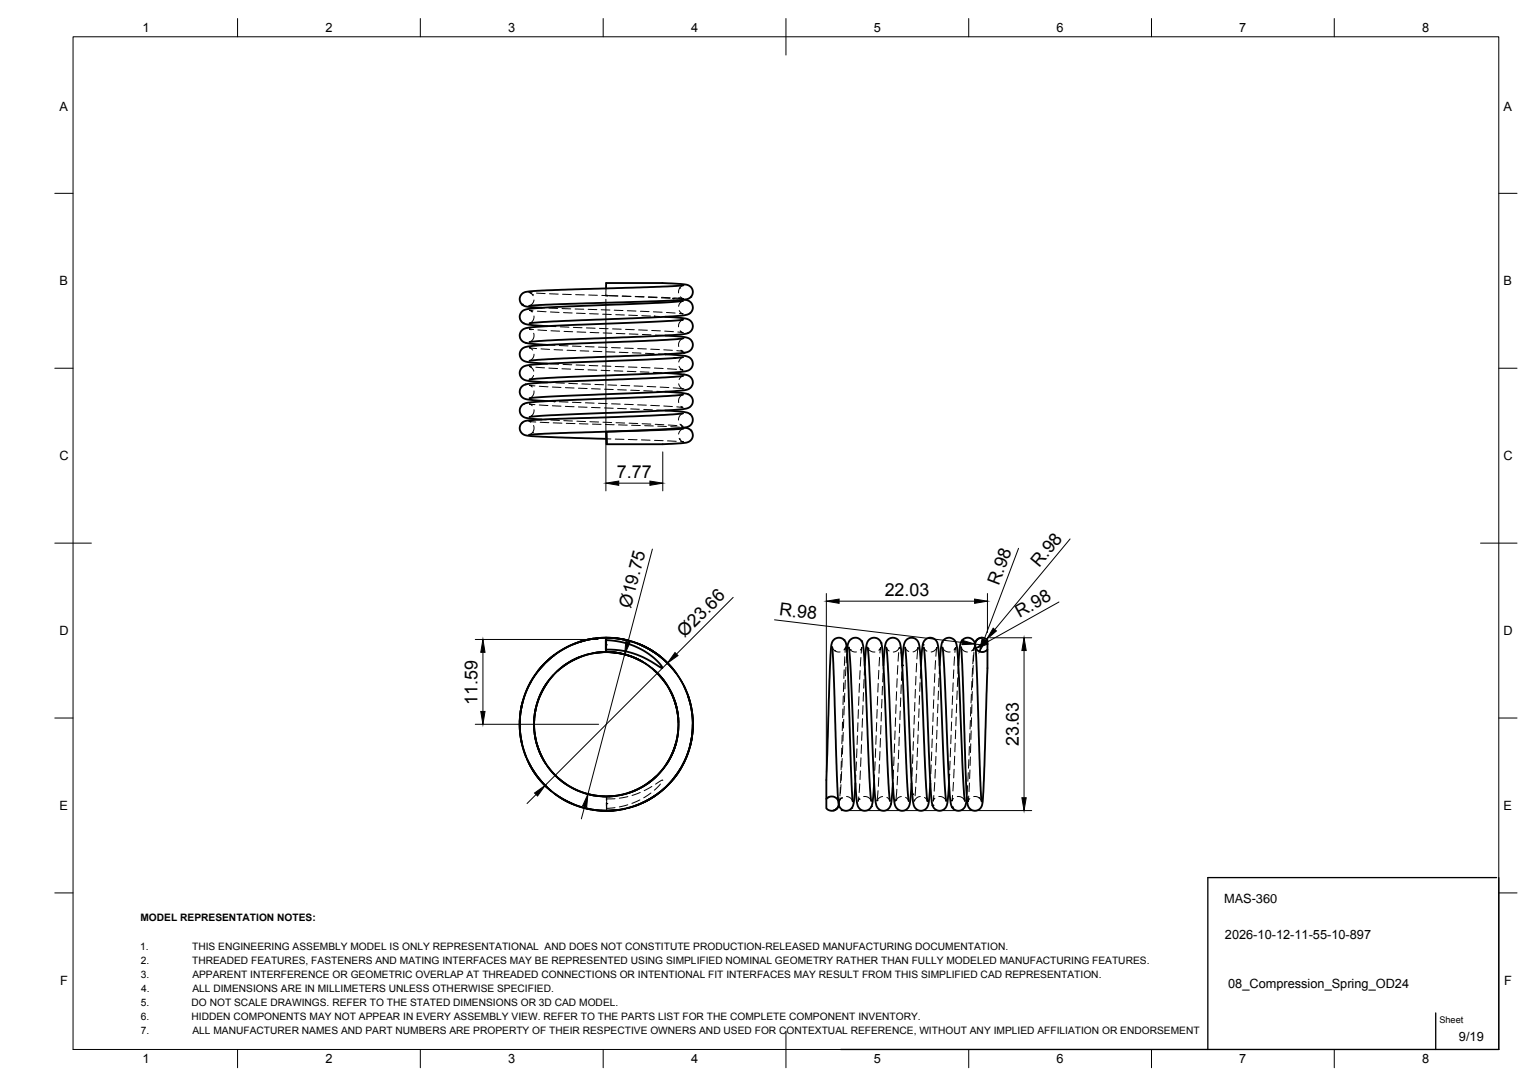
ISO-10303-21;
HEADER;
/* Generated by software containing ST-Developer
 * from STEP Tools, Inc. (www.steptools.com) 
 */

FILE_DESCRIPTION(
/* description */ (''),
/* implementation_level */ '2;1');

FILE_NAME(
/* name */ '08_Compression_Spring_OD24.step',
/* time_stamp */ '2026-11-04T18:53:29-08:00',
/* author */ (''),
/* organization */ (''),
/* preprocessor_version */ 'ST-DEVELOPER v20.2',
/* originating_system */ 'Autodesk Translation Framework v15.17.0.0',
/* authorisation */ '');

FILE_SCHEMA (('AUTOMOTIVE_DESIGN { 1 0 10303 214 3 1 1 }'));
ENDSEC;

DATA;
#10=MECHANICAL_DESIGN_GEOMETRIC_PRESENTATION_REPRESENTATION('',(#1334),#100031);
#1298=SHAPE_REPRESENTATION_RELATIONSHIP('SRR','None',#100108,#1316);
#1316=ADVANCED_BREP_SHAPE_REPRESENTATION('',(#1352),#100020);
#1334=STYLED_ITEM('',(#100203),#1352);
#1352=MANIFOLD_SOLID_BREP('Body1',#20124);
#1634=PLANE('',#22153);
#1635=PLANE('',#22154);
#1636=PLANE('',#22155);
#1637=PLANE('',#22156);
#1774=FACE_BOUND('',#7247,.T.);
#1775=FACE_BOUND('',#7248,.T.);
#3151=LINE('',#93226,#4438);
#3152=LINE('',#93320,#4439);
#4438=VECTOR('',#27336,10.);
#4439=VECTOR('',#27341,10.);
#6005=FACE_OUTER_BOUND('',#7242,.T.);
#6006=FACE_OUTER_BOUND('',#7243,.T.);
#6007=FACE_OUTER_BOUND('',#7244,.T.);
#6008=FACE_OUTER_BOUND('',#7245,.T.);
#6009=FACE_OUTER_BOUND('',#7246,.T.);
#6010=FACE_OUTER_BOUND('',#7249,.T.);
#7242=EDGE_LOOP('',(#18137,#18138));
#7243=EDGE_LOOP('',(#18139,#18140,#18141,#18142,#18143,#18144,#18145));
#7244=EDGE_LOOP('',(#18146,#18147));
#7245=EDGE_LOOP('',(#18148,#18149,#18150,#18151,#18152,#18153,#18154));
#7246=EDGE_LOOP('',(#18155,#18156,#18157,#18158,#18159,#18160,#18161,#18162));
#7247=EDGE_LOOP('',(#18163,#18164));
#7248=EDGE_LOOP('',(#18165,#18166));
#7249=EDGE_LOOP('',(#18167,#18168,#18169,#18170,#18171,#18172,#18173,#18174,
#18175,#18176));
#7985=B_SPLINE_CURVE_WITH_KNOTS('',3,(#93194,#93195,#93196,#93197,#93198,
#93199,#93200,#93201,#93202,#93203,#93204,#93205,#93206,#93207,#93208,#93209,
#93210,#93211,#93212,#93213,#93214,#93215,#93216,#93217,#93218,#93219,#93220,
#93221,#93222,#93223,#93224,#93225),.UNSPECIFIED.,.F.,.F.,(4,2,2,2,2,2,
2,2,2,2,2,2,2,2,2,4),(3.54152458065573E-10,0.288711445101139,0.523258332244725,
0.921227317049852,1.09267154481917,1.12602826877806,1.13805490776081,1.14561247672485,
1.15218349843735,1.15992334586198,1.17330081210199,1.20544465265463,1.30433060811633,
1.73541082798229,2.00533365271455,2.34908372554942),.UNSPECIFIED.);
#7986=B_SPLINE_CURVE_WITH_KNOTS('',3,(#93229,#93230,#93231,#93232,#93233,
#93234,#93235,#93236,#93237,#93238),.UNSPECIFIED.,.F.,.F.,(4,2,2,2,4),(-0.235035705616533,
-0.164045621201278,-0.0870897131881243,-0.0381417578315876,0.),
 .UNSPECIFIED.);
#7987=B_SPLINE_CURVE_WITH_KNOTS('',3,(#93240,#93241,#93242,#93243,#93244,
#93245,#93246,#93247,#93248,#93249),.UNSPECIFIED.,.F.,.F.,(4,2,2,2,4),(-0.0803122862957921,
-0.0602646333915054,-0.0402202940526313,-0.0201483463522527,-3.56243524540593E-5),
 .UNSPECIFIED.);
#7988=B_SPLINE_CURVE_WITH_KNOTS('',3,(#93251,#93252,#93253,#93254,#93255,
#93256),.UNSPECIFIED.,.F.,.F.,(4,2,4),(8.43662143615864E-5,0.00327116298064693,
0.00646179051431274),.UNSPECIFIED.);
#7989=B_SPLINE_CURVE_WITH_KNOTS('',3,(#93258,#93259,#93260,#93261,#93262,
#93263,#93264,#93265,#93266,#93267),.UNSPECIFIED.,.F.,.F.,(4,2,2,2,4),(-0.106351401183245,
-0.0798864576605021,-0.0531877160318232,-0.0265812067152108,-7.06104949174502E-6),
 .UNSPECIFIED.);
#7990=B_SPLINE_CURVE_WITH_KNOTS('',3,(#93269,#93270,#93271,#93272,#93273,
#93274,#93275,#93276,#93277,#93278),.UNSPECIFIED.,.F.,.F.,(4,2,2,2,4),(-0.0971883190541716,
-0.0727561460747867,-0.048468056376207,-0.0242270507757942,0.),
 .UNSPECIFIED.);
#7991=B_SPLINE_CURVE_WITH_KNOTS('',3,(#93279,#93280,#93281,#93282,#93283,
#93284),.UNSPECIFIED.,.F.,.F.,(4,2,4),(-0.0301723368590298,-0.0150922159606526,
-2.55953913249195E-6),.UNSPECIFIED.);
#7992=B_SPLINE_CURVE_WITH_KNOTS('',3,(#93288,#93289,#93290,#93291,#93292,
#93293,#93294,#93295,#93296,#93297,#93298,#93299,#93300,#93301,#93302,#93303,
#93304,#93305,#93306,#93307,#93308,#93309,#93310,#93311,#93312,#93313,#93314,
#93315,#93316,#93317,#93318,#93319),.UNSPECIFIED.,.F.,.F.,(4,2,2,2,2,2,
2,2,2,2,2,2,2,2,2,4),(-2.01212438752124,-1.76578196828659,-1.5647664663706,
-1.20118246901991,-1.06053517315717,-1.02977885200715,-1.0193276272259,
-1.01279623524482,-1.00715009449403,-1.00055979488344,-0.989257775261865,
-0.96242213266161,-0.881471927659453,-0.518895860123459,-0.290806811506921,
-8.2501916409683E-10),.UNSPECIFIED.);
#7993=B_SPLINE_CURVE_WITH_KNOTS('',3,(#93323,#93324,#93325,#93326,#93327,
#93328,#93329,#93330,#93331,#93332),.UNSPECIFIED.,.F.,.F.,(4,2,2,2,4),(-0.189468447311924,
-0.155678960910493,-0.111541963335214,-0.0470106922386932,-7.10058815808075E-6),
 .UNSPECIFIED.);
#7994=B_SPLINE_CURVE_WITH_KNOTS('',3,(#93334,#93335,#93336,#93337,#93338,
#93339,#93340,#93341,#93342,#93343),.UNSPECIFIED.,.F.,.F.,(4,2,2,2,4),(-0.0812741980146226,
-0.061010630542918,-0.0406258560977219,-0.0203042042142377,0.),
 .UNSPECIFIED.);
#7995=B_SPLINE_CURVE_WITH_KNOTS('',3,(#93345,#93346,#93347,#93348,#93349,
#93350),.UNSPECIFIED.,.F.,.F.,(4,2,4),(-0.0064959341341575,-0.00329347810601311,
-8.81436577924804E-5),.UNSPECIFIED.);
#7996=B_SPLINE_CURVE_WITH_KNOTS('',3,(#93352,#93353,#93354,#93355,#93356,
#93357),.UNSPECIFIED.,.F.,.F.,(4,2,4),(-0.00936112110047215,-0.00472017132367055,
-6.30707363171211E-5),.UNSPECIFIED.);
#7997=B_SPLINE_CURVE_WITH_KNOTS('',3,(#93359,#93360,#93361,#93362,#93363,
#93364,#93365,#93366,#93367,#93368,#93369,#93370,#93371,#93372,#93373,#93374),
 .UNSPECIFIED.,.F.,.F.,(4,2,2,2,2,2,2,4),(-0.201490383661384,-0.178130230033713,
-0.154775766161226,-0.145700922114215,-0.102563961887103,-0.0587557032775208,
-0.029368346867021,-7.06104927835685E-6),.UNSPECIFIED.);
#7998=B_SPLINE_CURVE_WITH_KNOTS('',3,(#93375,#93376,#93377,#93378,#93379,
#93380),.UNSPECIFIED.,.F.,.F.,(4,2,4),(-0.0308102197342027,-0.0154008404140284,
0.),.UNSPECIFIED.);
#7999=B_SPLINE_CURVE_WITH_KNOTS('',3,(#94481,#94482,#94483,#94484,#94485,
#94486,#94487,#94488,#94489,#94490,#94491,#94492,#94493,#94494,#94495,#94496,
#94497,#94498,#94499,#94500,#94501,#94502,#94503,#94504,#94505,#94506,#94507,
#94508,#94509,#94510,#94511,#94512,#94513,#94514,#94515,#94516,#94517,#94518,
#94519,#94520,#94521,#94522,#94523,#94524,#94525,#94526,#94527,#94528,#94529,
#94530,#94531,#94532,#94533,#94534,#94535,#94536,#94537,#94538,#94539,#94540,
#94541,#94542,#94543,#94544,#94545,#94546,#94547,#94548,#94549,#94550,#94551,
#94552,#94553,#94554,#94555,#94556,#94557,#94558,#94559,#94560,#94561,#94562,
#94563,#94564,#94565,#94566,#94567,#94568,#94569,#94570,#94571,#94572,#94573,
#94574,#94575,#94576,#94577,#94578,#94579,#94580,#94581,#94582,#94583,#94584,
#94585,#94586,#94587,#94588,#94589,#94590,#94591,#94592,#94593,#94594,#94595,
#94596,#94597,#94598,#94599,#94600,#94601,#94602,#94603,#94604,#94605,#94606,
#94607,#94608,#94609,#94610,#94611,#94612,#94613,#94614,#94615,#94616,#94617,
#94618,#94619,#94620,#94621,#94622,#94623,#94624,#94625,#94626,#94627,#94628,
#94629,#94630,#94631,#94632,#94633,#94634,#94635,#94636,#94637,#94638,#94639,
#94640,#94641,#94642,#94643,#94644,#94645,#94646,#94647,#94648,#94649,#94650,
#94651,#94652,#94653,#94654,#94655,#94656,#94657,#94658,#94659,#94660,#94661,
#94662,#94663,#94664,#94665,#94666,#94667,#94668,#94669,#94670,#94671,#94672,
#94673,#94674,#94675,#94676,#94677,#94678,#94679,#94680,#94681,#94682,#94683,
#94684,#94685,#94686,#94687,#94688,#94689,#94690,#94691,#94692,#94693,#94694,
#94695,#94696,#94697,#94698,#94699,#94700,#94701,#94702,#94703,#94704,#94705,
#94706,#94707,#94708,#94709,#94710,#94711,#94712,#94713,#94714,#94715,#94716,
#94717,#94718,#94719,#94720,#94721,#94722,#94723,#94724,#94725,#94726,#94727,
#94728,#94729,#94730,#94731,#94732,#94733,#94734,#94735,#94736,#94737,#94738,
#94739,#94740,#94741,#94742,#94743,#94744,#94745,#94746,#94747,#94748,#94749,
#94750,#94751,#94752,#94753,#94754,#94755,#94756,#94757,#94758,#94759,#94760,
#94761,#94762,#94763,#94764,#94765,#94766,#94767,#94768,#94769,#94770,#94771,
#94772,#94773,#94774,#94775,#94776,#94777,#94778,#94779,#94780,#94781,#94782,
#94783,#94784,#94785,#94786,#94787,#94788,#94789,#94790,#94791,#94792,#94793,
#94794,#94795,#94796,#94797,#94798,#94799,#94800,#94801,#94802,#94803,#94804,
#94805,#94806,#94807,#94808,#94809,#94810,#94811,#94812,#94813,#94814,#94815,
#94816,#94817,#94818,#94819,#94820,#94821,#94822,#94823,#94824,#94825,#94826,
#94827,#94828,#94829,#94830,#94831,#94832,#94833,#94834,#94835,#94836,#94837,
#94838,#94839,#94840,#94841,#94842,#94843,#94844,#94845,#94846,#94847,#94848,
#94849,#94850,#94851,#94852,#94853,#94854,#94855,#94856,#94857,#94858,#94859,
#94860,#94861,#94862,#94863,#94864,#94865,#94866,#94867,#94868,#94869,#94870,
#94871,#94872,#94873,#94874,#94875,#94876,#94877,#94878,#94879,#94880,#94881,
#94882,#94883,#94884,#94885,#94886,#94887,#94888,#94889,#94890,#94891,#94892,
#94893,#94894,#94895,#94896,#94897,#94898,#94899,#94900,#94901,#94902,#94903,
#94904,#94905,#94906,#94907,#94908,#94909,#94910,#94911,#94912,#94913,#94914,
#94915,#94916,#94917,#94918,#94919,#94920,#94921,#94922,#94923,#94924,#94925,
#94926,#94927,#94928,#94929,#94930,#94931,#94932,#94933,#94934,#94935,#94936,
#94937,#94938,#94939,#94940,#94941,#94942,#94943,#94944,#94945,#94946,#94947,
#94948,#94949,#94950,#94951,#94952,#94953,#94954,#94955,#94956,#94957,#94958,
#94959,#94960,#94961,#94962,#94963,#94964,#94965,#94966,#94967,#94968,#94969,
#94970,#94971,#94972,#94973,#94974,#94975,#94976,#94977,#94978,#94979,#94980,
#94981,#94982,#94983,#94984,#94985,#94986,#94987,#94988,#94989,#94990,#94991,
#94992,#94993,#94994,#94995,#94996,#94997,#94998,#94999,#95000,#95001,#95002,
#95003,#95004,#95005,#95006,#95007,#95008,#95009,#95010,#95011,#95012,#95013,
#95014,#95015,#95016,#95017,#95018,#95019,#95020,#95021,#95022,#95023,#95024,
#95025,#95026,#95027,#95028,#95029,#95030,#95031,#95032,#95033,#95034,#95035,
#95036,#95037,#95038,#95039,#95040,#95041,#95042,#95043,#95044,#95045,#95046,
#95047,#95048,#95049,#95050,#95051,#95052,#95053,#95054,#95055,#95056,#95057,
#95058,#95059,#95060,#95061,#95062,#95063,#95064,#95065,#95066,#95067,#95068,
#95069,#95070,#95071,#95072,#95073,#95074,#95075,#95076,#95077,#95078,#95079,
#95080,#95081,#95082,#95083,#95084,#95085,#95086,#95087,#95088,#95089,#95090,
#95091,#95092,#95093,#95094,#95095,#95096,#95097,#95098,#95099,#95100,#95101,
#95102,#95103,#95104,#95105,#95106,#95107,#95108,#95109,#95110,#95111,#95112,
#95113,#95114,#95115,#95116,#95117,#95118,#95119,#95120,#95121,#95122,#95123,
#95124,#95125,#95126,#95127,#95128,#95129,#95130,#95131,#95132,#95133,#95134,
#95135,#95136,#95137,#95138,#95139,#95140,#95141,#95142,#95143,#95144,#95145,
#95146,#95147,#95148,#95149,#95150,#95151,#95152,#95153,#95154,#95155,#95156,
#95157,#95158,#95159,#95160,#95161,#95162,#95163,#95164,#95165,#95166,#95167,
#95168,#95169,#95170,#95171,#95172,#95173,#95174,#95175,#95176,#95177,#95178,
#95179,#95180,#95181,#95182,#95183,#95184,#95185,#95186,#95187,#95188,#95189,
#95190,#95191,#95192,#95193,#95194,#95195,#95196,#95197,#95198,#95199,#95200,
#95201,#95202,#95203,#95204,#95205,#95206,#95207,#95208,#95209,#95210,#95211,
#95212,#95213,#95214,#95215,#95216,#95217,#95218,#95219,#95220,#95221,#95222,
#95223,#95224,#95225,#95226,#95227,#95228,#95229,#95230,#95231,#95232,#95233,
#95234,#95235,#95236,#95237,#95238,#95239,#95240,#95241,#95242,#95243,#95244,
#95245,#95246,#95247,#95248,#95249,#95250,#95251,#95252,#95253,#95254,#95255,
#95256,#95257,#95258,#95259,#95260,#95261,#95262,#95263,#95264,#95265,#95266,
#95267,#95268,#95269,#95270,#95271,#95272,#95273,#95274,#95275,#95276,#95277,
#95278,#95279,#95280,#95281,#95282,#95283,#95284,#95285,#95286,#95287,#95288,
#95289,#95290,#95291,#95292,#95293,#95294,#95295,#95296,#95297,#95298,#95299,
#95300,#95301,#95302,#95303,#95304,#95305,#95306,#95307,#95308,#95309,#95310,
#95311,#95312,#95313,#95314,#95315,#95316,#95317,#95318,#95319,#95320,#95321,
#95322,#95323,#95324,#95325,#95326,#95327,#95328,#95329,#95330,#95331,#95332,
#95333,#95334,#95335,#95336,#95337,#95338,#95339,#95340,#95341,#95342,#95343,
#95344,#95345,#95346,#95347,#95348,#95349,#95350,#95351,#95352,#95353,#95354,
#95355,#95356,#95357,#95358,#95359,#95360,#95361,#95362,#95363,#95364,#95365,
#95366,#95367,#95368,#95369,#95370,#95371,#95372,#95373,#95374,#95375,#95376,
#95377,#95378,#95379,#95380,#95381,#95382,#95383,#95384,#95385,#95386,#95387,
#95388,#95389,#95390,#95391,#95392,#95393,#95394,#95395,#95396,#95397,#95398,
#95399,#95400,#95401,#95402,#95403,#95404,#95405,#95406,#95407,#95408,#95409,
#95410,#95411,#95412,#95413,#95414,#95415,#95416,#95417,#95418,#95419,#95420,
#95421,#95422,#95423,#95424,#95425,#95426,#95427,#95428,#95429,#95430,#95431,
#95432,#95433,#95434,#95435,#95436,#95437,#95438,#95439,#95440,#95441,#95442,
#95443,#95444,#95445,#95446,#95447,#95448,#95449,#95450,#95451,#95452,#95453,
#95454,#95455,#95456,#95457,#95458,#95459,#95460,#95461,#95462,#95463,#95464,
#95465,#95466,#95467,#95468,#95469,#95470,#95471,#95472,#95473,#95474,#95475,
#95476,#95477,#95478,#95479,#95480,#95481,#95482,#95483,#95484,#95485,#95486,
#95487,#95488,#95489,#95490,#95491,#95492,#95493,#95494,#95495,#95496,#95497,
#95498,#95499,#95500,#95501,#95502,#95503,#95504,#95505,#95506,#95507,#95508,
#95509,#95510,#95511,#95512,#95513,#95514,#95515,#95516,#95517,#95518,#95519,
#95520,#95521,#95522,#95523,#95524,#95525,#95526,#95527,#95528,#95529,#95530,
#95531,#95532,#95533,#95534,#95535,#95536,#95537,#95538,#95539,#95540,#95541,
#95542,#95543,#95544,#95545,#95546,#95547,#95548,#95549,#95550,#95551,#95552,
#95553,#95554,#95555,#95556,#95557,#95558,#95559,#95560,#95561,#95562,#95563,
#95564,#95565,#95566,#95567,#95568,#95569,#95570,#95571,#95572,#95573,#95574,
#95575,#95576,#95577,#95578,#95579,#95580,#95581,#95582,#95583,#95584,#95585,
#95586,#95587,#95588,#95589,#95590,#95591,#95592,#95593,#95594,#95595,#95596,
#95597,#95598,#95599,#95600,#95601,#95602,#95603,#95604,#95605,#95606,#95607,
#95608,#95609,#95610,#95611,#95612,#95613,#95614,#95615,#95616,#95617,#95618,
#95619,#95620,#95621,#95622,#95623,#95624,#95625,#95626,#95627,#95628,#95629,
#95630,#95631,#95632,#95633,#95634,#95635,#95636,#95637,#95638,#95639,#95640,
#95641,#95642,#95643,#95644,#95645,#95646,#95647,#95648,#95649,#95650,#95651,
#95652,#95653,#95654,#95655,#95656,#95657,#95658,#95659,#95660,#95661,#95662,
#95663,#95664,#95665,#95666),.UNSPECIFIED.,.F.,.F.,(4,3,3,3,3,3,3,3,3,3,
3,3,3,3,3,3,3,3,3,3,3,3,3,3,3,3,3,3,3,3,3,3,3,3,3,3,3,3,3,3,3,3,3,3,3,3,
3,3,3,3,3,3,3,3,3,3,3,3,3,3,3,3,3,3,3,3,3,3,3,3,3,3,3,3,3,3,3,3,3,3,3,3,
3,3,3,3,3,3,3,3,3,3,3,3,3,3,3,3,3,3,3,3,3,3,3,3,3,3,3,3,3,3,3,3,3,3,3,3,
3,3,3,3,3,3,3,3,3,3,3,3,3,3,3,3,3,3,3,3,3,3,3,3,3,3,3,3,3,3,3,3,3,3,3,3,
3,3,3,3,3,3,3,3,3,3,3,3,3,3,3,3,3,3,3,3,3,3,3,3,3,3,3,3,3,3,3,3,3,3,3,3,
3,3,3,3,3,3,3,3,3,3,3,3,3,3,3,3,3,3,3,3,3,3,3,3,3,3,3,3,3,3,3,3,3,3,3,3,
3,3,3,3,3,3,3,3,3,3,3,3,3,3,3,3,3,3,3,3,3,3,3,3,3,3,3,3,3,3,3,3,3,3,3,3,
3,3,3,3,3,3,3,3,3,3,3,3,3,3,3,3,3,3,3,3,3,3,3,3,3,3,3,3,3,3,3,3,3,3,3,3,
3,3,3,3,3,3,3,3,3,3,3,3,3,3,3,3,3,3,3,3,3,3,3,3,3,3,3,3,3,3,3,3,3,3,3,3,
3,3,3,3,3,3,3,3,3,3,3,3,3,3,3,3,3,3,3,3,3,3,3,3,3,3,3,3,3,3,3,3,3,3,3,3,
3,3,3,3,3,3,3,3,3,3,3,3,3,3,3,3,3,3,3,3,3,3,3,3,3,4),(-1.,-0.991071428571429,
-0.991071389429951,-0.982142857142857,-0.982142822785736,-0.973214285714286,
-0.973214273423607,-0.964285719587971,-0.964285714285714,-0.955357154845019,
-0.955357142857143,-0.946428582987328,-0.946428571428571,-0.937500007454815,
-0.9375,-0.928571435886753,-0.928571428571429,-0.919642857142857,-0.910714285714286,
-0.910714278487105,-0.903444178215078,-0.901785714285714,-0.8962006132777,
-0.892857142857143,-0.89285703296426,-0.888392835478123,-0.883928637991986,
-0.883928571428571,-0.880170831457046,-0.876470542060389,-0.875,-0.874999572863337,
-0.871518316066235,-0.868090467473807,-0.866071717001134,-0.866071428571429,
-0.863200415042696,-0.860343926901775,-0.857531528156535,-0.857143004738549,
-0.857142857142857,-0.854312859661374,-0.852678571428572,-0.850614304741742,
-0.848565036595157,-0.848214285714286,-0.846890953347238,-0.845982142857143,
-0.845238193734111,-0.843631148930307,-0.842633928571428,-0.840878948010448,
-0.839285714285714,-0.836887599372128,-0.834821428571428,-0.833333913300317,
-0.832589285714286,-0.831300035123872,-0.830357142857143,-0.828357848817079,
-0.826356039658343,-0.825892857142857,-0.823988309272079,-0.822088982612407,
-0.821428571428571,-0.821428367725019,-0.819505414596167,-0.8175860310261,
-0.816964285714285,-0.814956467981351,-0.812947024322632,-0.8125,-0.810292489456701,
-0.809523200608117,-0.807330760640928,-0.805140498994953,-0.803571428571428,
-0.801586644036287,-0.798469918994543,-0.795270754281138,-0.794642857142857,
-0.793650917020491,-0.790320032619685,-0.787044258957954,-0.785714306584564,
-0.785714285714286,-0.783413209641271,-0.781107750138836,-0.780867818478783,
-0.778951670344505,-0.777780830372113,-0.777338671144154,-0.775574097476839,
-0.773809523809524,-0.770273481108357,-0.769838188635457,-0.7689930392807,
-0.767153440241231,-0.765448900592731,-0.763199787229666,-0.761904871965663,
-0.761904761904762,-0.760089872236183,-0.758275764324489,-0.757077354179359,
-0.755244041175192,-0.75396837627968,-0.753538677089679,-0.751655164247817,
-0.75,-0.748015716198947,-0.747767857142857,-0.746029646317197,-0.743550537444313,
-0.741071428571428,-0.739773961496372,-0.738839285714285,-0.738095686705119,
-0.736694105353861,-0.735491071428571,-0.733673411592545,-0.732142857142857,
-0.730204502448423,-0.728272184556273,-0.727678571428572,-0.72619055472343,
-0.725446428571429,-0.724300149594122,-0.723214285714286,-0.721270255978889,
-0.719314481159982,-0.71875,-0.717013707960798,-0.715279745045851,-0.714285714285714,
-0.714284646236362,-0.712090385576223,-0.709893252584267,-0.708333333333333,
-0.706097031223049,-0.703882549937917,-0.702381642308063,-0.702380952380952,
-0.699974534521517,-0.697519859321161,-0.695069959055868,-0.692693401084694,
-0.69047619047619,-0.690474133472452,-0.688920512294885,-0.687369792937533,
-0.686507936507937,-0.684145833909582,-0.682539682539683,-0.680167707232127,
-0.678571620568218,-0.67621012605145,-0.674603174603175,-0.67261819681719,
-0.66998184520372,-0.667337275851678,-0.666667233377128,-0.666666666666667,
-0.663645875002391,-0.660576136857663,-0.658730158730159,-0.658729978699635,
-0.655155726859902,-0.651537345370322,-0.650793955011456,-0.650793650793651,
-0.64648921283136,-0.642857384281078,-0.642857142857143,-0.637654450300913,
-0.634921030719177,-0.634920634920635,-0.627923928049837,-0.626984354640624,
-0.626984126984127,-0.622156503929432,-0.619047619047619,-0.619047289450574,
-0.613700647719127,-0.608263744404841,-0.607142857142857,-0.607142848983513,
-0.599710180861582,-0.595238127445014,-0.595238095238095,-0.586752880028379,
-0.583333340923382,-0.583333333333333,-0.573056502544092,-0.571428587791853,
-0.571428571428571,-0.559523813525363,-0.55952380952381,-0.547619052167738,
-0.547619047619048,-0.535714288277056,-0.535714285714286,-0.523809523809524,
-0.515873015873016,-0.507936512898811,-0.507936507936508,-0.5,-0.499999995871733,
-0.492063492063492,-0.492063478197101,-0.484467253634067,-0.481481481481481,
-0.481481440717216,-0.476190476190476,-0.476190396250867,-0.471892865305429,
-0.46825409755741,-0.468253968253968,-0.464547293860793,-0.460878327493757,
-0.46031746031746,-0.460317416879269,-0.457285356553107,-0.45429626344784,
-0.452381592760412,-0.452380952380952,-0.44969797322538,-0.447000164675377,
-0.444320561617439,-0.441723294699108,-0.44047619047619,-0.440476006991694,
-0.438220240631386,-0.43596270509345,-0.43452380952381,-0.432270078724781,
-0.430045371855419,-0.428571428571429,-0.428568980975705,-0.426647084103455,
-0.424633391022285,-0.422619697941116,-0.422619047619048,-0.420858569468115,
-0.419096741455247,-0.417339083079523,-0.416666903236966,-0.416666666666667,
-0.414332050427676,-0.411997434188685,-0.409856872686492,-0.40771882742928,
-0.405591465610837,-0.404761904761905,-0.404761616116348,-0.403144853246966,
-0.401526682096213,-0.400793650793651,-0.398777598024052,-0.396825396825397,
-0.395471659185257,-0.39484126984127,-0.393176998777955,-0.392858194162737,
-0.39186507936508,-0.390357253125332,-0.388888888888889,-0.387207358382915,
-0.386904761904762,-0.385110812996099,-0.383928571428572,-0.382587499125909,
-0.381247225112031,-0.380952457568705,-0.380952380952381,-0.378563261893649,
-0.376224906962247,-0.375661375661376,-0.373920443009037,-0.372193839494745,
-0.37097458200055,-0.369358460438232,-0.3690480190967,-0.368026973539958,
-0.365516896588505,-0.365079365079365,-0.363326640224003,-0.363095238095238,
-0.361512105321307,-0.35992885568622,-0.358346761150496,-0.357145070531906,
-0.357142857142857,-0.355546286153388,-0.35394320567017,-0.353174603174603,
-0.351902018190071,-0.351190476190476,-0.349634484581003,-0.349206349206349,
-0.347221939748124,-0.3452375302899,-0.34325368577987,-0.341269841269841,
-0.339198036849855,-0.337301587301587,-0.33531747481785,-0.333333362334113,
-0.333333333333333,-0.331306663695514,-0.329285252778724,-0.327382478472304,
-0.327380952380952,-0.325604664984563,-0.323826219469051,-0.322049559443716,
-0.321428739717564,-0.321428571428571,-0.318170228212089,-0.314792094541723,
-0.311349092498602,-0.309524714317972,-0.30952380952381,-0.306242345183409,
-0.302855094187904,-0.299476694932263,-0.297619047619048,-0.297618383218759,
-0.293739893156044,-0.28972711509084,-0.285714337025636,-0.285714285714286,
-0.280392556199838,-0.274939048722368,-0.273809527057199,-0.273809523809524,
-0.267759242157021,-0.261904904421664,-0.261904761904762,-0.255743652740556,
-0.250000588693953,-0.25,-0.243006450702321,-0.238095981836014,-0.236300908282312,
-0.23015906433374,-0.23015873015873,-0.226125727537763,-0.222222574129115,
-0.222222222222222,-0.218754557253951,-0.215242389059935,-0.214286338712583,
-0.214285714285714,-0.209074191895231,-0.203699859680209,-0.2023814347069,
-0.202380952380952,-0.195767114280798,-0.190476314984547,-0.19047619047619,
-0.182700873239942,-0.178571466870454,-0.178571428571429,-0.166666671143928,
-0.166666666666667,-0.154761914101637,-0.154761904761905,-0.142857151151493,
-0.142857142857143,-0.133928577582602,-0.133928571428571,-0.125000003845394,
-0.125,-0.116071430990516,-0.116071428571429,-0.107142857142857,-0.0982142857142857,
-0.0892857142857143,-0.0803571428571428,-0.0714285714285714,-0.0714285693344336,
-0.0625,-0.0624999960539666,-0.0535714285714286,-0.0535714237366097,-0.0446428571428571,
-0.0446428521159013,-0.0357142857142857,-0.0267857244811938,-0.0267857142857143,
-0.0178571653672693,-0.0178571428571429,-0.00892859399562328,-0.00892857142857143,
0.),.UNSPECIFIED.);
#8000=B_SPLINE_CURVE_WITH_KNOTS('',3,(#95667,#95668,#95669,#95670,#95671,
#95672,#95673,#95674,#95675,#95676,#95677,#95678,#95679,#95680,#95681,#95682,
#95683,#95684,#95685,#95686,#95687,#95688,#95689,#95690,#95691,#95692,#95693,
#95694,#95695,#95696,#95697,#95698,#95699,#95700,#95701,#95702,#95703,#95704,
#95705,#95706,#95707,#95708,#95709,#95710,#95711,#95712,#95713,#95714,#95715,
#95716,#95717,#95718,#95719,#95720,#95721,#95722,#95723,#95724,#95725,#95726,
#95727,#95728,#95729,#95730,#95731,#95732,#95733,#95734,#95735,#95736,#95737,
#95738,#95739,#95740,#95741,#95742,#95743,#95744,#95745,#95746,#95747,#95748,
#95749,#95750,#95751,#95752,#95753,#95754,#95755,#95756,#95757,#95758,#95759,
#95760,#95761,#95762,#95763,#95764,#95765,#95766,#95767,#95768,#95769,#95770,
#95771,#95772,#95773,#95774,#95775,#95776,#95777,#95778,#95779,#95780,#95781,
#95782,#95783,#95784,#95785,#95786,#95787,#95788,#95789,#95790,#95791,#95792,
#95793,#95794,#95795,#95796,#95797,#95798,#95799,#95800,#95801,#95802,#95803,
#95804,#95805,#95806,#95807,#95808,#95809,#95810,#95811,#95812,#95813,#95814,
#95815,#95816,#95817,#95818,#95819,#95820,#95821,#95822,#95823,#95824,#95825,
#95826,#95827,#95828,#95829,#95830,#95831,#95832,#95833,#95834,#95835,#95836,
#95837,#95838,#95839,#95840,#95841,#95842,#95843,#95844,#95845,#95846,#95847,
#95848,#95849,#95850,#95851,#95852,#95853,#95854,#95855,#95856,#95857,#95858,
#95859,#95860,#95861,#95862,#95863,#95864,#95865,#95866,#95867,#95868,#95869,
#95870,#95871,#95872,#95873,#95874,#95875,#95876,#95877,#95878,#95879,#95880,
#95881,#95882,#95883,#95884,#95885,#95886,#95887,#95888,#95889,#95890,#95891,
#95892,#95893,#95894,#95895,#95896,#95897,#95898,#95899,#95900,#95901,#95902,
#95903,#95904,#95905,#95906,#95907,#95908,#95909,#95910,#95911,#95912,#95913,
#95914,#95915,#95916,#95917,#95918,#95919,#95920,#95921,#95922,#95923,#95924,
#95925,#95926,#95927,#95928,#95929,#95930,#95931,#95932,#95933,#95934,#95935,
#95936,#95937,#95938,#95939,#95940,#95941,#95942,#95943,#95944,#95945,#95946,
#95947,#95948,#95949,#95950,#95951,#95952,#95953,#95954,#95955,#95956,#95957,
#95958,#95959,#95960,#95961,#95962,#95963,#95964,#95965,#95966,#95967,#95968,
#95969,#95970,#95971,#95972,#95973,#95974,#95975,#95976,#95977,#95978,#95979,
#95980,#95981,#95982,#95983,#95984,#95985,#95986,#95987,#95988,#95989,#95990,
#95991,#95992,#95993,#95994,#95995,#95996,#95997,#95998,#95999,#96000,#96001,
#96002,#96003,#96004,#96005,#96006,#96007,#96008,#96009,#96010,#96011,#96012,
#96013,#96014,#96015,#96016,#96017,#96018,#96019,#96020,#96021,#96022,#96023,
#96024,#96025,#96026,#96027,#96028,#96029,#96030,#96031,#96032,#96033,#96034,
#96035,#96036,#96037,#96038,#96039,#96040,#96041,#96042,#96043,#96044,#96045,
#96046,#96047,#96048,#96049,#96050,#96051,#96052,#96053,#96054,#96055,#96056,
#96057,#96058,#96059,#96060,#96061,#96062,#96063,#96064,#96065,#96066,#96067,
#96068,#96069,#96070,#96071,#96072,#96073,#96074,#96075,#96076,#96077,#96078,
#96079,#96080,#96081,#96082,#96083,#96084,#96085,#96086,#96087,#96088,#96089,
#96090,#96091,#96092,#96093,#96094,#96095,#96096,#96097,#96098,#96099,#96100,
#96101,#96102,#96103,#96104,#96105,#96106,#96107,#96108,#96109,#96110,#96111,
#96112,#96113,#96114,#96115,#96116,#96117,#96118,#96119,#96120,#96121,#96122,
#96123,#96124,#96125,#96126,#96127,#96128,#96129,#96130,#96131,#96132,#96133,
#96134,#96135,#96136,#96137,#96138,#96139,#96140,#96141,#96142,#96143,#96144,
#96145,#96146,#96147,#96148,#96149,#96150,#96151,#96152,#96153,#96154,#96155,
#96156,#96157,#96158,#96159,#96160,#96161,#96162,#96163,#96164,#96165,#96166,
#96167,#96168,#96169,#96170,#96171,#96172,#96173,#96174,#96175,#96176,#96177,
#96178,#96179,#96180,#96181,#96182,#96183,#96184,#96185,#96186,#96187,#96188,
#96189,#96190,#96191,#96192,#96193,#96194,#96195,#96196,#96197,#96198,#96199,
#96200,#96201,#96202,#96203,#96204,#96205,#96206,#96207,#96208,#96209,#96210,
#96211,#96212,#96213,#96214,#96215,#96216,#96217,#96218,#96219,#96220,#96221,
#96222,#96223,#96224,#96225,#96226,#96227,#96228,#96229,#96230,#96231,#96232,
#96233,#96234,#96235,#96236,#96237,#96238,#96239,#96240,#96241,#96242,#96243,
#96244,#96245,#96246,#96247,#96248,#96249,#96250,#96251,#96252,#96253,#96254,
#96255,#96256,#96257,#96258,#96259,#96260,#96261,#96262,#96263,#96264,#96265,
#96266,#96267,#96268,#96269,#96270,#96271,#96272,#96273,#96274,#96275,#96276,
#96277,#96278,#96279,#96280,#96281,#96282,#96283,#96284,#96285,#96286,#96287,
#96288,#96289,#96290,#96291,#96292,#96293,#96294,#96295,#96296,#96297,#96298,
#96299,#96300,#96301,#96302,#96303,#96304,#96305,#96306,#96307,#96308,#96309,
#96310,#96311,#96312,#96313,#96314,#96315,#96316,#96317,#96318,#96319,#96320,
#96321,#96322,#96323,#96324,#96325,#96326,#96327,#96328,#96329,#96330,#96331,
#96332,#96333,#96334,#96335,#96336,#96337,#96338,#96339,#96340,#96341,#96342,
#96343,#96344,#96345,#96346,#96347,#96348,#96349,#96350,#96351,#96352,#96353,
#96354,#96355,#96356,#96357,#96358,#96359,#96360,#96361,#96362,#96363,#96364,
#96365,#96366,#96367,#96368,#96369,#96370,#96371,#96372,#96373,#96374,#96375,
#96376,#96377,#96378,#96379,#96380,#96381,#96382,#96383,#96384,#96385,#96386,
#96387,#96388,#96389,#96390,#96391,#96392,#96393,#96394,#96395,#96396,#96397,
#96398,#96399,#96400,#96401,#96402,#96403,#96404,#96405,#96406,#96407,#96408,
#96409,#96410,#96411,#96412,#96413,#96414,#96415,#96416,#96417,#96418,#96419,
#96420,#96421,#96422,#96423,#96424,#96425,#96426,#96427,#96428,#96429,#96430,
#96431,#96432,#96433,#96434,#96435,#96436,#96437,#96438,#96439,#96440,#96441,
#96442,#96443,#96444,#96445,#96446,#96447,#96448,#96449,#96450,#96451,#96452,
#96453,#96454,#96455,#96456,#96457,#96458,#96459,#96460,#96461,#96462,#96463,
#96464,#96465,#96466,#96467,#96468,#96469,#96470,#96471,#96472,#96473,#96474,
#96475,#96476,#96477,#96478,#96479,#96480,#96481,#96482,#96483,#96484,#96485,
#96486,#96487,#96488,#96489,#96490,#96491,#96492,#96493,#96494,#96495,#96496,
#96497,#96498,#96499,#96500,#96501,#96502,#96503,#96504,#96505,#96506,#96507,
#96508,#96509,#96510,#96511,#96512,#96513,#96514,#96515,#96516,#96517,#96518,
#96519,#96520,#96521,#96522,#96523,#96524,#96525,#96526,#96527,#96528,#96529,
#96530,#96531,#96532,#96533,#96534,#96535,#96536,#96537,#96538,#96539,#96540,
#96541,#96542,#96543,#96544,#96545,#96546,#96547,#96548,#96549,#96550,#96551,
#96552,#96553,#96554,#96555,#96556,#96557,#96558,#96559,#96560,#96561,#96562,
#96563,#96564,#96565,#96566,#96567,#96568,#96569,#96570,#96571,#96572,#96573,
#96574,#96575,#96576,#96577,#96578,#96579,#96580,#96581,#96582,#96583,#96584,
#96585,#96586,#96587,#96588,#96589,#96590,#96591,#96592,#96593,#96594,#96595,
#96596,#96597,#96598,#96599,#96600,#96601,#96602,#96603,#96604,#96605,#96606,
#96607,#96608,#96609,#96610,#96611,#96612,#96613,#96614,#96615,#96616,#96617,
#96618,#96619,#96620,#96621,#96622,#96623,#96624,#96625,#96626,#96627,#96628,
#96629,#96630,#96631,#96632,#96633,#96634,#96635,#96636,#96637,#96638,#96639,
#96640,#96641,#96642,#96643,#96644,#96645,#96646,#96647,#96648,#96649,#96650,
#96651,#96652,#96653,#96654,#96655,#96656,#96657,#96658,#96659,#96660,#96661,
#96662,#96663,#96664,#96665,#96666,#96667,#96668,#96669,#96670,#96671,#96672,
#96673,#96674,#96675,#96676,#96677,#96678,#96679,#96680,#96681,#96682,#96683,
#96684,#96685,#96686,#96687,#96688,#96689,#96690,#96691,#96692,#96693,#96694,
#96695,#96696,#96697,#96698,#96699,#96700,#96701,#96702,#96703,#96704,#96705,
#96706,#96707,#96708,#96709,#96710,#96711,#96712,#96713,#96714,#96715,#96716,
#96717,#96718,#96719,#96720,#96721,#96722,#96723,#96724,#96725,#96726,#96727,
#96728,#96729,#96730,#96731,#96732,#96733,#96734,#96735,#96736,#96737,#96738,
#96739,#96740,#96741,#96742,#96743,#96744,#96745,#96746,#96747,#96748,#96749,
#96750,#96751,#96752,#96753,#96754,#96755,#96756,#96757,#96758,#96759,#96760,
#96761,#96762,#96763,#96764,#96765,#96766,#96767,#96768,#96769,#96770,#96771,
#96772,#96773,#96774,#96775,#96776,#96777,#96778,#96779,#96780,#96781,#96782,
#96783,#96784,#96785,#96786,#96787,#96788,#96789,#96790,#96791,#96792,#96793,
#96794,#96795,#96796,#96797,#96798,#96799,#96800,#96801,#96802,#96803,#96804,
#96805,#96806,#96807,#96808,#96809,#96810,#96811,#96812,#96813,#96814,#96815,
#96816,#96817,#96818,#96819,#96820,#96821,#96822,#96823,#96824,#96825,#96826,
#96827,#96828,#96829,#96830,#96831,#96832,#96833,#96834,#96835,#96836,#96837,
#96838,#96839,#96840,#96841,#96842,#96843,#96844,#96845,#96846,#96847,#96848,
#96849,#96850,#96851,#96852,#96853,#96854,#96855),.UNSPECIFIED.,.F.,.F.,
(4,3,3,3,3,3,3,3,3,3,3,3,3,3,3,3,3,3,3,3,3,3,3,3,3,3,3,3,3,3,3,3,3,3,3,
3,3,3,3,3,3,3,3,3,3,3,3,3,3,3,3,3,3,3,3,3,3,3,3,3,3,3,3,3,3,3,3,3,3,3,3,
3,3,3,3,3,3,3,3,3,3,3,3,3,3,3,3,3,3,3,3,3,3,3,3,3,3,3,3,3,3,3,3,3,3,3,3,
3,3,3,3,3,3,3,3,3,3,3,3,3,3,3,3,3,3,3,3,3,3,3,3,3,3,3,3,3,3,3,3,3,3,3,3,
3,3,3,3,3,3,3,3,3,3,3,3,3,3,3,3,3,3,3,3,3,3,3,3,3,3,3,3,3,3,3,3,3,3,3,3,
3,3,3,3,3,3,3,3,3,3,3,3,3,3,3,3,3,3,3,3,3,3,3,3,3,3,3,3,3,3,3,3,3,3,3,3,
3,3,3,3,3,3,3,3,3,3,3,3,3,3,3,3,3,3,3,3,3,3,3,3,3,3,3,3,3,3,3,3,3,3,3,3,
3,3,3,3,3,3,3,3,3,3,3,3,3,3,3,3,3,3,3,3,3,3,3,3,3,3,3,3,3,3,3,3,3,3,3,3,
3,3,3,3,3,3,3,3,3,3,3,3,3,3,3,3,3,3,3,3,3,3,3,3,3,3,3,3,3,3,3,3,3,3,3,3,
3,3,3,3,3,3,3,3,3,3,3,3,3,3,3,3,3,3,3,3,3,3,3,3,3,3,3,3,3,3,3,3,3,3,3,3,
3,3,3,3,3,3,3,3,3,3,3,3,3,3,3,3,3,3,3,3,3,3,3,3,3,3,3,3,3,3,3,3,3,3,3,3,
3,4),(-1.,-0.991071428571429,-0.991071405973057,-0.982142857142857,-0.982142834599964,
-0.973214285714286,-0.973214275566846,-0.964285714285714,-0.955357148041666,
-0.955357142857143,-0.946428577574046,-0.946428571428571,-0.937500003529489,
-0.9375,-0.928571433763255,-0.928571428571429,-0.919642857142857,-0.919642854683641,
-0.910714285714286,-0.910714277856615,-0.90397538929407,-0.901785714285714,
-0.896448418480331,-0.892857142857143,-0.892857035697021,-0.888647751552121,
-0.884506308889022,-0.883928673279972,-0.883928571428571,-0.88041123636024,
-0.876936336614861,-0.875,-0.874999573070411,-0.871773427601126,-0.868596771569603,
-0.866071877050543,-0.866071428571429,-0.863553536977713,-0.861044051593477,
-0.858566757473106,-0.857142933290389,-0.857142857142857,-0.854570729186596,
-0.852678571428572,-0.85068776613329,-0.848709234709232,-0.848214285714286,
-0.846942082102984,-0.845982142857143,-0.845238122918132,-0.844308035714286,
-0.842397782896502,-0.84048082150259,-0.839285714285714,-0.836995449126508,
-0.834821428571428,-0.833333712411568,-0.832589285714286,-0.831404902334418,
-0.830357142857143,-0.828409477636648,-0.826459457474174,-0.825892857142857,
-0.824172305158491,-0.822455192368131,-0.821428571428571,-0.821428483905876,
-0.819673336332699,-0.817918766447867,-0.816964285714285,-0.814732142857143,
-0.812990646808756,-0.8125,-0.81036867528272,-0.809523164919251,-0.807406437369691,
-0.805288805989849,-0.803571428571428,-0.801586675846038,-0.798563483815412,
-0.795467160554859,-0.794642857142857,-0.793650901470626,-0.790649071482189,
-0.787671978429273,-0.785714352289099,-0.785714285714286,-0.783406367608846,
-0.781098449503405,-0.779191458689562,-0.777780811792261,-0.777453986656465,
-0.775780896057209,-0.774094604477016,-0.773809523809524,-0.771455749275321,
-0.76983811830604,-0.769213886916033,-0.767482043422238,-0.765748581194053,
-0.765559324410398,-0.763527082629347,-0.761904879293183,-0.761904761904762,
-0.760211049423132,-0.758515188736367,-0.757289982687192,-0.755564339818027,
-0.753968278094141,-0.753644991343596,-0.751592831764285,-0.75,-0.748096146219864,
-0.747767857142857,-0.74602971015346,-0.743681153771395,-0.741326561883123,
-0.741071428571428,-0.739858902252659,-0.738839285714285,-0.738095637949478,
-0.737165178571428,-0.735178034352797,-0.734654017857143,-0.732935246119744,
-0.732142857142857,-0.730345907498532,-0.728557322034361,-0.727678571428572,
-0.726190464852684,-0.725446428571429,-0.724330357142857,-0.723214285714286,
-0.72132026187379,-0.71941280023548,-0.71875,-0.717118396276431,-0.71548846609358,
-0.714285714285714,-0.714284569279444,-0.712216868730684,-0.710146110364231,
-0.708333333333333,-0.706148636368604,-0.70398158883087,-0.702381597545649,
-0.702380952380952,-0.700040414155766,-0.697649358235872,-0.695270917610902,
-0.692873554043546,-0.690611885254948,-0.69047619047619,-0.690474022748346,
-0.688991753412322,-0.687509575139147,-0.686507936507937,-0.68452380952381,
-0.682539682539683,-0.680209262317156,-0.678571642685386,-0.676249377708499,
-0.674603174603175,-0.672618218450647,-0.670006806663296,-0.667384818573573,
-0.666667242024944,-0.666666666666667,-0.663694851668887,-0.660671770900525,
-0.658730158730159,-0.658729982998985,-0.655241597700335,-0.651709329701969,
-0.650793945959924,-0.650793650793651,-0.646576917414535,-0.642857379584437,
-0.642857142857143,-0.637731109382087,-0.634921028244712,-0.634920634920635,
-0.627838030023722,-0.626984353632836,-0.626984126984127,-0.622201404100147,
-0.619047619047619,-0.619047284573871,-0.613777427854794,-0.608408257537255,
-0.607142857142857,-0.60714284698062,-0.599891750889435,-0.595238125156089,
-0.595238095238095,-0.586965854968285,-0.583333340606969,-0.583333333333333,
-0.573165496153514,-0.571428587757185,-0.571428571428571,-0.559523813319172,
-0.55952380952381,-0.547619052116877,-0.547619047619048,-0.535714288280767,
-0.535714285714286,-0.523809523809524,-0.515873015873016,-0.507936512944415,
-0.507936507936508,-0.5,-0.499999996192246,-0.492063492063492,-0.492063478932126,
-0.484366949200099,-0.481481481481481,-0.481481440867044,-0.476190476190476,
-0.476190397017408,-0.471865439838946,-0.468254089647458,-0.468253968253968,
-0.464527668076928,-0.460836274986932,-0.46031746031746,-0.460317411536264,
-0.457262710573874,-0.454249774708069,-0.452381581581904,-0.452380952380952,
-0.449658807753246,-0.446917421123731,-0.444194891123593,-0.441559195015103,
-0.44047619047619,-0.440475982902852,-0.438215137353949,-0.435950436844339,
-0.43452380952381,-0.432258637549228,-0.430021071347414,-0.428571428571429,
-0.428568978804424,-0.426612283828262,-0.424615914690795,-0.422619545553327,
-0.422619047619048,-0.42082140712734,-0.419022095758401,-0.417226299865472,
-0.416666926024893,-0.416666666666667,-0.414295625247005,-0.411934470395318,
-0.410714285714286,-0.408493656754785,-0.406283905537045,-0.404761904761905,
-0.404761500519256,-0.403096206743634,-0.401430208287845,-0.400793650793651,
-0.398674168851715,-0.396825396825397,-0.394841709488377,-0.392858022151356,
-0.390873455520123,-0.388888888888889,-0.38719943767456,-0.386904761904762,
-0.385050373824101,-0.383928571428572,-0.382549746643403,-0.381171896725573,
-0.380952388360775,-0.380952380952381,-0.378568097677262,-0.376234421773945,
-0.375661375661376,-0.373868318870882,-0.372088527038354,-0.370867219366802,
-0.369169637070213,-0.369047893358194,-0.367973292223084,-0.365573066819849,
-0.365079365079365,-0.363318762554276,-0.363095238095238,-0.361445407401825,
-0.359793003859393,-0.358140218092806,-0.357144903583603,-0.357142857142857,
-0.355473461491447,-0.35379548218963,-0.353174603174603,-0.351784903839666,
-0.351190476190476,-0.34957662682823,-0.349206349206349,-0.34722192436045,
-0.345237499514551,-0.343253670392196,-0.341269841269841,-0.339161731810482,
-0.337301587301587,-0.33531747285813,-0.333333358414672,-0.333333333333333,
-0.33058720143975,-0.32779333713046,-0.32738201480293,-0.324561543223382,
-0.321777713208721,-0.321428782196021,-0.321428571428571,-0.318114135640606,
-0.314667391319921,-0.311149612851616,-0.309524729436134,-0.30952380952381,
-0.306184336181973,-0.302734751919678,-0.299293445712499,-0.297619047619048,
-0.297618380297086,-0.293681890016858,-0.289613420134287,-0.285714341509276,
-0.285714285714286,-0.280358734025149,-0.274868515762482,-0.273809523809524,
-0.27380952123257,-0.267412328789522,-0.261904900810491,-0.261904761904762,
-0.255586576240464,-0.250000586120232,-0.25,-0.242926748541942,-0.238095989407649,
-0.236119277627551,-0.230159085420616,-0.23015873015873,-0.225712370063969,
-0.222222557900205,-0.222222222222222,-0.218457566983552,-0.21463599506096,
-0.214286334007192,-0.214285714285714,-0.208717915545674,-0.202946280865649,
-0.202381436484301,-0.202380952380952,-0.195616125035644,-0.190476317028105,
-0.19047619047619,-0.182509579807485,-0.178571468264927,-0.178571428571429,
-0.166666671858936,-0.166666666666667,-0.154761913973698,-0.154761904761905,
-0.142857150422022,-0.142857142857143,-0.133928577558453,-0.133928571428571,
-0.125000004530461,-0.125,-0.116071431663786,-0.116071428571429,-0.107142857142857,
-0.0982142857142857,-0.0892857142857143,-0.0803571428571428,-0.0714285714285714,
-0.0714285676312334,-0.0625,-0.0624999926286917,-0.0535714285714286,-0.0535714184078512,
-0.0446428571428571,-0.0446428453333455,-0.0357142857142857,-0.0357142806094605,
-0.0267857266263663,-0.0267857142857143,-0.0178571772374333,-0.0178571428571429,
-0.00892861062247156,-0.00892857142857143,0.),.UNSPECIFIED.);
#8001=B_SPLINE_CURVE_WITH_KNOTS('',3,(#96856,#96857,#96858,#96859,#96860,
#96861,#96862,#96863,#96864,#96865,#96866,#96867,#96868,#96869,#96870,#96871,
#96872,#96873,#96874,#96875,#96876,#96877),.UNSPECIFIED.,.F.,.F.,(4,2,2,
2,2,2,2,2,2,2,4),(2.02792568943256E-6,0.0187194797883834,0.0270317198253142,
0.0296490618871348,0.030599511546207,0.0312029606220119,0.0317333938792736,
0.0323700195550393,0.0334848245376639,0.0361983254288313,0.0852348509526712),
 .UNSPECIFIED.);
#8002=B_SPLINE_CURVE_WITH_KNOTS('',3,(#96878,#96879,#96880,#96881,#96882,
#96883,#96884,#96885,#96886,#96887,#96888,#96889,#96890,#96891,#96892,#96893,
#96894,#96895,#96896,#96897,#96898,#96899,#96900,#96901,#96902,#96903,#96904,
#96905,#96906,#96907,#96908,#96909,#96910,#96911,#96912,#96913,#96914,#96915,
#96916,#96917,#96918,#96919,#96920),.UNSPECIFIED.,.F.,.F.,(4,3,3,3,3,3,
3,3,3,3,3,3,3,3,4),(1.19276284565608E-6,0.00921698783890213,0.0187194648875106,
0.0270315500022582,0.0296489825432181,0.0305994303610185,0.031202876530675,
0.0317333058143584,0.0323699244425081,0.0334847132766303,0.0361981632966636,
0.0484645045289161,0.0595378820786154,0.0710363226551942,0.0852410290365269),
 .UNSPECIFIED.);
#9705=VERTEX_POINT('',#93192);
#9706=VERTEX_POINT('',#93193);
#9707=VERTEX_POINT('',#93228);
#9708=VERTEX_POINT('',#93239);
#9709=VERTEX_POINT('',#93250);
#9710=VERTEX_POINT('',#93257);
#9711=VERTEX_POINT('',#93268);
#9712=VERTEX_POINT('',#93286);
#9713=VERTEX_POINT('',#93287);
#9714=VERTEX_POINT('',#93322);
#9715=VERTEX_POINT('',#93333);
#9716=VERTEX_POINT('',#93344);
#9717=VERTEX_POINT('',#93351);
#9718=VERTEX_POINT('',#93358);
#12543=EDGE_CURVE('',#9705,#9706,#7985,.T.);
#12544=EDGE_CURVE('',#9706,#9705,#3151,.T.);
#12545=EDGE_CURVE('',#9705,#9707,#7986,.T.);
#12546=EDGE_CURVE('',#9707,#9708,#7987,.T.);
#12547=EDGE_CURVE('',#9708,#9709,#7988,.T.);
#12548=EDGE_CURVE('',#9709,#9710,#7989,.T.);
#12549=EDGE_CURVE('',#9710,#9711,#7990,.T.);
#12550=EDGE_CURVE('',#9711,#9706,#7991,.T.);
#12551=EDGE_CURVE('',#9712,#9713,#7992,.T.);
#12552=EDGE_CURVE('',#9713,#9712,#3152,.T.);
#12553=EDGE_CURVE('',#9714,#9712,#7993,.T.);
#12554=EDGE_CURVE('',#9715,#9714,#7994,.T.);
#12555=EDGE_CURVE('',#9715,#9716,#7995,.T.);
#12556=EDGE_CURVE('',#9717,#9716,#7996,.T.);
#12557=EDGE_CURVE('',#9718,#9717,#7997,.T.);
#12558=EDGE_CURVE('',#9713,#9718,#7998,.T.);
#12559=EDGE_CURVE('',#9711,#9714,#7999,.T.);
#12560=EDGE_CURVE('',#9707,#9718,#8000,.T.);
#12561=EDGE_CURVE('',#9709,#9708,#8001,.T.);
#12562=EDGE_CURVE('',#9716,#9715,#8002,.T.);
#18137=ORIENTED_EDGE('',*,*,#12543,.F.);
#18138=ORIENTED_EDGE('',*,*,#12544,.F.);
#18139=ORIENTED_EDGE('',*,*,#12544,.T.);
#18140=ORIENTED_EDGE('',*,*,#12545,.T.);
#18141=ORIENTED_EDGE('',*,*,#12546,.T.);
#18142=ORIENTED_EDGE('',*,*,#12547,.T.);
#18143=ORIENTED_EDGE('',*,*,#12548,.T.);
#18144=ORIENTED_EDGE('',*,*,#12549,.T.);
#18145=ORIENTED_EDGE('',*,*,#12550,.T.);
#18146=ORIENTED_EDGE('',*,*,#12551,.F.);
#18147=ORIENTED_EDGE('',*,*,#12552,.F.);
#18148=ORIENTED_EDGE('',*,*,#12552,.T.);
#18149=ORIENTED_EDGE('',*,*,#12553,.F.);
#18150=ORIENTED_EDGE('',*,*,#12554,.F.);
#18151=ORIENTED_EDGE('',*,*,#12555,.T.);
#18152=ORIENTED_EDGE('',*,*,#12556,.F.);
#18153=ORIENTED_EDGE('',*,*,#12557,.F.);
#18154=ORIENTED_EDGE('',*,*,#12558,.F.);
#18155=ORIENTED_EDGE('',*,*,#12543,.T.);
#18156=ORIENTED_EDGE('',*,*,#12550,.F.);
#18157=ORIENTED_EDGE('',*,*,#12559,.T.);
#18158=ORIENTED_EDGE('',*,*,#12553,.T.);
#18159=ORIENTED_EDGE('',*,*,#12551,.T.);
#18160=ORIENTED_EDGE('',*,*,#12558,.T.);
#18161=ORIENTED_EDGE('',*,*,#12560,.F.);
#18162=ORIENTED_EDGE('',*,*,#12545,.F.);
#18163=ORIENTED_EDGE('',*,*,#12547,.F.);
#18164=ORIENTED_EDGE('',*,*,#12561,.F.);
#18165=ORIENTED_EDGE('',*,*,#12555,.F.);
#18166=ORIENTED_EDGE('',*,*,#12562,.F.);
#18167=ORIENTED_EDGE('',*,*,#12561,.T.);
#18168=ORIENTED_EDGE('',*,*,#12546,.F.);
#18169=ORIENTED_EDGE('',*,*,#12560,.T.);
#18170=ORIENTED_EDGE('',*,*,#12557,.T.);
#18171=ORIENTED_EDGE('',*,*,#12556,.T.);
#18172=ORIENTED_EDGE('',*,*,#12562,.T.);
#18173=ORIENTED_EDGE('',*,*,#12554,.T.);
#18174=ORIENTED_EDGE('',*,*,#12559,.F.);
#18175=ORIENTED_EDGE('',*,*,#12549,.F.);
#18176=ORIENTED_EDGE('',*,*,#12548,.F.);
#18936=B_SPLINE_SURFACE_WITH_KNOTS('',3,3,((#93381,#93382,#93383,#93384,
#93385,#93386,#93387,#93388,#93389,#93390,#93391,#93392,#93393,#93394,#93395,
#93396,#93397,#93398,#93399,#93400,#93401,#93402,#93403,#93404,#93405,#93406,
#93407,#93408,#93409,#93410,#93411,#93412,#93413,#93414,#93415,#93416,#93417,
#93418,#93419,#93420,#93421,#93422,#93423,#93424,#93425,#93426,#93427,#93428,
#93429,#93430,#93431,#93432,#93433,#93434,#93435,#93436,#93437,#93438,#93439,
#93440,#93441,#93442,#93443,#93444,#93445,#93446,#93447,#93448,#93449,#93450,
#93451,#93452,#93453,#93454,#93455,#93456,#93457,#93458,#93459,#93460,#93461,
#93462,#93463,#93464,#93465,#93466,#93467,#93468,#93469,#93470,#93471,#93472,
#93473,#93474,#93475,#93476,#93477,#93478,#93479,#93480,#93481,#93482,#93483,
#93484,#93485,#93486,#93487,#93488,#93489,#93490),(#93491,#93492,#93493,
#93494,#93495,#93496,#93497,#93498,#93499,#93500,#93501,#93502,#93503,#93504,
#93505,#93506,#93507,#93508,#93509,#93510,#93511,#93512,#93513,#93514,#93515,
#93516,#93517,#93518,#93519,#93520,#93521,#93522,#93523,#93524,#93525,#93526,
#93527,#93528,#93529,#93530,#93531,#93532,#93533,#93534,#93535,#93536,#93537,
#93538,#93539,#93540,#93541,#93542,#93543,#93544,#93545,#93546,#93547,#93548,
#93549,#93550,#93551,#93552,#93553,#93554,#93555,#93556,#93557,#93558,#93559,
#93560,#93561,#93562,#93563,#93564,#93565,#93566,#93567,#93568,#93569,#93570,
#93571,#93572,#93573,#93574,#93575,#93576,#93577,#93578,#93579,#93580,#93581,
#93582,#93583,#93584,#93585,#93586,#93587,#93588,#93589,#93590,#93591,#93592,
#93593,#93594,#93595,#93596,#93597,#93598,#93599,#93600),(#93601,#93602,
#93603,#93604,#93605,#93606,#93607,#93608,#93609,#93610,#93611,#93612,#93613,
#93614,#93615,#93616,#93617,#93618,#93619,#93620,#93621,#93622,#93623,#93624,
#93625,#93626,#93627,#93628,#93629,#93630,#93631,#93632,#93633,#93634,#93635,
#93636,#93637,#93638,#93639,#93640,#93641,#93642,#93643,#93644,#93645,#93646,
#93647,#93648,#93649,#93650,#93651,#93652,#93653,#93654,#93655,#93656,#93657,
#93658,#93659,#93660,#93661,#93662,#93663,#93664,#93665,#93666,#93667,#93668,
#93669,#93670,#93671,#93672,#93673,#93674,#93675,#93676,#93677,#93678,#93679,
#93680,#93681,#93682,#93683,#93684,#93685,#93686,#93687,#93688,#93689,#93690,
#93691,#93692,#93693,#93694,#93695,#93696,#93697,#93698,#93699,#93700,#93701,
#93702,#93703,#93704,#93705,#93706,#93707,#93708,#93709,#93710),(#93711,
#93712,#93713,#93714,#93715,#93716,#93717,#93718,#93719,#93720,#93721,#93722,
#93723,#93724,#93725,#93726,#93727,#93728,#93729,#93730,#93731,#93732,#93733,
#93734,#93735,#93736,#93737,#93738,#93739,#93740,#93741,#93742,#93743,#93744,
#93745,#93746,#93747,#93748,#93749,#93750,#93751,#93752,#93753,#93754,#93755,
#93756,#93757,#93758,#93759,#93760,#93761,#93762,#93763,#93764,#93765,#93766,
#93767,#93768,#93769,#93770,#93771,#93772,#93773,#93774,#93775,#93776,#93777,
#93778,#93779,#93780,#93781,#93782,#93783,#93784,#93785,#93786,#93787,#93788,
#93789,#93790,#93791,#93792,#93793,#93794,#93795,#93796,#93797,#93798,#93799,
#93800,#93801,#93802,#93803,#93804,#93805,#93806,#93807,#93808,#93809,#93810,
#93811,#93812,#93813,#93814,#93815,#93816,#93817,#93818,#93819,#93820),
(#93821,#93822,#93823,#93824,#93825,#93826,#93827,#93828,#93829,#93830,
#93831,#93832,#93833,#93834,#93835,#93836,#93837,#93838,#93839,#93840,#93841,
#93842,#93843,#93844,#93845,#93846,#93847,#93848,#93849,#93850,#93851,#93852,
#93853,#93854,#93855,#93856,#93857,#93858,#93859,#93860,#93861,#93862,#93863,
#93864,#93865,#93866,#93867,#93868,#93869,#93870,#93871,#93872,#93873,#93874,
#93875,#93876,#93877,#93878,#93879,#93880,#93881,#93882,#93883,#93884,#93885,
#93886,#93887,#93888,#93889,#93890,#93891,#93892,#93893,#93894,#93895,#93896,
#93897,#93898,#93899,#93900,#93901,#93902,#93903,#93904,#93905,#93906,#93907,
#93908,#93909,#93910,#93911,#93912,#93913,#93914,#93915,#93916,#93917,#93918,
#93919,#93920,#93921,#93922,#93923,#93924,#93925,#93926,#93927,#93928,#93929,
#93930),(#93931,#93932,#93933,#93934,#93935,#93936,#93937,#93938,#93939,
#93940,#93941,#93942,#93943,#93944,#93945,#93946,#93947,#93948,#93949,#93950,
#93951,#93952,#93953,#93954,#93955,#93956,#93957,#93958,#93959,#93960,#93961,
#93962,#93963,#93964,#93965,#93966,#93967,#93968,#93969,#93970,#93971,#93972,
#93973,#93974,#93975,#93976,#93977,#93978,#93979,#93980,#93981,#93982,#93983,
#93984,#93985,#93986,#93987,#93988,#93989,#93990,#93991,#93992,#93993,#93994,
#93995,#93996,#93997,#93998,#93999,#94000,#94001,#94002,#94003,#94004,#94005,
#94006,#94007,#94008,#94009,#94010,#94011,#94012,#94013,#94014,#94015,#94016,
#94017,#94018,#94019,#94020,#94021,#94022,#94023,#94024,#94025,#94026,#94027,
#94028,#94029,#94030,#94031,#94032,#94033,#94034,#94035,#94036,#94037,#94038,
#94039,#94040),(#94041,#94042,#94043,#94044,#94045,#94046,#94047,#94048,
#94049,#94050,#94051,#94052,#94053,#94054,#94055,#94056,#94057,#94058,#94059,
#94060,#94061,#94062,#94063,#94064,#94065,#94066,#94067,#94068,#94069,#94070,
#94071,#94072,#94073,#94074,#94075,#94076,#94077,#94078,#94079,#94080,#94081,
#94082,#94083,#94084,#94085,#94086,#94087,#94088,#94089,#94090,#94091,#94092,
#94093,#94094,#94095,#94096,#94097,#94098,#94099,#94100,#94101,#94102,#94103,
#94104,#94105,#94106,#94107,#94108,#94109,#94110,#94111,#94112,#94113,#94114,
#94115,#94116,#94117,#94118,#94119,#94120,#94121,#94122,#94123,#94124,#94125,
#94126,#94127,#94128,#94129,#94130,#94131,#94132,#94133,#94134,#94135,#94136,
#94137,#94138,#94139,#94140,#94141,#94142,#94143,#94144,#94145,#94146,#94147,
#94148,#94149,#94150),(#94151,#94152,#94153,#94154,#94155,#94156,#94157,
#94158,#94159,#94160,#94161,#94162,#94163,#94164,#94165,#94166,#94167,#94168,
#94169,#94170,#94171,#94172,#94173,#94174,#94175,#94176,#94177,#94178,#94179,
#94180,#94181,#94182,#94183,#94184,#94185,#94186,#94187,#94188,#94189,#94190,
#94191,#94192,#94193,#94194,#94195,#94196,#94197,#94198,#94199,#94200,#94201,
#94202,#94203,#94204,#94205,#94206,#94207,#94208,#94209,#94210,#94211,#94212,
#94213,#94214,#94215,#94216,#94217,#94218,#94219,#94220,#94221,#94222,#94223,
#94224,#94225,#94226,#94227,#94228,#94229,#94230,#94231,#94232,#94233,#94234,
#94235,#94236,#94237,#94238,#94239,#94240,#94241,#94242,#94243,#94244,#94245,
#94246,#94247,#94248,#94249,#94250,#94251,#94252,#94253,#94254,#94255,#94256,
#94257,#94258,#94259,#94260),(#94261,#94262,#94263,#94264,#94265,#94266,
#94267,#94268,#94269,#94270,#94271,#94272,#94273,#94274,#94275,#94276,#94277,
#94278,#94279,#94280,#94281,#94282,#94283,#94284,#94285,#94286,#94287,#94288,
#94289,#94290,#94291,#94292,#94293,#94294,#94295,#94296,#94297,#94298,#94299,
#94300,#94301,#94302,#94303,#94304,#94305,#94306,#94307,#94308,#94309,#94310,
#94311,#94312,#94313,#94314,#94315,#94316,#94317,#94318,#94319,#94320,#94321,
#94322,#94323,#94324,#94325,#94326,#94327,#94328,#94329,#94330,#94331,#94332,
#94333,#94334,#94335,#94336,#94337,#94338,#94339,#94340,#94341,#94342,#94343,
#94344,#94345,#94346,#94347,#94348,#94349,#94350,#94351,#94352,#94353,#94354,
#94355,#94356,#94357,#94358,#94359,#94360,#94361,#94362,#94363,#94364,#94365,
#94366,#94367,#94368,#94369,#94370),(#94371,#94372,#94373,#94374,#94375,
#94376,#94377,#94378,#94379,#94380,#94381,#94382,#94383,#94384,#94385,#94386,
#94387,#94388,#94389,#94390,#94391,#94392,#94393,#94394,#94395,#94396,#94397,
#94398,#94399,#94400,#94401,#94402,#94403,#94404,#94405,#94406,#94407,#94408,
#94409,#94410,#94411,#94412,#94413,#94414,#94415,#94416,#94417,#94418,#94419,
#94420,#94421,#94422,#94423,#94424,#94425,#94426,#94427,#94428,#94429,#94430,
#94431,#94432,#94433,#94434,#94435,#94436,#94437,#94438,#94439,#94440,#94441,
#94442,#94443,#94444,#94445,#94446,#94447,#94448,#94449,#94450,#94451,#94452,
#94453,#94454,#94455,#94456,#94457,#94458,#94459,#94460,#94461,#94462,#94463,
#94464,#94465,#94466,#94467,#94468,#94469,#94470,#94471,#94472,#94473,#94474,
#94475,#94476,#94477,#94478,#94479,#94480)),.UNSPECIFIED.,.F.,.F.,.F.,(4,
1,1,1,1,1,1,4),(4,1,1,1,1,1,1,1,1,1,1,1,1,1,1,1,1,1,1,1,1,1,1,1,1,1,1,1,
1,1,1,1,1,1,1,1,1,1,1,1,1,1,1,1,1,1,1,1,1,1,1,1,1,1,1,1,1,1,1,1,1,1,1,1,
1,1,1,1,1,1,1,1,1,1,1,1,1,1,1,1,1,1,1,1,1,1,1,1,1,1,1,1,1,1,1,1,1,1,1,1,
1,1,1,1,1,1,1,4),(-2.15967935518058,-1.67714812064519,-1.20351419577799,
-0.729880270910797,-0.2562463460436,0.217387578823596,0.691021503690793,
1.17374330931374),(-0.00388260537544204,0.00892857142857143,0.0178571428571429,
0.0267857142857143,0.0357142857142857,0.0446428571428571,0.0535714285714286,
0.0625,0.0714285714285714,0.0803571428571428,0.0892857142857143,0.0982142857142857,
0.107142857142857,0.116071428571429,0.125,0.133928571428571,0.142857142857143,
0.154761904761905,0.166666666666667,0.178571428571429,0.19047619047619,
0.202380952380952,0.214285714285714,0.222222222222222,0.23015873015873,
0.238095238095238,0.25,0.261904761904762,0.273809523809524,0.285714285714286,
0.297619047619048,0.30952380952381,0.321428571428571,0.333333333333333,
0.341269841269841,0.349206349206349,0.357142857142857,0.365079365079365,
0.375661375661376,0.380952380952381,0.388888888888889,0.396825396825397,
0.404761904761905,0.416666666666667,0.428571428571429,0.43452380952381,
0.44047619047619,0.452380952380952,0.46031746031746,0.468253968253968,0.476190476190476,
0.481481481481481,0.492063492063492,0.5,0.507936507936508,0.515873015873016,
0.523809523809524,0.535714285714286,0.547619047619048,0.55952380952381,
0.571428571428571,0.583333333333333,0.595238095238095,0.607142857142857,
0.619047619047619,0.626984126984127,0.634920634920635,0.642857142857143,
0.650793650793651,0.658730158730159,0.666666666666667,0.674603174603175,
0.682539682539683,0.69047619047619,0.702380952380952,0.708333333333333,
0.714285714285714,0.723214285714286,0.732142857142857,0.741071428571428,
0.75,0.761904761904762,0.773809523809524,0.785714285714286,0.794642857142857,
0.803571428571428,0.8125,0.821428571428571,0.830357142857143,0.839285714285714,
0.848214285714286,0.857142857142857,0.866071428571429,0.875,0.883928571428571,
0.892857142857143,0.901785714285714,0.910714285714286,0.919642857142857,
0.928571428571429,0.9375,0.946428571428571,0.955357142857143,0.964285714285714,
0.973214285714286,0.982142857142857,0.991071428571429,1.00388260537544),
 .UNSPECIFIED.);
#18937=B_SPLINE_SURFACE_WITH_KNOTS('',3,3,((#96921,#96922,#96923,#96924,
#96925,#96926,#96927,#96928,#96929,#96930,#96931,#96932,#96933,#96934,#96935,
#96936,#96937,#96938,#96939,#96940,#96941,#96942,#96943,#96944,#96945,#96946,
#96947,#96948,#96949,#96950,#96951,#96952,#96953,#96954,#96955,#96956,#96957,
#96958,#96959,#96960,#96961,#96962,#96963,#96964,#96965,#96966,#96967,#96968,
#96969,#96970,#96971,#96972,#96973,#96974,#96975,#96976,#96977,#96978,#96979,
#96980,#96981,#96982,#96983,#96984,#96985,#96986,#96987,#96988,#96989,#96990,
#96991,#96992,#96993,#96994,#96995,#96996,#96997,#96998,#96999,#97000,#97001,
#97002,#97003,#97004,#97005,#97006,#97007,#97008,#97009,#97010,#97011,#97012,
#97013,#97014,#97015,#97016,#97017,#97018,#97019,#97020,#97021,#97022,#97023,
#97024,#97025,#97026,#97027),(#97028,#97029,#97030,#97031,#97032,#97033,
#97034,#97035,#97036,#97037,#97038,#97039,#97040,#97041,#97042,#97043,#97044,
#97045,#97046,#97047,#97048,#97049,#97050,#97051,#97052,#97053,#97054,#97055,
#97056,#97057,#97058,#97059,#97060,#97061,#97062,#97063,#97064,#97065,#97066,
#97067,#97068,#97069,#97070,#97071,#97072,#97073,#97074,#97075,#97076,#97077,
#97078,#97079,#97080,#97081,#97082,#97083,#97084,#97085,#97086,#97087,#97088,
#97089,#97090,#97091,#97092,#97093,#97094,#97095,#97096,#97097,#97098,#97099,
#97100,#97101,#97102,#97103,#97104,#97105,#97106,#97107,#97108,#97109,#97110,
#97111,#97112,#97113,#97114,#97115,#97116,#97117,#97118,#97119,#97120,#97121,
#97122,#97123,#97124,#97125,#97126,#97127,#97128,#97129,#97130,#97131,#97132,
#97133,#97134),(#97135,#97136,#97137,#97138,#97139,#97140,#97141,#97142,
#97143,#97144,#97145,#97146,#97147,#97148,#97149,#97150,#97151,#97152,#97153,
#97154,#97155,#97156,#97157,#97158,#97159,#97160,#97161,#97162,#97163,#97164,
#97165,#97166,#97167,#97168,#97169,#97170,#97171,#97172,#97173,#97174,#97175,
#97176,#97177,#97178,#97179,#97180,#97181,#97182,#97183,#97184,#97185,#97186,
#97187,#97188,#97189,#97190,#97191,#97192,#97193,#97194,#97195,#97196,#97197,
#97198,#97199,#97200,#97201,#97202,#97203,#97204,#97205,#97206,#97207,#97208,
#97209,#97210,#97211,#97212,#97213,#97214,#97215,#97216,#97217,#97218,#97219,
#97220,#97221,#97222,#97223,#97224,#97225,#97226,#97227,#97228,#97229,#97230,
#97231,#97232,#97233,#97234,#97235,#97236,#97237,#97238,#97239,#97240,#97241),
(#97242,#97243,#97244,#97245,#97246,#97247,#97248,#97249,#97250,#97251,
#97252,#97253,#97254,#97255,#97256,#97257,#97258,#97259,#97260,#97261,#97262,
#97263,#97264,#97265,#97266,#97267,#97268,#97269,#97270,#97271,#97272,#97273,
#97274,#97275,#97276,#97277,#97278,#97279,#97280,#97281,#97282,#97283,#97284,
#97285,#97286,#97287,#97288,#97289,#97290,#97291,#97292,#97293,#97294,#97295,
#97296,#97297,#97298,#97299,#97300,#97301,#97302,#97303,#97304,#97305,#97306,
#97307,#97308,#97309,#97310,#97311,#97312,#97313,#97314,#97315,#97316,#97317,
#97318,#97319,#97320,#97321,#97322,#97323,#97324,#97325,#97326,#97327,#97328,
#97329,#97330,#97331,#97332,#97333,#97334,#97335,#97336,#97337,#97338,#97339,
#97340,#97341,#97342,#97343,#97344,#97345,#97346,#97347,#97348),(#97349,
#97350,#97351,#97352,#97353,#97354,#97355,#97356,#97357,#97358,#97359,#97360,
#97361,#97362,#97363,#97364,#97365,#97366,#97367,#97368,#97369,#97370,#97371,
#97372,#97373,#97374,#97375,#97376,#97377,#97378,#97379,#97380,#97381,#97382,
#97383,#97384,#97385,#97386,#97387,#97388,#97389,#97390,#97391,#97392,#97393,
#97394,#97395,#97396,#97397,#97398,#97399,#97400,#97401,#97402,#97403,#97404,
#97405,#97406,#97407,#97408,#97409,#97410,#97411,#97412,#97413,#97414,#97415,
#97416,#97417,#97418,#97419,#97420,#97421,#97422,#97423,#97424,#97425,#97426,
#97427,#97428,#97429,#97430,#97431,#97432,#97433,#97434,#97435,#97436,#97437,
#97438,#97439,#97440,#97441,#97442,#97443,#97444,#97445,#97446,#97447,#97448,
#97449,#97450,#97451,#97452,#97453,#97454,#97455),(#97456,#97457,#97458,
#97459,#97460,#97461,#97462,#97463,#97464,#97465,#97466,#97467,#97468,#97469,
#97470,#97471,#97472,#97473,#97474,#97475,#97476,#97477,#97478,#97479,#97480,
#97481,#97482,#97483,#97484,#97485,#97486,#97487,#97488,#97489,#97490,#97491,
#97492,#97493,#97494,#97495,#97496,#97497,#97498,#97499,#97500,#97501,#97502,
#97503,#97504,#97505,#97506,#97507,#97508,#97509,#97510,#97511,#97512,#97513,
#97514,#97515,#97516,#97517,#97518,#97519,#97520,#97521,#97522,#97523,#97524,
#97525,#97526,#97527,#97528,#97529,#97530,#97531,#97532,#97533,#97534,#97535,
#97536,#97537,#97538,#97539,#97540,#97541,#97542,#97543,#97544,#97545,#97546,
#97547,#97548,#97549,#97550,#97551,#97552,#97553,#97554,#97555,#97556,#97557,
#97558,#97559,#97560,#97561,#97562),(#97563,#97564,#97565,#97566,#97567,
#97568,#97569,#97570,#97571,#97572,#97573,#97574,#97575,#97576,#97577,#97578,
#97579,#97580,#97581,#97582,#97583,#97584,#97585,#97586,#97587,#97588,#97589,
#97590,#97591,#97592,#97593,#97594,#97595,#97596,#97597,#97598,#97599,#97600,
#97601,#97602,#97603,#97604,#97605,#97606,#97607,#97608,#97609,#97610,#97611,
#97612,#97613,#97614,#97615,#97616,#97617,#97618,#97619,#97620,#97621,#97622,
#97623,#97624,#97625,#97626,#97627,#97628,#97629,#97630,#97631,#97632,#97633,
#97634,#97635,#97636,#97637,#97638,#97639,#97640,#97641,#97642,#97643,#97644,
#97645,#97646,#97647,#97648,#97649,#97650,#97651,#97652,#97653,#97654,#97655,
#97656,#97657,#97658,#97659,#97660,#97661,#97662,#97663,#97664,#97665,#97666,
#97667,#97668,#97669)),.UNSPECIFIED.,.F.,.F.,.F.,(4,1,1,1,4),(4,1,1,1,1,
1,1,1,1,1,1,1,1,1,1,1,1,1,1,1,1,1,1,1,1,1,1,1,1,1,1,1,1,1,1,1,1,1,1,1,1,
1,1,1,1,1,1,1,1,1,1,1,1,1,1,1,1,1,1,1,1,1,1,1,1,1,1,1,1,1,1,1,1,1,1,1,1,
1,1,1,1,1,1,1,1,1,1,1,1,1,1,1,1,1,1,1,1,1,1,1,1,1,1,1,4),(1.16465542855799,
1.80060139279568,2.43654735703337,3.28447530935028,4.1324032616672),(0.,
0.00892857142857143,0.0178571428571429,0.0267857142857143,0.0357142857142857,
0.0446428571428571,0.0535714285714286,0.0625,0.0714285714285714,0.0803571428571428,
0.0892857142857143,0.0982142857142857,0.107142857142857,0.116071428571429,
0.125,0.133928571428571,0.142857142857143,0.154761904761905,0.166666666666667,
0.178571428571429,0.19047619047619,0.202380952380952,0.214285714285714,
0.222222222222222,0.23015873015873,0.238095238095238,0.25,0.261904761904762,
0.273809523809524,0.285714285714286,0.297619047619048,0.30952380952381,
0.321428571428571,0.327380952380952,0.333333333333333,0.345238095238095,
0.357142857142857,0.369047619047619,0.380952380952381,0.392857142857143,
0.404761904761905,0.416666666666667,0.422619047619048,0.428571428571429,
0.44047619047619,0.452380952380952,0.46031746031746,0.468253968253968,0.476190476190476,
0.481481481481481,0.492063492063492,0.5,0.507936507936508,0.515873015873016,
0.523809523809524,0.535714285714286,0.547619047619048,0.55952380952381,
0.571428571428571,0.583333333333333,0.595238095238095,0.607142857142857,
0.619047619047619,0.626984126984127,0.634920634920635,0.642857142857143,
0.650793650793651,0.658730158730159,0.666666666666667,0.672619047619048,
0.678571428571429,0.69047619047619,0.702380952380952,0.714285714285714,
0.726190476190476,0.738095238095238,0.746031746031746,0.753968253968254,
0.761904761904762,0.76984126984127,0.777777777777778,0.785714285714286,
0.793650793650794,0.801587301587302,0.809523809523809,0.821428571428571,
0.833333333333333,0.845238095238095,0.857142857142857,0.866071428571429,
0.875,0.883928571428571,0.892857142857143,0.901785714285714,0.910714285714286,
0.919642857142857,0.928571428571429,0.9375,0.946428571428571,0.955357142857143,
0.964285714285714,0.973214285714286,0.982142857142857,0.991071428571429,
1.),.UNSPECIFIED.);
#19939=ADVANCED_FACE('',(#6005),#1634,.T.);
#19940=ADVANCED_FACE('',(#6006),#1635,.T.);
#19941=ADVANCED_FACE('',(#6007),#1636,.F.);
#19942=ADVANCED_FACE('',(#6008),#1637,.F.);
#19943=ADVANCED_FACE('',(#6009,#1774,#1775),#18936,.T.);
#19944=ADVANCED_FACE('',(#6010),#18937,.T.);
#20124=CLOSED_SHELL('',(#19939,#19940,#19941,#19942,#19943,#19944));
#22152=AXIS2_PLACEMENT_3D('',#93190,#27332,#27333);
#22153=AXIS2_PLACEMENT_3D('',#93191,#27334,#27335);
#22154=AXIS2_PLACEMENT_3D('',#93227,#27337,#27338);
#22155=AXIS2_PLACEMENT_3D('',#93285,#27339,#27340);
#22156=AXIS2_PLACEMENT_3D('',#93321,#27342,#27343);
#27332=DIRECTION('axis',(0.,0.,1.));
#27333=DIRECTION('refdir',(1.,0.,0.));
#27334=DIRECTION('center_axis',(1.,0.,0.));
#27335=DIRECTION('ref_axis',(0.,0.,-1.));
#27336=DIRECTION('',(0.,-0.99999354730451,0.00359240161224881));
#27337=DIRECTION('center_axis',(0.027955631445268,-0.00359099757581823,
-0.999602714785683));
#27338=DIRECTION('ref_axis',(0.4350805171232,-0.900259809769442,0.0154019003274739));
#27339=DIRECTION('center_axis',(1.,0.,0.));
#27340=DIRECTION('ref_axis',(0.,0.,-1.));
#27341=DIRECTION('',(0.,0.999993547304682,0.00359240156428263));
#27342=DIRECTION('center_axis',(0.0279556313622445,-0.00359099752787914,
0.999602714788177));
#27343=DIRECTION('ref_axis',(-0.991456520419747,0.127356018817566,0.0281853257583967));
#93190=CARTESIAN_POINT('',(0.,0.,0.));
#93191=CARTESIAN_POINT('Origin',(22.032,0.,0.));
#93192=CARTESIAN_POINT('',(22.0319999995994,-11.5000119847845,0.0228638357956435));
#93193=CARTESIAN_POINT('',(22.032,-10.2055351096819,0.0182135250455447));
#93194=CARTESIAN_POINT('Ctrl Pts',(22.032,-11.5000119837245,0.0228638357581901));
#93195=CARTESIAN_POINT('Ctrl Pts',(22.032,-11.4660039066419,0.98463424605543));
#93196=CARTESIAN_POINT('Ctrl Pts',(22.0320000000025,-11.3136952518557,1.93685858767515));
#93197=CARTESIAN_POINT('Ctrl Pts',(22.0320000000025,-10.8106581948625,3.60550041619086));
#93198=CARTESIAN_POINT('Ctrl Pts',(22.0320000001919,-10.5043379386651,4.32629225339571));
#93199=CARTESIAN_POINT('Ctrl Pts',(22.0320000001919,-9.46446343489987,6.15504317488174));
#93200=CARTESIAN_POINT('Ctrl Pts',(22.0319999999366,-8.72063759985904,6.938122886154));
#93201=CARTESIAN_POINT('Ctrl Pts',(22.0319999999366,-8.03193816956031,7.51949158019168));
#93202=CARTESIAN_POINT('Ctrl Pts',(22.0319999999997,-7.85932443550526,7.63633005181417));
#93203=CARTESIAN_POINT('Ctrl Pts',(22.0319999999997,-7.73686440492364,7.68512650246837));
#93204=CARTESIAN_POINT('Ctrl Pts',(22.0320000000002,-7.71458757555367,7.69219740534354));
#93205=CARTESIAN_POINT('Ctrl Pts',(22.0320000000002,-7.68888585032816,7.69366409920399));
#93206=CARTESIAN_POINT('Ctrl Pts',(22.032,-7.68166282362026,7.69332086239068));
#93207=CARTESIAN_POINT('Ctrl Pts',(22.032,-7.6709934259232,7.69016254445955));
#93208=CARTESIAN_POINT('Ctrl Pts',(22.032,-7.66713809909079,7.68831385381647));
#93209=CARTESIAN_POINT('Ctrl Pts',(22.032,-7.66088557595881,7.68327738229244));
#93210=CARTESIAN_POINT('Ctrl Pts',(22.032,-7.65855096777891,7.68044695877115));
#93211=CARTESIAN_POINT('Ctrl Pts',(22.032,-7.65460320422513,7.67333693309721));
#93212=CARTESIAN_POINT('Ctrl Pts',(22.032,-7.65329985444339,7.66908195382268));
#93213=CARTESIAN_POINT('Ctrl Pts',(22.032,-7.65126894293338,7.65725956689985));
#93214=CARTESIAN_POINT('Ctrl Pts',(22.032,-7.65158753554677,7.64913230233977));
#93215=CARTESIAN_POINT('Ctrl Pts',(22.032,-7.65481301559317,7.62353907721947));
#93216=CARTESIAN_POINT('Ctrl Pts',(22.032,-7.66148618499009,7.6028062413979));
#93217=CARTESIAN_POINT('Ctrl Pts',(22.032,-7.69333704035368,7.52201090468904));
#93218=CARTESIAN_POINT('Ctrl Pts',(22.032,-7.74069889072153,7.43827269921366));
#93219=CARTESIAN_POINT('Ctrl Pts',(22.032,-8.0762146857713,6.89691692694695));
#93220=CARTESIAN_POINT('Ctrl Pts',(22.0320000000002,-8.64551455485788,6.11724445629462));
#93221=CARTESIAN_POINT('Ctrl Pts',(22.0320000000002,-9.48552373995225,4.32369687901933));
#93222=CARTESIAN_POINT('Ctrl Pts',(22.0319999999999,-9.73628062912841,3.61588039473753));
#93223=CARTESIAN_POINT('Ctrl Pts',(22.0319999999999,-10.1372396947166,1.93922249627196));
#93224=CARTESIAN_POINT('Ctrl Pts',(22.032,-10.2326443525765,0.983079921512957));
#93225=CARTESIAN_POINT('Ctrl Pts',(22.032,-10.2055351096819,0.0182135250456028));
#93226=CARTESIAN_POINT('',(22.032,-5.42639624653361,0.00104482810403733));
#93227=CARTESIAN_POINT('Origin',(21.2976,-10.8528,-1.59247615094671E-14));
#93228=CARTESIAN_POINT('',(20.6563591733144,-11.5926712737699,-0.0152754849923013));
#93229=CARTESIAN_POINT('Ctrl Pts',(22.0319999992972,-11.5000119845197,0.0228638358451183));
#93230=CARTESIAN_POINT('Ctrl Pts',(21.9350321970426,-11.610239680658,0.0205479470244637));
#93231=CARTESIAN_POINT('Ctrl Pts',(21.8275399155968,-11.6829048894223,0.0178027823963555));
#93232=CARTESIAN_POINT('Ctrl Pts',(21.626607745303,-11.7823418227845,0.0125405838911135));
#93233=CARTESIAN_POINT('Ctrl Pts',(21.503231827314,-11.8204901071103,0.00922720623917468));
#93234=CARTESIAN_POINT('Ctrl Pts',(21.2741540024461,-11.8356971493868,0.00287527591883714));
#93235=CARTESIAN_POINT('Ctrl Pts',(21.1398060819373,-11.833007170968,-0.000891661286779711));
#93236=CARTESIAN_POINT('Ctrl Pts',(20.8648819597256,-11.7401403524706,-0.00891401040353155));
#93237=CARTESIAN_POINT('Ctrl Pts',(20.7523786699402,-11.6759522630052,-0.012290951791703));
#93238=CARTESIAN_POINT('Ctrl Pts',(20.6563591733144,-11.5926712737699,-0.015275484992302));
#93239=CARTESIAN_POINT('',(20.3193037808912,-10.8848592494362,-0.0272277890842044));
#93240=CARTESIAN_POINT('Ctrl Pts',(20.6563591733144,-11.5926712737699,-0.0152754849923009));
#93241=CARTESIAN_POINT('Ctrl Pts',(20.6055977297694,-11.5486441398856,-0.0168532813658944));
#93242=CARTESIAN_POINT('Ctrl Pts',(20.5595669862461,-11.4992460137549,-0.0183180703571777));
#93243=CARTESIAN_POINT('Ctrl Pts',(20.4783995888503,-11.3921384623027,-0.020972833860049));
#93244=CARTESIAN_POINT('Ctrl Pts',(20.4432698252404,-11.3344418887259,-0.0221625695045156));
#93245=CARTESIAN_POINT('Ctrl Pts',(20.3852853252821,-11.2131046998991,-0.0242201017929761));
#93246=CARTESIAN_POINT('Ctrl Pts',(20.3624460868063,-11.1494529184308,-0.0250875051257663));
#93247=CARTESIAN_POINT('Ctrl Pts',(20.3305045689841,-11.0185761815986,-0.0264509701549973));
#93248=CARTESIAN_POINT('Ctrl Pts',(20.3215498650961,-10.9516061699761,-0.0269419887804196));
#93249=CARTESIAN_POINT('Ctrl Pts',(20.3193957862769,-10.8845984096372,-0.0272429516870437));
#93250=CARTESIAN_POINT('',(20.3193161062581,-10.8205589424572,-0.0274550152749159));
#93251=CARTESIAN_POINT('Ctrl Pts',(20.3182662561622,-10.8845986717901,-0.0272745400228147));
#93252=CARTESIAN_POINT('Ctrl Pts',(20.3186047499116,-10.8739814510219,-0.0273032150225033));
#93253=CARTESIAN_POINT('Ctrl Pts',(20.318769563458,-10.8633587412999,-0.0273367670103365));
#93254=CARTESIAN_POINT('Ctrl Pts',(20.3187534786035,-10.8421008046921,-0.0274135843898352));
#93255=CARTESIAN_POINT('Ctrl Pts',(20.3185721644116,-10.8314655952278,-0.0274568613472546));
#93256=CARTESIAN_POINT('Ctrl Pts',(20.3182184169768,-10.8208361620798,-0.0275049399497529));
#93257=CARTESIAN_POINT('',(20.8715427754356,-9.97121102350762,-0.0150824746661654));
#93258=CARTESIAN_POINT('Ctrl Pts',(20.3193928792644,-10.8208352952865,-0.02747209717959));
#93259=CARTESIAN_POINT('Ctrl Pts',(20.3222338376522,-10.7320725931465,-0.0277115181605737));
#93260=CARTESIAN_POINT('Ctrl Pts',(20.3369462701113,-10.6435913145696,-0.0276179216934669));
#93261=CARTESIAN_POINT('Ctrl Pts',(20.3900860096127,-10.4733016174146,-0.0267435292273411));
#93262=CARTESIAN_POINT('Ctrl Pts',(20.428288215811,-10.3933182142733,-0.0259624723348962));
#93263=CARTESIAN_POINT('Ctrl Pts',(20.5260865493615,-10.244975468023,-0.0237602817105972));
#93264=CARTESIAN_POINT('Ctrl Pts',(20.5849926040816,-10.177509639553,-0.0223552371780158));
#93265=CARTESIAN_POINT('Ctrl Pts',(20.717898292447,-10.060226299178,-0.0190596296319128));
#93266=CARTESIAN_POINT('Ctrl Pts',(20.7920498117973,-10.0102371102918,-0.0171654356066794));
#93267=CARTESIAN_POINT('Ctrl Pts',(20.8715427754356,-9.97121102350762,-0.0150824746661655));
#93268=CARTESIAN_POINT('',(21.8012598463038,-10.0131352633455,0.0110692926695165));
#93269=CARTESIAN_POINT('Ctrl Pts',(20.8715427754356,-9.97121102350762,-0.0150824746661655));
#93270=CARTESIAN_POINT('Ctrl Pts',(20.9442163306386,-9.93553284090563,-0.0131782032694574));
#93271=CARTESIAN_POINT('Ctrl Pts',(21.0203053921159,-9.90953391310775,-0.0111436392942924));
#93272=CARTESIAN_POINT('Ctrl Pts',(21.1794653443307,-9.87759783181623,-0.0068071819094258));
#93273=CARTESIAN_POINT('Ctrl Pts',(21.2608328138172,-9.87179676321389,-0.00455243876800186));
#93274=CARTESIAN_POINT('Ctrl Pts',(21.4223470658279,-9.87962131412445,-7.30220672824389E-6));
#93275=CARTESIAN_POINT('Ctrl Pts',(21.5026568601935,-9.89321709277015,0.00228754292219898));
#93276=CARTESIAN_POINT('Ctrl Pts',(21.6574749417698,-9.93919782733929,0.00678248263126461));
#93277=CARTESIAN_POINT('Ctrl Pts',(21.7320415886282,-9.97158827955724,0.00898422908565387));
#93278=CARTESIAN_POINT('Ctrl Pts',(21.8012598463038,-10.0131352633455,0.0110692926695161));
#93279=CARTESIAN_POINT('Ctrl Pts',(21.8012598463038,-10.0131352633455,0.0110692926695162));
#93280=CARTESIAN_POINT('Ctrl Pts',(21.8443447378487,-10.0389961756343,0.0123671401073386));
#93281=CARTESIAN_POINT('Ctrl Pts',(21.885392900488,-10.0682342167638,0.013620158954269));
#93282=CARTESIAN_POINT('Ctrl Pts',(21.9625903176812,-10.1326420227271,0.0160104994198505));
#93283=CARTESIAN_POINT('Ctrl Pts',(21.9987394741801,-10.1678180480274,0.0171478407864812));
#93284=CARTESIAN_POINT('Ctrl Pts',(22.032,-10.2055351096819,0.0182135250455451));
#93285=CARTESIAN_POINT('Origin',(0.,0.,0.));
#93286=CARTESIAN_POINT('',(-4.16932807723036E-10,11.5001144173584,0.0228642038285899));
#93287=CARTESIAN_POINT('',(5.58994029708336E-16,10.205522161444,0.0182134784999908));
#93288=CARTESIAN_POINT('Ctrl Pts',(3.15981143696682E-18,11.5001144184625,
0.0228642038676663));
#93289=CARTESIAN_POINT('Ctrl Pts',(3.15981143696682E-18,11.4666648155453,
0.967921600731115));
#93290=CARTESIAN_POINT('Ctrl Pts',(-1.8863341238837E-12,11.3189678591532,
1.90385824366225));
#93291=CARTESIAN_POINT('Ctrl Pts',(-1.88634172183575E-12,10.8311683388227,
3.54908849500464));
#93292=CARTESIAN_POINT('Ctrl Pts',(-4.24723149583475E-18,10.5332036884033,
4.26226166170117));
#93293=CARTESIAN_POINT('Ctrl Pts',(7.68212098176784E-18,9.47876554604743,
6.15082285610065));
#93294=CARTESIAN_POINT('Ctrl Pts',(-3.46944695195361E-16,8.6951852496647,
6.96624905203417));
#93295=CARTESIAN_POINT('Ctrl Pts',(-3.46944695195361E-16,8.01684087521194,
7.5287776435044));
#93296=CARTESIAN_POINT('Ctrl Pts',(7.62904918881266E-13,7.85893173523043,
7.63486304190703));
#93297=CARTESIAN_POINT('Ctrl Pts',(7.62905461193962E-13,7.73987625544612,
7.68416881913137));
#93298=CARTESIAN_POINT('Ctrl Pts',(-3.02327607393238E-13,7.71568897779549,
7.69225569369772));
#93299=CARTESIAN_POINT('Ctrl Pts',(-3.02327607393238E-13,7.68852262290096,
7.6939848370806));
#93300=CARTESIAN_POINT('Ctrl Pts',(-7.80625564189563E-16,7.68119863204128,
7.69369346751344));
#93301=CARTESIAN_POINT('Ctrl Pts',(-7.80625564189563E-16,7.67039722237102,
7.69059423969854));
#93302=CARTESIAN_POINT('Ctrl Pts',(-5.20417042793042E-17,7.66649558212329,
7.6887691875303));
#93303=CARTESIAN_POINT('Ctrl Pts',(-5.20417042793042E-17,7.66017498071618,
7.68376907703856));
#93304=CARTESIAN_POINT('Ctrl Pts',(3.46992765880931E-17,7.65781392986216,
7.68095885930986));
#93305=CARTESIAN_POINT('Ctrl Pts',(3.46888586034366E-17,7.65382955269162,
7.67390838917976));
#93306=CARTESIAN_POINT('Ctrl Pts',(5.20417042793042E-17,7.65250629254514,
7.6697025383618));
#93307=CARTESIAN_POINT('Ctrl Pts',(5.20417042793042E-17,7.65042516861425,
7.65804982966815));
#93308=CARTESIAN_POINT('Ctrl Pts',(-1.73472347597681E-17,7.65068602749646,
7.65006360430989));
#93309=CARTESIAN_POINT('Ctrl Pts',(-1.73472347597681E-17,7.65369059736511,
7.62507165521352));
#93310=CARTESIAN_POINT('Ctrl Pts',(2.60208521396521E-17,7.66004240645279,
7.60490404284757));
#93311=CARTESIAN_POINT('Ctrl Pts',(2.60208521396521E-17,7.69041651575825,
7.52681063325573));
#93312=CARTESIAN_POINT('Ctrl Pts',(-8.78203759713259E-17,7.73535299370069,
7.44659886752905));
#93313=CARTESIAN_POINT('Ctrl Pts',(-8.78203759713259E-17,8.06204860091466,
6.91667103262996));
#93314=CARTESIAN_POINT('Ctrl Pts',(-3.59719505845404E-13,8.6362158993291,
6.13221168027708));
#93315=CARTESIAN_POINT('Ctrl Pts',(-3.59707701754705E-13,9.47953422855764,
4.3392821160567));
#93316=CARTESIAN_POINT('Ctrl Pts',(7.94902241816546E-14,9.73203279797478,
3.62981596955891));
#93317=CARTESIAN_POINT('Ctrl Pts',(7.94981390428919E-14,10.1364001920077,
1.94730306292097));
#93318=CARTESIAN_POINT('Ctrl Pts',(9.43168451234247E-18,10.2327414932924,
0.987187282335549));
#93319=CARTESIAN_POINT('Ctrl Pts',(9.43168451234247E-18,10.205522161444,
0.018213478499991));
#93320=CARTESIAN_POINT('',(0.,5.42639624653295,0.00104482830329189));
#93321=CARTESIAN_POINT('Origin',(0.7344,10.8528,5.18225781656585E-18));
#93322=CARTESIAN_POINT('',(1.37078399030106,11.5968559808931,-0.0151246218382906));
#93323=CARTESIAN_POINT('Ctrl Pts',(1.37078399030106,11.5968559808931,-0.0151246218382906));
#93324=CARTESIAN_POINT('Ctrl Pts',(1.27515758559223,11.6787046729424,-0.0121562275697988));
#93325=CARTESIAN_POINT('Ctrl Pts',(1.1634760436845,11.7417288632361,-0.00880644902523928));
#93326=CARTESIAN_POINT('Ctrl Pts',(0.88822355641489,11.8338390991337,-0.000777634600949455));
#93327=CARTESIAN_POINT('Ctrl Pts',(0.753591200162323,11.8356484498897,0.00299409374586479));
#93328=CARTESIAN_POINT('Ctrl Pts',(0.536934457303539,11.8205287432007,0.00899896059682586));
#93329=CARTESIAN_POINT('Ctrl Pts',(0.412342432885092,11.7863075085859,0.0123604564058159));
#93330=CARTESIAN_POINT('Ctrl Pts',(0.21382646341409,11.6872334852206,0.0175563853606194));
#93331=CARTESIAN_POINT('Ctrl Pts',(0.103404433621971,11.6177861304089,0.0203950453979665));
#93332=CARTESIAN_POINT('Ctrl Pts',(-7.31578044671499E-10,11.5001144176338,
0.0228642037764085));
#93333=CARTESIAN_POINT('',(1.71367396487917,10.884828376917,-0.0272688936357386));
#93334=CARTESIAN_POINT('Ctrl Pts',(1.71323760973584,10.884757371723,-0.0272600945708667));
#93335=CARTESIAN_POINT('Ctrl Pts',(1.71095380282436,10.9522588475904,-0.0269537299596494));
#93336=CARTESIAN_POINT('Ctrl Pts',(1.70125599859845,11.0194421721267,-0.0264411629320617));
#93337=CARTESIAN_POINT('Ctrl Pts',(1.66832024614853,11.150863447781,-0.0250479361935688));
#93338=CARTESIAN_POINT('Ctrl Pts',(1.64499600892519,11.2151054272743,-0.0241648487888341));
#93339=CARTESIAN_POINT('Ctrl Pts',(1.58618668503831,11.3373729668203,-0.0220809066579494));
#93340=CARTESIAN_POINT('Ctrl Pts',(1.5506912354297,11.3955174606547,-0.0208793348533259));
#93341=CARTESIAN_POINT('Ctrl Pts',(1.46868851153284,11.5032546695393,-0.0181989480045432));
#93342=CARTESIAN_POINT('Ctrl Pts',(1.42218772068958,11.552858424867,-0.0167202746198522));
#93343=CARTESIAN_POINT('Ctrl Pts',(1.37078399030106,11.5968559808931,-0.0151246218382906));
#93344=CARTESIAN_POINT('',(1.71371885186958,10.8205931966853,-0.0274987012850932));
#93345=CARTESIAN_POINT('Ctrl Pts',(1.71367158232227,10.8847577695798,-0.0272722299410126));
#93346=CARTESIAN_POINT('Ctrl Pts',(1.71332804833583,10.8740884873295,-0.027300951008168));
#93347=CARTESIAN_POINT('Ctrl Pts',(1.71316046545629,10.8634136017891,-0.0273346129839613));
#93348=CARTESIAN_POINT('Ctrl Pts',(1.71317536219933,10.8420544454392,-0.0274117607591387));
#93349=CARTESIAN_POINT('Ctrl Pts',(1.71335815656387,10.831370214279,-0.0274552552183969));
#93350=CARTESIAN_POINT('Ctrl Pts',(1.71371536404704,10.8206918479203,-0.0275036063755117));
#93351=CARTESIAN_POINT('',(1.70529432647543,10.72808525788,-0.0276007795948528));
#93352=CARTESIAN_POINT('Ctrl Pts',(1.70529432647543,10.72808525788,-0.0276007795948528));
#93353=CARTESIAN_POINT('Ctrl Pts',(1.70735454658141,10.7434173025721,-0.0276033180225536));
#93354=CARTESIAN_POINT('Ctrl Pts',(1.70904613121517,10.7587984274458,-0.0275953706002022));
#93355=CARTESIAN_POINT('Ctrl Pts',(1.71168063254266,10.7896797461349,-0.0275581102060633));
#93356=CARTESIAN_POINT('Ctrl Pts',(1.71262079348754,10.8051786491146,-0.0275287248021881));
#93357=CARTESIAN_POINT('Ctrl Pts',(1.71317372525099,10.8206923858305,-0.0274884565705673));
#93358=CARTESIAN_POINT('',(0.236247419988345,10.0098541173715,0.0109034851016902));
#93359=CARTESIAN_POINT('Ctrl Pts',(0.236247419988345,10.0098541173715,0.0109034851016902));
#93360=CARTESIAN_POINT('Ctrl Pts',(0.30606056814941,9.96856972869477,0.00880272772994621));
#93361=CARTESIAN_POINT('Ctrl Pts',(0.381103068719988,9.93630945446466,0.00658814085987126));
#93362=CARTESIAN_POINT('Ctrl Pts',(0.536789596238908,9.89086391615539,0.00207083621442976));
#93363=CARTESIAN_POINT('Ctrl Pts',(0.617427443273441,9.87767541233786,-0.000231720367397251));
#93364=CARTESIAN_POINT('Ctrl Pts',(0.72992935704866,9.87330259655987,-0.00339374139128517));
#93365=CARTESIAN_POINT('Ctrl Pts',(0.761467622684855,9.87359480108384,-0.00427471421096523));
#93366=CARTESIAN_POINT('Ctrl Pts',(0.942427970193946,9.88416684405416,-0.00929760631769659));
#93367=CARTESIAN_POINT('Ctrl Pts',(1.0684186552677,9.92647143273604,-0.0126691792673942));
#93368=CARTESIAN_POINT('Ctrl Pts',(1.26139994575964,10.0202638957781,-0.0177292948903863));
#93369=CARTESIAN_POINT('Ctrl Pts',(1.36839556444661,10.0913712265771,-0.0204661660330931));
#93370=CARTESIAN_POINT('Ctrl Pts',(1.52969665304764,10.2744047761715,-0.0243196977313969));
#93371=CARTESIAN_POINT('Ctrl Pts',(1.58325884460451,10.3578038615545,-0.0255180527928208));
#93372=CARTESIAN_POINT('Ctrl Pts',(1.66446908023142,10.5360177894713,-0.0271490183867767));
#93373=CARTESIAN_POINT('Ctrl Pts',(1.69226021046953,10.6310860835949,-0.0275847200675102));
#93374=CARTESIAN_POINT('Ctrl Pts',(1.70529432647543,10.72808525788,-0.0276007795948528));
#93375=CARTESIAN_POINT('Ctrl Pts',(1.2490009027033E-15,10.205522161444,
0.0182134784999908));
#93376=CARTESIAN_POINT('Ctrl Pts',(0.033968553860442,10.1670088719863,0.0171251326194028));
#93377=CARTESIAN_POINT('Ctrl Pts',(0.0709495090590134,10.1311471009747,
0.0159620650678615));
#93378=CARTESIAN_POINT('Ctrl Pts',(0.150002720154503,10.0656333354706,0.0135158510258428));
#93379=CARTESIAN_POINT('Ctrl Pts',(0.192074236372062,10.035976172164,0.0122327066532125));
#93380=CARTESIAN_POINT('Ctrl Pts',(0.236247419988344,10.0098541173715,0.0109034851016902));
#93381=CARTESIAN_POINT('Ctrl Pts',(1.30897478982197,11.3504630390858,-2.50498148137219));
#93382=CARTESIAN_POINT('Ctrl Pts',(1.38386448873185,11.8926837577678,0.261422345341801));
#93383=CARTESIAN_POINT('Ctrl Pts',(1.51312640105233,11.2420912813384,4.85222885469421));
#93384=CARTESIAN_POINT('Ctrl Pts',(1.69450156347185,6.96747103308611,9.80841498077292));
#93385=CARTESIAN_POINT('Ctrl Pts',(1.85302105907588,1.69666347680562,11.8855184550591));
#93386=CARTESIAN_POINT('Ctrl Pts',(2.01132807879988,-3.94947939190903,11.3373251838206));
#93387=CARTESIAN_POINT('Ctrl Pts',(2.16948245088834,-8.70317504738577,8.24890086458565));
#93388=CARTESIAN_POINT('Ctrl Pts',(2.32764998417709,-11.5100452091871,3.33273214547989));
#93389=CARTESIAN_POINT('Ctrl Pts',(2.48532551435814,-11.7452138138953,-2.32118714406843));
#93390=CARTESIAN_POINT('Ctrl Pts',(2.64369910587744,-9.36167700277716,-7.44664390195442));
#93391=CARTESIAN_POINT('Ctrl Pts',(2.80006441572129,-4.89466326032176,-10.9038432854129));
#93392=CARTESIAN_POINT('Ctrl Pts',(2.96038504525873,0.655585150116943,-11.9232041725978));
#93393=CARTESIAN_POINT('Ctrl Pts',(3.11196817314966,6.05030776943863,-10.2836091806122));
#93394=CARTESIAN_POINT('Ctrl Pts',(3.28097474479473,10.0860135530921,-6.35229193778149));
#93395=CARTESIAN_POINT('Ctrl Pts',(3.41362143929016,11.8666268602166,-1.01359022713016));
#93396=CARTESIAN_POINT('Ctrl Pts',(3.62798652276341,10.9978448176373,4.53108407232712));
#93397=CARTESIAN_POINT('Ctrl Pts',(3.83136289374924,7.68047060934463,9.06465386067078));
#93398=CARTESIAN_POINT('Ctrl Pts',(4.05934605751117,2.10302841524976,11.8468921137569));
#93399=CARTESIAN_POINT('Ctrl Pts',(4.30893325794595,-4.85958883366253,11.1951873452828));
#93400=CARTESIAN_POINT('Ctrl Pts',(4.58111469907456,-10.5439802324246,6.10854505812171));
#93401=CARTESIAN_POINT('Ctrl Pts',(4.85266833009858,-12.0838233435126,-1.33981903278729));
#93402=CARTESIAN_POINT('Ctrl Pts',(5.12382899664887,-8.91442850896208,-8.23976580227665));
#93403=CARTESIAN_POINT('Ctrl Pts',(5.39447422289012,-2.27332112649084,-11.9037038363946));
#93404=CARTESIAN_POINT('Ctrl Pts',(5.63462866738158,4.38930278932178,-11.0139596956066));
#93405=CARTESIAN_POINT('Ctrl Pts',(5.84443876548001,8.89587552847269,-7.49634408243274));
#93406=CARTESIAN_POINT('Ctrl Pts',(6.02405598838773,11.1785196113352,-3.17466519093072));
#93407=CARTESIAN_POINT('Ctrl Pts',(6.23334858135947,11.5367789170952,2.51834492771313));
#93408=CARTESIAN_POINT('Ctrl Pts',(6.47216536153378,8.52591928036444,8.48613021692799));
#93409=CARTESIAN_POINT('Ctrl Pts',(6.74032351979013,1.81378966884307,11.8672295275066));
#93410=CARTESIAN_POINT('Ctrl Pts',(7.0079645542307,-5.57435948674926,10.605462370046));
#93411=CARTESIAN_POINT('Ctrl Pts',(7.27508531570782,-10.7625364349888,5.21331503061486));
#93412=CARTESIAN_POINT('Ctrl Pts',(7.5416794938748,-11.7311710285706,-2.19176367291935));
#93413=CARTESIAN_POINT('Ctrl Pts',(7.8077437693088,-8.1229758038346,-8.7108511612512));
#93414=CARTESIAN_POINT('Ctrl Pts',(8.07327440627059,-1.35788077218519,-11.810228596338));
#93415=CARTESIAN_POINT('Ctrl Pts',(8.3088229880755,5.09482672424843,-10.4525999052638));
#93416=CARTESIAN_POINT('Ctrl Pts',(8.51457805138463,9.24392923696522,-6.68374543262319));
#93417=CARTESIAN_POINT('Ctrl Pts',(8.69069787800009,11.1618634053179,-2.28846725754921));
#93418=CARTESIAN_POINT('Ctrl Pts',(8.86657573197387,11.0975692878018,2.49903950200297));
#93419=CARTESIAN_POINT('Ctrl Pts',(9.06172558105388,8.85449784911366,7.32026089744886));
#93420=CARTESIAN_POINT('Ctrl Pts',(9.23707598578613,4.95803577700564,10.2175308052139));
#93421=CARTESIAN_POINT('Ctrl Pts',(9.41218197984377,0.353935032346256,11.2200746322382));
#93422=CARTESIAN_POINT('Ctrl Pts',(9.56765013607029,-3.83951280272671,10.6454205565639));
#93423=CARTESIAN_POINT('Ctrl Pts',(9.74230644009734,-7.8631980922651,8.10968127001615));
#93424=CARTESIAN_POINT('Ctrl Pts',(9.94578506400173,-10.9327846091029,3.49606033646916));
#93425=CARTESIAN_POINT('Ctrl Pts',(10.1779215386847,-11.3026255166413,-2.99474193137141));
#93426=CARTESIAN_POINT('Ctrl Pts',(10.3950862741132,-7.96186222719694,-8.07924641994259));
#93427=CARTESIAN_POINT('Ctrl Pts',(10.5685399649705,-3.88496594820853,-10.3692560271556));
#93428=CARTESIAN_POINT('Ctrl Pts',(10.7418080726905,0.698226275935602,-11.2916890703984));
#93429=CARTESIAN_POINT('Ctrl Pts',(10.9292134877369,5.73545411152713,-9.83539908865925));
#93430=CARTESIAN_POINT('Ctrl Pts',(11.1306736564829,9.51259625505713,-5.8530435057731));
#93431=CARTESIAN_POINT('Ctrl Pts',(11.303106225153,11.0641086404226,-1.42127934142605));
#93432=CARTESIAN_POINT('Ctrl Pts',(11.4561595909811,10.6960254211943,2.72874079862435));
#93433=CARTESIAN_POINT('Ctrl Pts',(11.6281385166885,8.7278532497703,6.91733533563937));
#93434=CARTESIAN_POINT('Ctrl Pts',(11.7998702409163,5.11081927142178,10.0033545553924));
#93435=CARTESIAN_POINT('Ctrl Pts',(11.990363183906,0.0338904688058861,11.0876495659952));
#93436=CARTESIAN_POINT('Ctrl Pts',(12.1615603432201,-4.52246394700098,10.1101748948404));
#93437=CARTESIAN_POINT('Ctrl Pts',(12.3325112871038,-8.26592723037474,7.34305430882504));
#93438=CARTESIAN_POINT('Ctrl Pts',(12.5316675984782,-10.9260818914473,2.61447385314119));
#93439=CARTESIAN_POINT('Ctrl Pts',(12.7588657234676,-10.8119033324059,-3.74505536412208));
#93440=CARTESIAN_POINT('Ctrl Pts',(13.0139143775298,-6.45822803221135,-9.41359275769931));
#93441=CARTESIAN_POINT('Ctrl Pts',(13.2684156739832,0.391051711522962,-11.3845366962931));
#93442=CARTESIAN_POINT('Ctrl Pts',(13.5223720121342,7.06058079564972,-8.90911861064873));
#93443=CARTESIAN_POINT('Ctrl Pts',(13.7757872242173,10.9472554116764,-2.96870788326275));
#93444=CARTESIAN_POINT('Ctrl Pts',(14.0286634776398,10.5494242808733,4.10178934251099));
#93445=CARTESIAN_POINT('Ctrl Pts',(14.2810050361338,6.0378241672127,9.54734246153401));
#93446=CARTESIAN_POINT('Ctrl Pts',(14.5048367771901,-0.0457796910363487,
11.0484597831507));
#93447=CARTESIAN_POINT('Ctrl Pts',(14.7003478024558,-5.15247455494966,9.53528368421946));
#93448=CARTESIAN_POINT('Ctrl Pts',(14.8676959182846,-8.60689881955561,6.56596087686259));
#93449=CARTESIAN_POINT('Ctrl Pts',(15.0348124912905,-10.5304401021696,2.44009830321553));
#93450=CARTESIAN_POINT('Ctrl Pts',(15.2016992363267,-10.5889896031044,-2.10339644174452));
#93451=CARTESIAN_POINT('Ctrl Pts',(15.3683571298684,-8.77365701916214,-6.26387195102793));
#93452=CARTESIAN_POINT('Ctrl Pts',(15.5347882691619,-5.41443881745476,-9.30488661898314));
#93453=CARTESIAN_POINT('Ctrl Pts',(15.7009938729794,-1.10506303701437,-10.6939689442717));
#93454=CARTESIAN_POINT('Ctrl Pts',(15.8669756154884,3.38421159098208,-10.1885736990089));
#93455=CARTESIAN_POINT('Ctrl Pts',(16.0603620719526,7.91915265148676,-7.50326322098924));
#93456=CARTESIAN_POINT('Ctrl Pts',(16.239636841349,10.346417595362,-3.11521415876683));
#93457=CARTESIAN_POINT('Ctrl Pts',(16.4048767410778,10.4634131688112,1.34239684552686));
#93458=CARTESIAN_POINT('Ctrl Pts',(16.5493197829215,9.35599017071544,5.07525108848545));
#93459=CARTESIAN_POINT('Ctrl Pts',(16.7141963176832,6.49237344325913,8.56862170466309));
#93460=CARTESIAN_POINT('Ctrl Pts',(16.8994136289952,1.83069526121731,10.5775323405323));
#93461=CARTESIAN_POINT('Ctrl Pts',(17.0843650545091,-3.22035309403346,10.2223670343401));
#93462=CARTESIAN_POINT('Ctrl Pts',(17.2895747157592,-8.03234514251166,7.30506860791021));
#93463=CARTESIAN_POINT('Ctrl Pts',(17.5149342113487,-10.8733400024111,1.67419416675553));
#93464=CARTESIAN_POINT('Ctrl Pts',(17.7603281370208,-9.73044464288831,-5.10667512772299));
#93465=CARTESIAN_POINT('Ctrl Pts',(17.9848608346678,-5.19699805192515,-9.46388837584811));
#93466=CARTESIAN_POINT('Ctrl Pts',(18.1886661451407,0.265632069066906,-10.6262404306785));
#93467=CARTESIAN_POINT('Ctrl Pts',(18.3718394205153,5.10633304707169,-9.30876868720459));
#93468=CARTESIAN_POINT('Ctrl Pts',(18.5547939179018,8.79802794991572,-5.91765010486416));
#93469=CARTESIAN_POINT('Ctrl Pts',(18.7374627363208,10.5191177631719,-1.2179863155584));
#93470=CARTESIAN_POINT('Ctrl Pts',(18.9200143211695,9.89212967677138,3.74154082705846));
#93471=CARTESIAN_POINT('Ctrl Pts',(19.1020930075487,7.06236441759157,7.85504180831257));
#93472=CARTESIAN_POINT('Ctrl Pts',(19.2844116650314,2.66565483537424,10.2072618947442));
#93473=CARTESIAN_POINT('Ctrl Pts',(19.4657299037891,-2.31400728008752,10.2809442197002));
#93474=CARTESIAN_POINT('Ctrl Pts',(19.648066469154,-6.76693935292665,8.0595630932652));
#93475=CARTESIAN_POINT('Ctrl Pts',(19.8276165222382,-9.70035629775437,4.05485210714321));
#93476=CARTESIAN_POINT('Ctrl Pts',(20.0175251180967,-10.4657896755927,-0.857742150482306));
#93477=CARTESIAN_POINT('Ctrl Pts',(20.1343530166592,-8.89702629841736,-5.56249800699203));
#93478=CARTESIAN_POINT('Ctrl Pts',(20.2829990256603,-5.34622937894769,-9.01726442891408));
#93479=CARTESIAN_POINT('Ctrl Pts',(20.416084338308,-0.60971988323014,-10.4571484597653));
#93480=CARTESIAN_POINT('Ctrl Pts',(20.5566179423485,4.25527008514754,-9.56204556806775));
#93481=CARTESIAN_POINT('Ctrl Pts',(20.6934363685739,8.16330759088052,-6.53628165676501));
#93482=CARTESIAN_POINT('Ctrl Pts',(20.8317979438454,10.2448413935788,-2.05829576335044));
#93483=CARTESIAN_POINT('Ctrl Pts',(20.9693138595582,10.0386345642595,2.87335852336565));
#93484=CARTESIAN_POINT('Ctrl Pts',(21.1070527977384,7.59382441058238,7.15294197070558));
#93485=CARTESIAN_POINT('Ctrl Pts',(21.2445261479924,3.46011245261836,9.83939395559342));
#93486=CARTESIAN_POINT('Ctrl Pts',(21.3820140102286,-1.44110991972201,10.3106942348191));
#93487=CARTESIAN_POINT('Ctrl Pts',(21.5192385743442,-6.00937269882226,8.51719726799948));
#93488=CARTESIAN_POINT('Ctrl Pts',(21.6765786177924,-9.70830673657193,4.21254883161156));
#93489=CARTESIAN_POINT('Ctrl Pts',(21.7873558901873,-10.268703591987,0.279124218596134));
#93490=CARTESIAN_POINT('Ctrl Pts',(21.8541003835446,-9.80111969116135,-2.18436427930479));
#93491=CARTESIAN_POINT('Ctrl Pts',(1.18974746786317,11.4517922664652,-2.52090132956655));
#93492=CARTESIAN_POINT('Ctrl Pts',(1.26518414667326,11.9988181450597,0.265780471340153));
#93493=CARTESIAN_POINT('Ctrl Pts',(1.39565853232302,11.3425692650812,4.89981968805774));
#93494=CARTESIAN_POINT('Ctrl Pts',(1.57866787392373,7.02897372769986,9.90043289144675));
#93495=CARTESIAN_POINT('Ctrl Pts',(1.73867035820078,1.70925650077172,11.9974400786412));
#93496=CARTESIAN_POINT('Ctrl Pts',(1.89846534925839,-3.99014183964466,11.4439163937075));
#93497=CARTESIAN_POINT('Ctrl Pts',(2.05813461856846,-8.78937060554582,8.32616088827542));
#93498=CARTESIAN_POINT('Ctrl Pts',(2.2178372191676,-11.6235870025466,3.36222965129985));
#93499=CARTESIAN_POINT('Ctrl Pts',(2.37706510609572,-11.8611623899059,-2.3473285393946));
#93500=CARTESIAN_POINT('Ctrl Pts',(2.53702005955193,-9.4538997106099,-7.52403366560333));
#93501=CARTESIAN_POINT('Ctrl Pts',(2.69496675943479,-4.94174608981969,-11.0162600707292));
#93502=CARTESIAN_POINT('Ctrl Pts',(2.85693169535897,0.665427965998577,-12.046217394457));
#93503=CARTESIAN_POINT('Ctrl Pts',(3.01008843650435,6.11617669158266,-10.3895731296628));
#93504=CARTESIAN_POINT('Ctrl Pts',(3.18087145496237,10.1944375660391,-6.41713549186393));
#93505=CARTESIAN_POINT('Ctrl Pts',(3.31492761737946,11.9939986422514,-1.02153441070433));
#93506=CARTESIAN_POINT('Ctrl Pts',(3.53165396391817,11.1159703877652,4.58442295205435));
#93507=CARTESIAN_POINT('Ctrl Pts',(3.73722553710061,7.76246260128082,9.16681927618251));
#93508=CARTESIAN_POINT('Ctrl Pts',(3.96775616233569,2.12305632832777,11.980505907057));
#93509=CARTESIAN_POINT('Ctrl Pts',(4.22015087915041,-4.918109620414,11.3214168981758));
#93510=CARTESIAN_POINT('Ctrl Pts',(4.49546369841027,-10.6680280311112,6.1766295866806));
#93511=CARTESIAN_POINT('Ctrl Pts',(4.77019090889438,-12.2260930284393,-1.35884290056484));
#93512=CARTESIAN_POINT('Ctrl Pts',(5.04457454319731,-9.01924683266811,-8.34087088097074));
#93513=CARTESIAN_POINT('Ctrl Pts',(5.31848644889902,-2.29805924217776,-12.049253587911));
#93514=CARTESIAN_POINT('Ctrl Pts',(5.56158289892602,4.4462322167097,-11.1487877087618));
#93515=CARTESIAN_POINT('Ctrl Pts',(5.77399527205737,9.00875437884592,-7.58759241958776));
#93516=CARTESIAN_POINT('Ctrl Pts',(5.95586064806108,11.3200193718728,-3.21184415601971));
#93517=CARTESIAN_POINT('Ctrl Pts',(6.167795918538,11.6828725325942,2.55304786169007));
#93518=CARTESIAN_POINT('Ctrl Pts',(6.40966019967681,8.63373216818036,8.5970722721158));
#93519=CARTESIAN_POINT('Ctrl Pts',(6.68128293317983,1.83495642429353,12.0220246559432));
#93520=CARTESIAN_POINT('Ctrl Pts',(6.95242181181914,-5.64979323947622,10.7439345769541));
#93521=CARTESIAN_POINT('Ctrl Pts',(7.22307251307632,-10.9066557638468,5.28064151031707));
#93522=CARTESIAN_POINT('Ctrl Pts',(7.49322591235527,-11.8883788942064,-2.22329037953124));
#93523=CARTESIAN_POINT('Ctrl Pts',(7.762877003322,-8.23166841266443,-8.83034127715893));
#93524=CARTESIAN_POINT('Ctrl Pts',(8.03202026329645,-1.37458546094406,-11.9720187625362));
#93525=CARTESIAN_POINT('Ctrl Pts',(8.27080031567461,5.1666841103954,-10.5958720135022));
#93526=CARTESIAN_POINT('Ctrl Pts',(8.47939743040809,9.37312928197355,-6.77498911346165));
#93527=CARTESIAN_POINT('Ctrl Pts',(8.65796190964001,11.3177170749869,-2.3187107460461));
#93528=CARTESIAN_POINT('Ctrl Pts',(8.83629282307935,11.2525571600563,2.53557131712909));
#93529=CARTESIAN_POINT('Ctrl Pts',(9.03417691141257,8.97809165929157,7.42435568944228));
#93530=CARTESIAN_POINT('Ctrl Pts',(9.21199612018571,5.02679642075796,10.3624580547133));
#93531=CARTESIAN_POINT('Ctrl Pts',(9.38957733795619,0.35761650699035,11.3791857664677));
#93532=CARTESIAN_POINT('Ctrl Pts',(9.54724976039764,-3.8952913802988,10.7964042010188));
#93533=CARTESIAN_POINT('Ctrl Pts',(9.72439118282002,-7.97624041142031,8.22460440416845));
#93534=CARTESIAN_POINT('Ctrl Pts',(9.93077429626411,-11.0896632215142,3.54514357646063));
#93535=CARTESIAN_POINT('Ctrl Pts',(10.1662370872959,-11.4648622236249,-3.03865513251931));
#93536=CARTESIAN_POINT('Ctrl Pts',(10.3865254314365,-8.07608583722479,-8.19631869413491));
#93537=CARTESIAN_POINT('Ctrl Pts',(10.5624802891134,-3.94040545902368,-10.5193556970742));
#93538=CARTESIAN_POINT('Ctrl Pts',(10.7382506126395,0.708969224933737,-11.4551172204512));
#93539=CARTESIAN_POINT('Ctrl Pts',(10.9283685210332,5.81910754761555,-9.97777463152521));
#93540=CARTESIAN_POINT('Ctrl Pts',(11.1327495067884,9.65101628657111,-5.93769000513916));
#93541=CARTESIAN_POINT('Ctrl Pts',(11.3076849817366,11.2250562811182,-1.44160136579286));
#93542=CARTESIAN_POINT('Ctrl Pts',(11.4629625774418,10.8516272644798,2.76872199953724));
#93543=CARTESIAN_POINT('Ctrl Pts',(11.6374418821889,8.85484247875078,7.01821193605031));
#93544=CARTESIAN_POINT('Ctrl Pts',(11.8116716998053,5.18519912941044,10.1491227347192));
#93545=CARTESIAN_POINT('Ctrl Pts',(12.0049367578346,0.0343959505934401,
11.2491953572123));
#93546=CARTESIAN_POINT('Ctrl Pts',(12.1786245890754,-4.58824344319239,10.2574978750432));
#93547=CARTESIAN_POINT('Ctrl Pts',(12.352062477449,-8.38615633729713,7.45012563881324));
#93548=CARTESIAN_POINT('Ctrl Pts',(12.554113756606,-11.0849733631632,2.65280836007122));
#93549=CARTESIAN_POINT('Ctrl Pts',(12.7846122961941,-10.9691146512919,-3.7990828045243));
#93550=CARTESIAN_POINT('Ctrl Pts',(13.0433583516889,-6.55230109938501,-9.54976360017405));
#93551=CARTESIAN_POINT('Ctrl Pts',(13.3015404849569,0.396035834484766,-11.5491659899366));
#93552=CARTESIAN_POINT('Ctrl Pts',(13.5591589282335,7.16170582651916,-9.03800376659064));
#93553=CARTESIAN_POINT('Ctrl Pts',(13.8162148628397,11.1041565484206,-3.0122242034893));
#93554=CARTESIAN_POINT('Ctrl Pts',(14.0727093835286,10.7005567366767,4.15941404407192));
#93555=CARTESIAN_POINT('Ctrl Pts',(14.3286435930605,6.12466583879098,9.68243478675451));
#93556=CARTESIAN_POINT('Ctrl Pts',(14.5556458025187,-0.0451007091892611,
11.20471923806));
#93557=CARTESIAN_POINT('Ctrl Pts',(14.7539104053305,-5.22370059967178,9.670201548657));
#93558=CARTESIAN_POINT('Ctrl Pts',(14.9236060827809,-8.72655048304717,6.65920792858466));
#93559=CARTESIAN_POINT('Ctrl Pts',(15.0930560971764,-10.6769135579603,2.47573475735213));
#93560=CARTESIAN_POINT('Ctrl Pts',(15.2622606653902,-10.7362380843536,-2.13085705163885));
#93561=CARTESIAN_POINT('Ctrl Pts',(15.4312223228812,-8.89578686497418,-6.34881194318317));
#93562=CARTESIAN_POINT('Ctrl Pts',(15.5999407121251,-5.49038444331317,-9.43157994135716));
#93563=CARTESIAN_POINT('Ctrl Pts',(15.7684173535114,-1.12212996432778,-10.8396028454176));
#93564=CARTESIAN_POINT('Ctrl Pts',(15.9366523292351,3.42807230949616,-10.3273045410418));
#93565=CARTESIAN_POINT('Ctrl Pts',(16.1326467590311,8.02413915422211,-7.60574003322458));
#93566=CARTESIAN_POINT('Ctrl Pts',(16.314321409095,10.4837845689353,-3.1589303196056));
#93567=CARTESIAN_POINT('Ctrl Pts',(16.4817523929375,10.6022981932295,1.35777601683656));
#93568=CARTESIAN_POINT('Ctrl Pts',(16.628100233848,9.48025342044983,5.13984100178697));
#93569=CARTESIAN_POINT('Ctrl Pts',(16.7951358098011,6.5790973516086,8.67890252146067));
#93570=CARTESIAN_POINT('Ctrl Pts',(16.9827558713765,1.85693486775176,10.7137909459705));
#93571=CARTESIAN_POINT('Ctrl Pts',(17.1700831822853,-3.25897596162862,10.3539932205293));
#93572=CARTESIAN_POINT('Ctrl Pts',(17.3779027649741,-8.13209734273167,7.39951611744703));
#93573=CARTESIAN_POINT('Ctrl Pts',(17.6060922224903,-11.0086032355239,1.69787761110265));
#93574=CARTESIAN_POINT('Ctrl Pts',(17.8545207088345,-9.85135526552179,-5.16679810337559));
#93575=CARTESIAN_POINT('Ctrl Pts',(18.0817887133709,-5.26259033002558,-9.57691066568822));
#93576=CARTESIAN_POINT('Ctrl Pts',(18.2880380245083,0.265548580560466,-10.7530867295508));
#93577=CARTESIAN_POINT('Ctrl Pts',(18.4733796814325,5.16350438434969,-9.41993410006301));
#93578=CARTESIAN_POINT('Ctrl Pts',(18.6584701908049,8.89821185951937,-5.98916918444961));
#93579=CARTESIAN_POINT('Ctrl Pts',(18.8432409950164,10.6390066358219,-1.23539709009161));
#93580=CARTESIAN_POINT('Ctrl Pts',(19.0278628981949,10.0048039354509,3.78029736455163));
#93581=CARTESIAN_POINT('Ctrl Pts',(19.2119723825552,7.14338976532434,7.93968275473146));
#93582=CARTESIAN_POINT('Ctrl Pts',(19.3962971146005,2.69833785744414,10.3175199556526));
#93583=CARTESIAN_POINT('Ctrl Pts',(19.579564992325,-2.33502128752636,10.3921141672789));
#93584=CARTESIAN_POINT('Ctrl Pts',(19.7638538077289,-6.83522052429279,8.14659582436836));
#93585=CARTESIAN_POINT('Ctrl Pts',(19.9452412106374,-9.79898956792458,4.10104273626897));
#93586=CARTESIAN_POINT('Ctrl Pts',(20.1371455329409,-10.5721168787306,-0.863355728409352));
#93587=CARTESIAN_POINT('Ctrl Pts',(20.2551462392215,-8.98758519098429,-5.61547760810045));
#93588=CARTESIAN_POINT('Ctrl Pts',(20.4052645664765,-5.40151747470937,-9.1042056824633));
#93589=CARTESIAN_POINT('Ctrl Pts',(20.5396467848151,-0.618870314778679,
-10.5581353506426));
#93590=CARTESIAN_POINT('Ctrl Pts',(20.681528826317,4.29274934883192,-9.65430165578985));
#93591=CARTESIAN_POINT('Ctrl Pts',(20.8196362604007,8.2375272330093,-6.59999125855159));
#93592=CARTESIAN_POINT('Ctrl Pts',(20.9592798997399,10.3382476746094,-2.0804841092725));
#93593=CARTESIAN_POINT('Ctrl Pts',(21.0980466529407,10.1300663649379,2.8959570685733));
#93594=CARTESIAN_POINT('Ctrl Pts',(21.2370151017179,7.66334706916283,7.21373849358107));
#93595=CARTESIAN_POINT('Ctrl Pts',(21.3756941059591,3.49341097342452,9.92347886797355));
#93596=CARTESIAN_POINT('Ctrl Pts',(21.5143584573025,-1.44987922468851,10.3989557782019));
#93597=CARTESIAN_POINT('Ctrl Pts',(21.6527478812955,-6.05651644093992,8.58980440466931));
#93598=CARTESIAN_POINT('Ctrl Pts',(21.8113618981694,-9.78578944726137,4.2505359954563));
#93599=CARTESIAN_POINT('Ctrl Pts',(21.9230775074673,-10.3505739977289,0.283696021016612));
#93600=CARTESIAN_POINT('Ctrl Pts',(21.9902419502383,-9.87925711877443,-2.19539365961811));
#93601=CARTESIAN_POINT('Ctrl Pts',(0.903441628217493,11.5956865362208,-2.54034914141355));
#93602=CARTESIAN_POINT('Ctrl Pts',(0.979658017345533,12.1495390241206,0.275253015337542));
#93603=CARTESIAN_POINT('Ctrl Pts',(1.11185919217728,11.4853157251709,4.97085529600647));
#93604=CARTESIAN_POINT('Ctrl Pts',(1.29722630370222,7.11559218861858,10.03559800166));
#93605=CARTESIAN_POINT('Ctrl Pts',(1.4593901240281,1.72464681668832,12.1616878256515));
#93606=CARTESIAN_POINT('Ctrl Pts',(1.62137479817313,-4.05308567022919,11.6004162607819));
#93607=CARTESIAN_POINT('Ctrl Pts',(1.78329400206896,-8.9199643442394,8.43919520839999));
#93608=CARTESIAN_POINT('Ctrl Pts',(1.94529726649785,-11.7952180436883,3.40376438492117));
#93609=CARTESIAN_POINT('Ctrl Pts',(2.10687154681895,-12.0365246368009,-2.38985096138074));
#93610=CARTESIAN_POINT('Ctrl Pts',(2.26923745269956,-9.59318307000292,-7.64468833195954));
#93611=CARTESIAN_POINT('Ctrl Pts',(2.42961363996627,-5.01176400552785,-11.1907591909536));
#93612=CARTESIAN_POINT('Ctrl Pts',(2.59412589846795,0.683543359587545,-12.2372546878033));
#93613=CARTESIAN_POINT('Ctrl Pts',(2.74973808312862,6.22167787228081,-10.5540021858096));
#93614=CARTESIAN_POINT('Ctrl Pts',(2.92331316951063,10.3669128347436,-6.5171622001184));
#93615=CARTESIAN_POINT('Ctrl Pts',(3.05959909542248,12.1964574224635,-1.03146587853192));
#93616=CARTESIAN_POINT('Ctrl Pts',(3.28013866994355,11.3038043278321,4.67361588913699));
#93617=CARTESIAN_POINT('Ctrl Pts',(3.48921509325285,7.89233189478907,9.33384404675561));
#93618=CARTESIAN_POINT('Ctrl Pts',(3.7238939372982,2.15239269705436,12.1990469837114));
#93619=CARTESIAN_POINT('Ctrl Pts',(3.98088049228753,-5.01739795831119,11.5278737873867));
#93620=CARTESIAN_POINT('Ctrl Pts',(4.26138198908379,-10.8759517203058,6.28713144448326));
#93621=CARTESIAN_POINT('Ctrl Pts',(4.54141217777241,-12.4647033890014,-1.39391008316943));
#93622=CARTESIAN_POINT('Ctrl Pts',(4.82123757322336,-9.19485740050448,-8.51453853976309));
#93623=CARTESIAN_POINT('Ctrl Pts',(5.1007140760936,-2.33739080685041,-12.298841317748));
#93624=CARTESIAN_POINT('Ctrl Pts',(5.34886880731605,4.54729884524234,-11.3801342835202));
#93625=CARTESIAN_POINT('Ctrl Pts',(5.56578483547677,9.20670066674851,-7.74358589277483));
#93626=CARTESIAN_POINT('Ctrl Pts',(5.75156316224047,11.5678259674798,-3.27376473974182));
#93627=CARTESIAN_POINT('Ctrl Pts',(5.96812411478037,11.938803177318,2.61691849448023));
#93628=CARTESIAN_POINT('Ctrl Pts',(6.21535908381347,8.82238390057781,8.79536260171968));
#93629=CARTESIAN_POINT('Ctrl Pts',(6.49313495565504,1.86984596831206,12.298388326641));
#93630=CARTESIAN_POINT('Ctrl Pts',(6.77053350207384,-5.78779554802438,10.9913053328563));
#93631=CARTESIAN_POINT('Ctrl Pts',(7.04754819093855,-11.1686313246679,5.39990857726151));
#93632=CARTESIAN_POINT('Ctrl Pts',(7.324164919137,-12.1743331960759,-2.28349397809555));
#93633=CARTESIAN_POINT('Ctrl Pts',(7.60037559731866,-8.42908729095345,-9.05150436343379));
#93634=CARTESIAN_POINT('Ctrl Pts',(7.87617142963179,-1.40270668032046,-12.2712679337148));
#93635=CARTESIAN_POINT('Ctrl Pts',(8.12094266444456,5.30279634249133,-10.860966895162));
#93636=CARTESIAN_POINT('Ctrl Pts',(8.33483813586797,9.61619727452542,-6.94314027168755));
#93637=CARTESIAN_POINT('Ctrl Pts',(8.51798011869584,11.6107486373453,-2.37266665322963));
#93638=CARTESIAN_POINT('Ctrl Pts',(8.70092420271314,11.5440204005338,2.60719448233829));
#93639=CARTESIAN_POINT('Ctrl Pts',(8.90397235759044,9.21032715117327,7.62361020233496));
#93640=CARTESIAN_POINT('Ctrl Pts',(9.08647734189219,5.15501713728993,10.6392974998355));
#93641=CARTESIAN_POINT('Ctrl Pts',(9.26877643799424,0.361793133769277,11.6830912584508));
#93642=CARTESIAN_POINT('Ctrl Pts',(9.430664325476,-4.00483936387056,11.0848200731915));
#93643=CARTESIAN_POINT('Ctrl Pts',(9.61257868421856,-8.19580469716808,8.4438069689631));
#93644=CARTESIAN_POINT('Ctrl Pts',(9.82456303798387,-11.3938252065926,3.63741421882482));
#93645=CARTESIAN_POINT('Ctrl Pts',(10.0664719630594,-11.7795844654107,-3.12660926401823));
#93646=CARTESIAN_POINT('Ctrl Pts',(10.2928503059377,-8.2973304430841,-8.42702524023792));
#93647=CARTESIAN_POINT('Ctrl Pts',(10.4737043934838,-4.04650394557917,-10.8147950872555));
#93648=CARTESIAN_POINT('Ctrl Pts',(10.6543909804151,0.732894864854846,-11.7767781854194));
#93649=CARTESIAN_POINT('Ctrl Pts',(10.8498591133757,5.98692392555446,-10.2580419437641));
#93650=CARTESIAN_POINT('Ctrl Pts',(11.0600325724026,9.92751353416783,-6.1035108728662));
#93651=CARTESIAN_POINT('Ctrl Pts',(11.2399512369267,11.546460582177,-1.47936245392121));
#93652=CARTESIAN_POINT('Ctrl Pts',(11.3996731072529,11.1624047905268,2.85148184763383));
#93653=CARTESIAN_POINT('Ctrl Pts',(11.5791658207047,9.10827354395886,7.22309597989244));
#93654=CARTESIAN_POINT('Ctrl Pts',(11.7584243417152,5.33277954211481,10.4444566098854));
#93655=CARTESIAN_POINT('Ctrl Pts',(11.9572932478171,0.0326178630782873,
11.5764970906776));
#93656=CARTESIAN_POINT('Ctrl Pts',(12.1360376686652,-4.72461621902352,10.5559808042784));
#93657=CARTESIAN_POINT('Ctrl Pts',(12.3145418868021,-8.63351244335065,7.66662870298955));
#93658=CARTESIAN_POINT('Ctrl Pts',(12.5225155707071,-11.4114946324002,2.72871466178511));
#93659=CARTESIAN_POINT('Ctrl Pts',(12.7597959443576,-11.2923500573187,-3.91302535507406));
#93660=CARTESIAN_POINT('Ctrl Pts',(13.0261856238862,-6.74514927963575,-9.83368730756411));
#93661=CARTESIAN_POINT('Ctrl Pts',(13.292021165761,0.409157784142408,-11.8924724744053));
#93662=CARTESIAN_POINT('Ctrl Pts',(13.557298875633,7.37603514967898,-9.30672631479365));
#93663=CARTESIAN_POINT('Ctrl Pts',(13.8220144202162,11.43603621917,-3.10140811095855));
#93664=CARTESIAN_POINT('Ctrl Pts',(14.086165589555,11.0204456508738,4.28435228537355));
#93665=CARTESIAN_POINT('Ctrl Pts',(14.3497490950746,6.30779512977284,9.97248011234989));
#93666=CARTESIAN_POINT('Ctrl Pts',(14.5835381803786,-0.0464713597019573,
11.5403085937317));
#93667=CARTESIAN_POINT('Ctrl Pts',(14.7877335980687,-5.37998875590803,9.95988209741448));
#93668=CARTESIAN_POINT('Ctrl Pts',(14.9625028495183,-8.98758107606861,6.85885374524538));
#93669=CARTESIAN_POINT('Ctrl Pts',(15.1370166293793,-10.9962276335929,2.55034433801783));
#93670=CARTESIAN_POINT('Ctrl Pts',(15.3112747861453,-11.057316471522,-2.19384403747148));
#93671=CARTESIAN_POINT('Ctrl Pts',(15.4852762580546,-9.16194215872132,-6.53762558663525));
#93672=CARTESIAN_POINT('Ctrl Pts',(15.6590212752161,-5.65505712284883,-9.71224134793712));
#93673=CARTESIAN_POINT('Ctrl Pts',(15.8325093831332,-1.15683632859144,-11.1621233815762));
#93674=CARTESIAN_POINT('Ctrl Pts',(16.0057407273942,3.52850982383791,-10.634588642758));
#93675=CARTESIAN_POINT('Ctrl Pts',(16.2075439831294,8.26078713351443,-7.83231510161214));
#93676=CARTESIAN_POINT('Ctrl Pts',(16.3945835370073,10.79301239595,-3.25410627544597));
#93677=CARTESIAN_POINT('Ctrl Pts',(16.5669469472843,10.9149944222274,1.39566838694312));
#93678=CARTESIAN_POINT('Ctrl Pts',(16.7175961104587,9.75994551453762,5.28890387414351));
#93679=CARTESIAN_POINT('Ctrl Pts',(16.8895254520512,6.77373145232914,8.93163549966943));
#93680=CARTESIAN_POINT('Ctrl Pts',(17.0826211217225,1.91369898979447,11.025856134666));
#93681=CARTESIAN_POINT('Ctrl Pts',(17.2753922254922,-3.3508976031883,10.6555208202389));
#93682=CARTESIAN_POINT('Ctrl Pts',(17.4892223589,-8.36495116825048,7.61549170937787));
#93683=CARTESIAN_POINT('Ctrl Pts',(17.7239740129484,-11.323999962384,1.74977000123159));
#93684=CARTESIAN_POINT('Ctrl Pts',(17.9794946102052,-10.1334781781364,-5.31086964421616));
#93685=CARTESIAN_POINT('Ctrl Pts',(18.2131956523234,-5.41461046876539,-9.84567084479958));
#93686=CARTESIAN_POINT('Ctrl Pts',(18.4252409173706,0.2689155062104,-11.0547790277262));
#93687=CARTESIAN_POINT('Ctrl Pts',(18.6157538537825,5.30353569117718,-9.68430051555971));
#93688=CARTESIAN_POINT('Ctrl Pts',(18.8059711829349,9.14161879340698,-6.15840703222966));
#93689=CARTESIAN_POINT('Ctrl Pts',(18.9958193954241,10.9301430713354,-1.27390300512045));
#93690=CARTESIAN_POINT('Ctrl Pts',(19.1854745393041,10.2785058526305,3.87847986224289));
#93691=CARTESIAN_POINT('Ctrl Pts',(19.3745566088602,7.33965248047654,8.15027554492915));
#93692=CARTESIAN_POINT('Ctrl Pts',(19.5638226072173,2.77544111869361,10.5915075520203));
#93693=CARTESIAN_POINT('Ctrl Pts',(19.7519388114443,-2.39136880705402,10.6682602417168));
#93694=CARTESIAN_POINT('Ctrl Pts',(19.9410928244703,-7.0098241819731,8.36292115754712));
#93695=CARTESIAN_POINT('Ctrl Pts',(20.1271442720693,-10.0503377871766,4.21349399010993));
#93696=CARTESIAN_POINT('Ctrl Pts',(20.3240622194817,-10.8431563294057,-0.880894283363258));
#93697=CARTESIAN_POINT('Ctrl Pts',(20.4450629396927,-9.21826875757226,-5.75417784878344));
#93698=CARTESIAN_POINT('Ctrl Pts',(20.5989705638437,-5.54148991110627,-9.330623077557));
#93699=CARTESIAN_POINT('Ctrl Pts',(20.7367118993859,-0.639233991474592,
-10.8209454851943));
#93700=CARTESIAN_POINT('Ctrl Pts',(20.8821091417125,4.39406593230452,-9.8944887684073));
#93701=CARTESIAN_POINT('Ctrl Pts',(21.0236016284966,8.43547518933461,-6.76521535821915));
#93702=CARTESIAN_POINT('Ctrl Pts',(21.1666348355068,10.5870605911627,-2.13587908149872));
#93703=CARTESIAN_POINT('Ctrl Pts',(21.3087336481745,10.3737327496134,2.95997788375124));
#93704=CARTESIAN_POINT('Ctrl Pts',(21.4510017239846,7.84825374656463,7.380423184045));
#93705=CARTESIAN_POINT('Ctrl Pts',(21.59294179475,3.58032156429269,10.1533105718855));
#93706=CARTESIAN_POINT('Ctrl Pts',(21.7348140241776,-1.47776662004928,10.6402982054532));
#93707=CARTESIAN_POINT('Ctrl Pts',(21.8764055683373,-6.19000771396059,8.788190550891));
#93708=CARTESIAN_POINT('Ctrl Pts',(22.0385534863357,-10.0035800617522,4.35288066991984));
#93709=CARTESIAN_POINT('Ctrl Pts',(22.1528974355741,-10.5806803818037,0.292347047550849));
#93710=CARTESIAN_POINT('Ctrl Pts',(22.2212444823395,-10.0989252768157,-2.23060044547888));
#93711=CARTESIAN_POINT('Ctrl Pts',(0.423670339017024,11.5945440159359,-2.5274869736091));
#93712=CARTESIAN_POINT('Ctrl Pts',(0.499910026360594,12.1482059396284,0.288878858844674));
#93713=CARTESIAN_POINT('Ctrl Pts',(0.632109379329947,11.4845538919804,4.9846161952424));
#93714=CARTESIAN_POINT('Ctrl Pts',(0.817612579386571,7.11199402872522,10.0533146758472));
#93715=CARTESIAN_POINT('Ctrl Pts',(0.979985218407911,1.71424573113258,12.1825515349628));
#93716=CARTESIAN_POINT('Ctrl Pts',(1.14226800128799,-4.07414027681685,11.6205930393753));
#93717=CARTESIAN_POINT('Ctrl Pts',(1.30457476479594,-8.95288746042918,8.45215882401799));
#93718=CARTESIAN_POINT('Ctrl Pts',(1.46705658537464,-11.8369449681502,3.40204576066399));
#93719=CARTESIAN_POINT('Ctrl Pts',(1.62919612679919,-12.0795032442586,-2.41181865880537));
#93720=CARTESIAN_POINT('Ctrl Pts',(1.7922231908137,-9.62655368386558,-7.68820709553356));
#93721=CARTESIAN_POINT('Ctrl Pts',(1.95333642472349,-5.02430928732878,-11.2508211808369));
#93722=CARTESIAN_POINT('Ctrl Pts',(2.11870241151089,0.700466955544165,-12.3033343538523));
#93723=CARTESIAN_POINT('Ctrl Pts',(2.27520347918107,6.27024822871081,-10.6103749171108));
#93724=CARTESIAN_POINT('Ctrl Pts',(2.44986594459918,10.4419736262804,-6.54920361312032));
#93725=CARTESIAN_POINT('Ctrl Pts',(2.58707156317327,12.2839753927472,-1.02582701461511));
#93726=CARTESIAN_POINT('Ctrl Pts',(2.80947697362479,11.3852443672071,4.7283936720716));
#93727=CARTESIAN_POINT('Ctrl Pts',(3.02012261112198,7.94675209063415,9.42308149047911));
#93728=CARTESIAN_POINT('Ctrl Pts',(3.25695544175519,2.1558172122942,12.3161751177547));
#93729=CARTESIAN_POINT('Ctrl Pts',(3.51639564443165,-5.08337488329011,11.6384542804377));
#93730=CARTESIAN_POINT('Ctrl Pts',(3.79990696773698,-11.0053104607542,6.34331092371967));
#93731=CARTESIAN_POINT('Ctrl Pts',(4.08317996499983,-12.6136176870944,-1.42687314372758));
#93732=CARTESIAN_POINT('Ctrl Pts',(4.36652199501975,-9.30382142526618,-8.63724843788744));
#93733=CARTESIAN_POINT('Ctrl Pts',(4.64976733453564,-2.35439972201832,-12.4737105684233));
#93734=CARTESIAN_POINT('Ctrl Pts',(4.90150350992193,4.62977560927775,-11.5427208503617));
#93735=CARTESIAN_POINT('Ctrl Pts',(5.12171659361905,9.36028395486059,-7.8512031028979));
#93736=CARTESIAN_POINT('Ctrl Pts',(5.31043357641154,11.7590219812312,-3.31083020027306));
#93737=CARTESIAN_POINT('Ctrl Pts',(5.53055349196105,12.1365080578965,2.67659366125153));
#93738=CARTESIAN_POINT('Ctrl Pts',(5.78204065257121,8.96738060148916,8.96171723805314));
#93739=CARTESIAN_POINT('Ctrl Pts',(6.06484712251421,1.88946402405893,12.5292031204931));
#93740=CARTESIAN_POINT('Ctrl Pts',(6.34751963344422,-5.91395276198827,11.1983677940525));
#93741=CARTESIAN_POINT('Ctrl Pts',(6.63004974724334,-11.4027073465007,5.49642901003884));
#93742=CARTESIAN_POINT('Ctrl Pts',(6.91241907517974,-12.4304112089619,-2.34661336699943));
#93743=CARTESIAN_POINT('Ctrl Pts',(7.19461683901169,-8.60493455977115,-9.26183221523559));
#93744=CARTESIAN_POINT('Ctrl Pts',(7.47663110699745,-1.42059143694494,-12.5551778481077));
#93745=CARTESIAN_POINT('Ctrl Pts',(7.7271314516778,5.44207090065182,-11.1127539908751));
#93746=CARTESIAN_POINT('Ctrl Pts',(7.94618529937553,9.85975525065126,-7.10070001078025));
#93747=CARTESIAN_POINT('Ctrl Pts',(8.13384686792588,11.9037917265843,-2.41755821962657));
#93748=CARTESIAN_POINT('Ctrl Pts',(8.32140797882049,11.8356666147205,2.68798146599893));
#93749=CARTESIAN_POINT('Ctrl Pts',(8.52969267973505,9.44210865594734,7.83388635082118));
#93750=CARTESIAN_POINT('Ctrl Pts',(8.7170210774575,5.27991968869386,10.9296745279879));
#93751=CARTESIAN_POINT('Ctrl Pts',(8.90423692873056,0.357432150175136,12.0017609531342));
#93752=CARTESIAN_POINT('Ctrl Pts',(9.07056383278122,-4.12894815337104,11.3873305431638));
#93753=CARTESIAN_POINT('Ctrl Pts',(9.2575629576071,-8.43721289934054,8.67272832383416));
#93754=CARTESIAN_POINT('Ctrl Pts',(9.47558408444354,-11.7265578415237,3.7296686533837));
#93755=CARTESIAN_POINT('Ctrl Pts',(9.7245411344107,-12.1243895083082,-3.23133011071166));
#93756=CARTESIAN_POINT('Ctrl Pts',(9.95768828784286,-8.53865012954471,-8.69066976617957));
#93757=CARTESIAN_POINT('Ctrl Pts',(10.1440524905267,-4.15835460390148,-11.1513280757522));
#93758=CARTESIAN_POINT('Ctrl Pts',(10.3303115703698,0.768371413765467,-12.1431266911025));
#93759=CARTESIAN_POINT('Ctrl Pts',(10.5319176514054,6.1875553550476,-10.5772889499276));
#93760=CARTESIAN_POINT('Ctrl Pts',(10.7488175153498,10.2544916217239,-6.28999306444741));
#93761=CARTESIAN_POINT('Ctrl Pts',(10.9345802297141,11.9262575937623,-1.51572827249708));
#93762=CARTESIAN_POINT('Ctrl Pts',(11.0995661281895,11.5297510391498,2.95786818177737));
#93763=CARTESIAN_POINT('Ctrl Pts',(11.2850434916283,9.4072473885783,7.47527420050668));
#93764=CARTESIAN_POINT('Ctrl Pts',(11.4703614167965,5.50440093654708,10.8058306130731));
#93765=CARTESIAN_POINT('Ctrl Pts',(11.6760576098715,0.0223254280214599,
11.977008200122));
#93766=CARTESIAN_POINT('Ctrl Pts',(11.8610173200076,-4.90036432229749,10.9212226493378));
#93767=CARTESIAN_POINT('Ctrl Pts',(12.0458069090812,-8.94702876856218,7.93031395909145));
#93768=CARTESIAN_POINT('Ctrl Pts',(12.2611920470817,-11.8242343241244,2.81657705125164));
#93769=CARTESIAN_POINT('Ctrl Pts',(12.507054950679,-11.7014296258157,-4.06536850085611));
#93770=CARTESIAN_POINT('Ctrl Pts',(12.7832424374564,-6.98756758515652,-10.204238068239));
#93771=CARTESIAN_POINT('Ctrl Pts',(13.0590144035629,0.433956965789265,-12.3406476876779));
#93772=CARTESIAN_POINT('Ctrl Pts',(13.3343616190032,7.6655120483341,-9.65738889411834));
#93773=CARTESIAN_POINT('Ctrl Pts',(13.609272528718,11.8824312629553,-3.21343169127533));
#93774=CARTESIAN_POINT('Ctrl Pts',(13.8837411210347,11.4512344395676,4.46083420421942));
#93775=CARTESIAN_POINT('Ctrl Pts',(14.157756841466,6.55253517995481,10.37448148582));
#93776=CARTESIAN_POINT('Ctrl Pts',(14.4009162181298,-0.0562993866030424,
12.0056367310909));
#93777=CARTESIAN_POINT('Ctrl Pts',(14.613377610303,-5.60579188925755,10.3614149373415));
#93778=CARTESIAN_POINT('Ctrl Pts',(14.7952761706161,-9.36063725916999,7.13400533499643));
#93779=CARTESIAN_POINT('Ctrl Pts',(14.9769616528988,-11.4519683094566,2.64850567104104));
#93780=CARTESIAN_POINT('Ctrl Pts',(15.1584316174266,-11.5157281433124,-2.29202178385935));
#93781=CARTESIAN_POINT('Ctrl Pts',(15.3396841079563,-9.5415030993255,-6.81686991985697));
#93782=CARTESIAN_POINT('Ctrl Pts',(15.520716584191,-5.88761675003304,-10.1247386305629));
#93783=CARTESIAN_POINT('Ctrl Pts',(15.7015273430644,-1.19957735055218,-11.635944756842));
#93784=CARTESIAN_POINT('Ctrl Pts',(15.8821144770507,3.6847281306788,-11.0861297401642));
#93785=CARTESIAN_POINT('Ctrl Pts',(16.092535838484,8.61916674222325,-8.164317052411));
#93786=CARTESIAN_POINT('Ctrl Pts',(16.2876180879184,11.2605086022686,-3.38938545620713));
#93787=CARTESIAN_POINT('Ctrl Pts',(16.4674350022227,11.3878313110805,1.46147344387607));
#93788=CARTESIAN_POINT('Ctrl Pts',(16.6246226123464,10.1826987634612,5.523689705124));
#93789=CARTESIAN_POINT('Ctrl Pts',(16.8040468044215,7.06640964607396,9.32529450302247));
#93790=CARTESIAN_POINT('Ctrl Pts',(17.0056015586567,1.99352102361405,11.5113829717538));
#93791=CARTESIAN_POINT('Ctrl Pts',(17.2068563683828,-3.50277342848018,11.1248679174581));
#93792=CARTESIAN_POINT('Ctrl Pts',(17.4301372643576,-8.73849927430506,7.95059990444826));
#93793=CARTESIAN_POINT('Ctrl Pts',(17.6753124404026,-11.8291357002828,1.82452958899942));
#93794=CARTESIAN_POINT('Ctrl Pts',(17.9422312867441,-10.5857337571376,-5.55110411124777));
#93795=CARTESIAN_POINT('Ctrl Pts',(18.1864008297577,-5.65560812392042,-10.2891705783639));
#93796=CARTESIAN_POINT('Ctrl Pts',(18.4079732642625,0.283267861568415,-11.5526785802843));
#93797=CARTESIAN_POINT('Ctrl Pts',(18.6070659207362,5.54463515770339,-10.1205401749562));
#93798=CARTESIAN_POINT('Ctrl Pts',(18.8058667587473,9.55594572003318,-6.43558073229036));
#93799=CARTESIAN_POINT('Ctrl Pts',(19.004296009319,11.4253516620804,-1.33031017300727));
#93800=CARTESIAN_POINT('Ctrl Pts',(19.2025352896204,10.7442529016399,4.05527348946615));
#93801=CARTESIAN_POINT('Ctrl Pts',(19.4001836338508,7.6722717924416,8.52063310338956));
#93802=CARTESIAN_POINT('Ctrl Pts',(19.5980315539952,2.90113062562472,11.072540055233));
#93803=CARTESIAN_POINT('Ctrl Pts',(19.7946776467893,-2.5000090595846,11.1528230858435));
#93804=CARTESIAN_POINT('Ctrl Pts',(19.9924152586705,-7.32795514376305,8.74282571258241));
#93805=CARTESIAN_POINT('Ctrl Pts',(20.1868948262722,-10.506301854141,4.40543523386043));
#93806=CARTESIAN_POINT('Ctrl Pts',(20.3927492397039,-11.3350287821838,-0.920131778514912));
#93807=CARTESIAN_POINT('Ctrl Pts',(20.5192302799543,-9.63653174764009,-6.01425458044086));
#93808=CARTESIAN_POINT('Ctrl Pts',(20.6801053219349,-5.79329331148848,-9.75250286771838));
#93809=CARTESIAN_POINT('Ctrl Pts',(20.824073482086,-0.669397782210286,-11.3102133361092));
#93810=CARTESIAN_POINT('Ctrl Pts',(20.9760363808395,4.59117028503297,-10.341855027379));
#93811=CARTESIAN_POINT('Ctrl Pts',(21.1239075502339,8.81475307055138,-7.07151228909026));
#93812=CARTESIAN_POINT('Ctrl Pts',(21.2733782519326,11.0631196578749,-2.23372990206915));
#93813=CARTESIAN_POINT('Ctrl Pts',(21.4218610235557,10.8401809746124,3.09085572555693));
#93814=CARTESIAN_POINT('Ctrl Pts',(21.5705041401616,8.20139051869354,7.7097335231965));
#93815=CARTESIAN_POINT('Ctrl Pts',(21.7188009929258,3.74263352723652,10.6058633049019));
#93816=CARTESIAN_POINT('Ctrl Pts',(21.8669806048059,-1.54112766069498,11.1157326171366));
#93817=CARTESIAN_POINT('Ctrl Pts',(22.0149272318989,-6.46295628686545,9.17861775642755));
#93818=CARTESIAN_POINT('Ctrl Pts',(22.184149004847,-10.4455333151633,4.55128270428701));
#93819=CARTESIAN_POINT('Ctrl Pts',(22.303825740982,-11.0480802116222,0.300873741754191));
#93820=CARTESIAN_POINT('Ctrl Pts',(22.374548238521,-10.5449815461394,-2.31029863300481));
#93821=CARTESIAN_POINT('Ctrl Pts',(0.000900289619140335,11.3804638834915,
-2.47613834775811));
#93822=CARTESIAN_POINT('Ctrl Pts',(0.0760295925109289,11.9237491928521,
0.298886540614988));
#93823=CARTESIAN_POINT('Ctrl Pts',(0.205681996899962,11.2728196273968,4.90414136366958));
#93824=CARTESIAN_POINT('Ctrl Pts',(0.38794973553318,6.97799472302775,9.88526793682913));
#93825=CARTESIAN_POINT('Ctrl Pts',(0.547505005240074,1.67325159616518,11.9771828269468));
#93826=CARTESIAN_POINT('Ctrl Pts',(0.707085602513105,-4.01842843579301,
11.4254349394003));
#93827=CARTESIAN_POINT('Ctrl Pts',(0.866758979071408,-8.81835900038039,
8.30837071392562));
#93828=CARTESIAN_POINT('Ctrl Pts',(1.02669281100368,-11.6574299498413,3.33779701847597));
#93829=CARTESIAN_POINT('Ctrl Pts',(1.1863696529269,-11.8966938796723,-2.38782040177236));
#93830=CARTESIAN_POINT('Ctrl Pts',(1.34700769853469,-9.48000818153135,-7.58698885918058));
#93831=CARTESIAN_POINT('Ctrl Pts',(1.50583823722894,-4.94319286098826,-11.0993660324489));
#93832=CARTESIAN_POINT('Ctrl Pts',(1.66895327102401,0.703563529205378,-12.1380990070998));
#93833=CARTESIAN_POINT('Ctrl Pts',(1.82340078503438,6.20026236479091,-10.4672689721285));
#93834=CARTESIAN_POINT('Ctrl Pts',(1.99586293482947,10.3199138911453,-6.45818496655306));
#93835=CARTESIAN_POINT('Ctrl Pts',(2.13140208596345,12.1396560511668,-1.0012609065115));
#93836=CARTESIAN_POINT('Ctrl Pts',(2.35147265048197,11.2517822360554,4.69337676657042));
#93837=CARTESIAN_POINT('Ctrl Pts',(2.55971574243581,7.85115399103111,9.33401839064537));
#93838=CARTESIAN_POINT('Ctrl Pts',(2.79422737759169,2.11861543132166,12.2002863161899));
#93839=CARTESIAN_POINT('Ctrl Pts',(3.0512206555009,-5.0531972452128,11.5288550107248));
#93840=CARTESIAN_POINT('Ctrl Pts',(3.33238525234115,-10.9266143368972,6.27934698525193));
#93841=CARTESIAN_POINT('Ctrl Pts',(3.6135516195531,-12.5241293849237,-1.43321866908381));
#93842=CARTESIAN_POINT('Ctrl Pts',(3.895065976677,-9.23684114979357,-8.59733339719354));
#93843=CARTESIAN_POINT('Ctrl Pts',(4.17674612036772,-2.3263774897798,-12.4137395464659));
#93844=CARTESIAN_POINT('Ctrl Pts',(4.42733432200923,4.62604823359843,-11.4880055956006));
#93845=CARTESIAN_POINT('Ctrl Pts',(4.64671446045608,9.33895743109829,-7.81077468702255));
#93846=CARTESIAN_POINT('Ctrl Pts',(4.83483829661682,11.7304278021032,-3.28483832386075));
#93847=CARTESIAN_POINT('Ctrl Pts',(5.05440724020435,12.1074033960408,2.68751675904296));
#93848=CARTESIAN_POINT('Ctrl Pts',(5.30546640657026,8.94463140752224,8.96236282495723));
#93849=CARTESIAN_POINT('Ctrl Pts',(5.58806199031735,1.87258526440905,12.528277867321));
#93850=CARTESIAN_POINT('Ctrl Pts',(5.87079511955371,-5.93268261644051,11.1983565302455));
#93851=CARTESIAN_POINT('Ctrl Pts',(6.15365719351318,-11.428734123529,5.49059286230551));
#93852=CARTESIAN_POINT('Ctrl Pts',(6.43662965392189,-12.4598385816407,-2.36901622871161));
#93853=CARTESIAN_POINT('Ctrl Pts',(6.71970157861287,-8.62358728920016,-9.3061984871583));
#93854=CARTESIAN_POINT('Ctrl Pts',(7.00286024125015,-1.41063629995952,-12.6140167198692));
#93855=CARTESIAN_POINT('Ctrl Pts',(7.25461839642261,5.48668947887283,-11.1653717969649));
#93856=CARTESIAN_POINT('Ctrl Pts',(7.47494586003375,9.93035099743477,-7.13029121147144));
#93857=CARTESIAN_POINT('Ctrl Pts',(7.66381885286863,11.9878796392882,-2.41707720971809));
#93858=CARTESIAN_POINT('Ctrl Pts',(7.85271039473043,11.9196078305902,2.72466571552369));
#93859=CARTESIAN_POINT('Ctrl Pts',(8.06260425041251,9.50793750751671,7.91045632829471));
#93860=CARTESIAN_POINT('Ctrl Pts',(8.25151943811564,5.31086519215702,11.0329345940469));
#93861=CARTESIAN_POINT('Ctrl Pts',(8.4404389964955,0.343601266253404,12.1149463652386));
#93862=CARTESIAN_POINT('Ctrl Pts',(8.60836913040726,-4.18601440528256,11.4948946391602));
#93863=CARTESIAN_POINT('Ctrl Pts',(8.79728667337804,-8.53866643130548,8.75273207656539));
#93864=CARTESIAN_POINT('Ctrl Pts',(9.01768164738511,-11.8641266373615,3.75611609832303));
#93865=CARTESIAN_POINT('Ctrl Pts',(9.26954822543693,-12.2676543833531,-3.28608472892146));
#93866=CARTESIAN_POINT('Ctrl Pts',(9.50563786526714,-8.63747604798216,-8.81485613790273));
#93867=CARTESIAN_POINT('Ctrl Pts',(9.69448333045407,-4.19892530952498,-11.3084481812179));
#93868=CARTESIAN_POINT('Ctrl Pts',(9.88330841704327,0.795573210174991,-12.31409890475));
#93869=CARTESIAN_POINT('Ctrl Pts',(10.0878363483475,6.29348062935308,-10.7263386495003));
#93870=CARTESIAN_POINT('Ctrl Pts',(10.3080425852288,10.4227066096295,-6.373952123734));
#93871=CARTESIAN_POINT('Ctrl Pts',(10.4967508502962,12.1212890942399,-1.5241070887372));
#93872=CARTESIAN_POINT('Ctrl Pts',(10.6644551092141,11.7185241015762,3.02321116376383));
#93873=CARTESIAN_POINT('Ctrl Pts',(10.8530809920984,9.56015331219004,7.61733162462507));
#93874=CARTESIAN_POINT('Ctrl Pts',(11.0416565818448,5.58907527410401,11.0068489757527));
#93875=CARTESIAN_POINT('Ctrl Pts',(11.2511145551901,0.00682605008962356,
12.1998226540138));
#93876=CARTESIAN_POINT('Ctrl Pts',(11.4395654059283,-5.008825606421,11.1244108695771));
#93877=CARTESIAN_POINT('Ctrl Pts',(11.6279548005678,-9.13449427634377,8.07551137181917));
#93878=CARTESIAN_POINT('Ctrl Pts',(11.8476610895102,-12.0697351676139,2.85940599125345));
#93879=CARTESIAN_POINT('Ctrl Pts',(12.0986399649365,-11.9453291153835,-4.1656754855368));
#93880=CARTESIAN_POINT('Ctrl Pts',(12.380813347536,-7.1301861622191,-10.4382358096941));
#93881=CARTESIAN_POINT('Ctrl Pts',(12.6628007775777,0.458280864595954,-12.6238052602907));
#93882=CARTESIAN_POINT('Ctrl Pts',(12.9445891529439,7.85932826240679,-9.87877525418112));
#93883=CARTESIAN_POINT('Ctrl Pts',(13.2261623670661,12.1792965341059,-3.27924005831069));
#93884=CARTESIAN_POINT('Ctrl Pts',(13.5075123240597,11.7382981773641,4.58743988341015));
#93885=CARTESIAN_POINT('Ctrl Pts',(13.78862270095,6.7135683306726,10.6548364892803));
#93886=CARTESIAN_POINT('Ctrl Pts',(14.0382770210205,-0.0715674345651694,
12.3303771601699));
#93887=CARTESIAN_POINT('Ctrl Pts',(14.2565522948072,-5.77303535786754,10.6414830835723));
#93888=CARTESIAN_POINT('Ctrl Pts',(14.4435258860147,-9.63278931728537,7.3242445945618));
#93889=CARTESIAN_POINT('Ctrl Pts',(14.6303754923499,-11.7838090680834,2.71138944009352));
#93890=CARTESIAN_POINT('Ctrl Pts',(14.8170958795502,-11.8496754051594,-2.37206455387923));
#93891=CARTESIAN_POINT('Ctrl Pts',(15.0036871297529,-9.81756163638772,-7.03027663503322));
#93892=CARTESIAN_POINT('Ctrl Pts',(15.1901423954911,-6.05440883736194,-10.4374095339218));
#93893=CARTESIAN_POINT('Ctrl Pts',(15.3764600570967,-1.22369089789884,-11.9948963860826));
#93894=CARTESIAN_POINT('Ctrl Pts',(15.562635366768,3.81176920962088,-11.4283094282349));
#93895=CARTESIAN_POINT('Ctrl Pts',(15.7796703137958,8.90143044882656,-8.41495584271175));
#93896=CARTESIAN_POINT('Ctrl Pts',(15.981004715721,11.6279173541602,-3.4873266676171));
#93897=CARTESIAN_POINT('Ctrl Pts',(16.1666763388528,11.7595350467105,1.52149245812212));
#93898=CARTESIAN_POINT('Ctrl Pts',(16.3290372382266,10.5148554672375,5.71740896283513));
#93899=CARTESIAN_POINT('Ctrl Pts',(16.5144448880648,7.29489788686152,9.64596057464015));
#93900=CARTESIAN_POINT('Ctrl Pts',(16.7228234986026,2.05041108784682,11.9063669249619));
#93901=CARTESIAN_POINT('Ctrl Pts',(16.930992551001,-3.63471752235437,11.5068909821674));
#93902=CARTESIAN_POINT('Ctrl Pts',(17.1620546044951,-9.05305178321521,8.22235330647674));
#93903=CARTESIAN_POINT('Ctrl Pts',(17.4159113519357,-12.2537284610614,1.87968497770613));
#93904=CARTESIAN_POINT('Ctrl Pts',(17.6924475759089,-10.9662624459213,-5.76178740457814));
#93905=CARTESIAN_POINT('Ctrl Pts',(17.945566339639,-5.85591523772921,-10.6739734171909));
#93906=CARTESIAN_POINT('Ctrl Pts',(18.1753717303344,0.303573719096216,-11.9847397656707));
#93907=CARTESIAN_POINT('Ctrl Pts',(18.3819490799225,5.76277859895906,-10.4990413623162));
#93908=CARTESIAN_POINT('Ctrl Pts',(18.5883070393005,9.92675289335987,-6.67420313817307));
#93909=CARTESIAN_POINT('Ctrl Pts',(18.7943617430537,11.8682318114508,-1.37288219672597));
#93910=CARTESIAN_POINT('Ctrl Pts',(19.0002970711139,11.1609539414397,4.22186752150935));
#93911=CARTESIAN_POINT('Ctrl Pts',(19.2056993787138,7.96869361929753,8.86238310851352));
#93912=CARTESIAN_POINT('Ctrl Pts',(19.4113749853726,3.00880991732028,11.5157353993555));
#93913=CARTESIAN_POINT('Ctrl Pts',(19.6158941321298,-2.60825633138589,11.5990543182677));
#93914=CARTESIAN_POINT('Ctrl Pts',(19.8215745264496,-7.63078703075867,9.09294033135363));
#93915=CARTESIAN_POINT('Ctrl Pts',(20.0240196534198,-10.9387245165996,4.57767395040845));
#93916=CARTESIAN_POINT('Ctrl Pts',(20.2382196602506,-11.8016588555741,-0.963371624759982));
#93917=CARTESIAN_POINT('Ctrl Pts',(20.3699279122194,-10.0330275954534,-6.2677802445981));
#93918=CARTESIAN_POINT('Ctrl Pts',(20.5374857980306,-6.03037781526117,-10.1616546059296));
#93919=CARTESIAN_POINT('Ctrl Pts',(20.6874666540089,-0.692498617449417,
-11.7843870861828));
#93920=CARTESIAN_POINT('Ctrl Pts',(20.8458089263913,4.78891142674402,-10.7755909958413));
#93921=CARTESIAN_POINT('Ctrl Pts',(20.9999220312606,9.19085121893355,-7.36733395392426));
#93922=CARTESIAN_POINT('Ctrl Pts',(21.1557315978258,11.5346665649489,-2.32438533941469));
#93923=CARTESIAN_POINT('Ctrl Pts',(21.3105437060683,11.302391404217,3.22695219679456));
#93924=CARTESIAN_POINT('Ctrl Pts',(21.4655482862605,8.55068275589101,8.04392519302322));
#93925=CARTESIAN_POINT('Ctrl Pts',(21.6202312153138,3.9003498130575,11.063996769607));
#93926=CARTESIAN_POINT('Ctrl Pts',(21.7747884398775,-1.61158669978775,11.5971907852724));
#93927=CARTESIAN_POINT('Ctrl Pts',(21.9292048348329,-6.74680889827636,9.57370973440197));
#93928=CARTESIAN_POINT('Ctrl Pts',(22.1056736106782,-10.9027234868844,4.74979039067917));
#93929=CARTESIAN_POINT('Ctrl Pts',(22.2308646891255,-11.5318780889901,0.303165289390478));
#93930=CARTESIAN_POINT('Ctrl Pts',(22.304029593088,-11.0066085895293,-2.39878637653492));
#93931=CARTESIAN_POINT('Ctrl Pts',(-0.274269641050573,11.0004695673906,
-2.39761094709083));
#93932=CARTESIAN_POINT('Ctrl Pts',(-0.201135280450074,11.5254245847803,
0.303191618745211));
#93933=CARTESIAN_POINT('Ctrl Pts',(-0.076018233199116,10.8966599438403,
4.74719998282454));
#93934=CARTESIAN_POINT('Ctrl Pts',(0.100354336277068,6.74303500522591,9.56853913405492));
#93935=CARTESIAN_POINT('Ctrl Pts',(0.254685225272068,1.61062313657491,11.5908849925943));
#93936=CARTESIAN_POINT('Ctrl Pts',(0.409158220632143,-3.89832589267103,
11.0580000084071));
#93937=CARTESIAN_POINT('Ctrl Pts',(0.563757230594105,-8.54615907764945,
8.0395458607866));
#93938=CARTESIAN_POINT('Ctrl Pts',(0.718678293364365,-11.2964009987587,
3.22515286261878));
#93939=CARTESIAN_POINT('Ctrl Pts',(0.87340785468557,-11.5285575146058,-2.3232498873316));
#93940=CARTESIAN_POINT('Ctrl Pts',(1.02913439746881,-9.18597776810957,-7.363536753465));
#93941=CARTESIAN_POINT('Ctrl Pts',(1.18316711498639,-4.78633731515139,-10.7700426512527));
#93942=CARTESIAN_POINT('Ctrl Pts',(1.3414248089356,0.692236946541352,-11.7782646755505));
#93943=CARTESIAN_POINT('Ctrl Pts',(1.49133112294563,6.02737678504246,-10.1564808574998));
#93944=CARTESIAN_POINT('Ctrl Pts',(1.65879364084819,10.0279923142955,-6.26431175924732));
#93945=CARTESIAN_POINT('Ctrl Pts',(1.79044918943787,11.7957247916513,-0.963149160289205));
#93946=CARTESIAN_POINT('Ctrl Pts',(2.00450680071523,10.9332197456105,4.5765641208312));
#93947=CARTESIAN_POINT('Ctrl Pts',(2.20691084524558,7.62686256520766,9.0867291314954));
#93948=CARTESIAN_POINT('Ctrl Pts',(2.4351468519884,2.04896770526915,11.8775245776043));
#93949=CARTESIAN_POINT('Ctrl Pts',(2.68534078308583,-4.93385442790983,11.2237829300574));
#93950=CARTESIAN_POINT('Ctrl Pts',(2.95932835724008,-10.6578654904289,6.1096651465346));
#93951=CARTESIAN_POINT('Ctrl Pts',(3.23352058266583,-12.2167042661632,-1.41175057439282));
#93952=CARTESIAN_POINT('Ctrl Pts',(3.50827847232005,-9.00925924299354,-8.40424538776617));
#93953=CARTESIAN_POINT('Ctrl Pts',(3.78342130461475,-2.25959033454623,-12.1330610356035));
#93954=CARTESIAN_POINT('Ctrl Pts',(4.02839617829052,4.53728952345717,-11.228935417426));
#93955=CARTESIAN_POINT('Ctrl Pts',(4.24301582882195,9.14819504519508,-7.63175549721547));
#93956=CARTESIAN_POINT('Ctrl Pts',(4.42716125447877,11.489350822963,-3.20165828960071));
#93957=CARTESIAN_POINT('Ctrl Pts',(4.64220730361779,11.8589357929702,2.64765770593709));
#93958=CARTESIAN_POINT('Ctrl Pts',(4.88827003082658,8.75992235184213,8.79806219469721));
#93959=CARTESIAN_POINT('Ctrl Pts',(5.16548273281936,1.82302921333241,12.2970640865527));
#93960=CARTESIAN_POINT('Ctrl Pts',(5.44307400835471,-5.84053666929798,10.9923890055324));
#93961=CARTESIAN_POINT('Ctrl Pts',(5.72103722792618,-11.2422406693477,5.38420624340654));
#93962=CARTESIAN_POINT('Ctrl Pts',(5.99935768984567,-12.25751466873,-2.3461082746222));
#93963=CARTESIAN_POINT('Ctrl Pts',(6.27802614604401,-8.48189613373607,-9.17597296653521));
#93964=CARTESIAN_POINT('Ctrl Pts',(6.5570329715071,-1.37513713028755,-12.4363664797683));
#93965=CARTESIAN_POINT('Ctrl Pts',(6.80532498827725,5.42752948217785,-11.0086321842624));
#93966=CARTESIAN_POINT('Ctrl Pts',(7.0227875379952,9.8137364793638,-7.02627359380098));
#93967=CARTESIAN_POINT('Ctrl Pts',(7.20931847710744,11.8460716008633,-2.37160812629482));
#93968=CARTESIAN_POINT('Ctrl Pts',(7.39598279382656,11.7789295620232,2.70955515259177));
#93969=CARTESIAN_POINT('Ctrl Pts',(7.6035319327092,9.39456410752855,7.83758421962789));
#93970=CARTESIAN_POINT('Ctrl Pts',(7.79047118958947,5.24170674678976,10.9278934529097));
#93971=CARTESIAN_POINT('Ctrl Pts',(7.97753301867008,0.323277611298938,11.9994386003805));
#93972=CARTESIAN_POINT('Ctrl Pts',(8.14389525793364,-4.16411557432759,11.3854632941077));
#93973=CARTESIAN_POINT('Ctrl Pts',(8.33117028318344,-8.47913095199905,8.66739933230884));
#93974=CARTESIAN_POINT('Ctrl Pts',(8.5497868133909,-11.7780926744232,3.71133890204296));
#93975=CARTESIAN_POINT('Ctrl Pts',(8.79981268641912,-12.1797020209906,-3.27938720685819));
#93976=CARTESIAN_POINT('Ctrl Pts',(9.03440097162593,-8.57341027780405,-8.77362867592834));
#93977=CARTESIAN_POINT('Ctrl Pts',(9.22218188156679,-4.15989549397587,-11.2533688331925));
#93978=CARTESIAN_POINT('Ctrl Pts',(9.41003302249585,0.808765494160608,-12.2540291038378));
#93979=CARTESIAN_POINT('Ctrl Pts',(9.61364471581217,6.2823757029123,-10.6741610615063));
#93980=CARTESIAN_POINT('Ctrl Pts',(9.83304623986146,10.3968674534573,-6.33793941805998));
#93981=CARTESIAN_POINT('Ctrl Pts',(10.0211848030554,12.0906486399765,-1.50282609668041));
#93982=CARTESIAN_POINT('Ctrl Pts',(10.1884870588186,11.6891499040377,3.03367054210446));
#93983=CARTESIAN_POINT('Ctrl Pts',(10.3767631363507,9.53493716486031,7.61934830129794));
#93984=CARTESIAN_POINT('Ctrl Pts',(10.5651100391956,5.56904507615985,11.0052203614278));
#93985=CARTESIAN_POINT('Ctrl Pts',(10.7744673930001,-0.0105150758165145,
12.1980348159159));
#93986=CARTESIAN_POINT('Ctrl Pts',(10.9629516928778,-5.02713480755923,11.1227644880695));
#93987=CARTESIAN_POINT('Ctrl Pts',(11.1514917238607,-9.15634821021125,8.07165786784285));
#93988=CARTESIAN_POINT('Ctrl Pts',(11.3715173352852,-12.0962213591835,2.84818528749816));
#93989=CARTESIAN_POINT('Ctrl Pts',(11.62305833115,-11.9725739258084,-4.19269902494711));
#93990=CARTESIAN_POINT('Ctrl Pts',(11.9061372568435,-7.14292658277634,-10.4861879255579));
#93991=CARTESIAN_POINT('Ctrl Pts',(12.1892998809645,0.476910464515135,-12.6820398490254));
#93992=CARTESIAN_POINT('Ctrl Pts',(12.4725334331891,7.91638967099688,-9.92404980923661));
#93993=CARTESIAN_POINT('Ctrl Pts',(12.7558205103974,12.2636994513997,-3.28495237398259));
#93994=CARTESIAN_POINT('Ctrl Pts',(13.0391515836362,11.8207969469138,4.63725930776699));
#93995=CARTESIAN_POINT('Ctrl Pts',(13.3225108438936,6.75677175138148,10.7540029972883));
#93996=CARTESIAN_POINT('Ctrl Pts',(13.5743965363279,-0.0888694770886342,
12.4455753705037));
#93997=CARTESIAN_POINT('Ctrl Pts',(13.7948007691669,-5.84611408574753,10.7405846022518));
#93998=CARTESIAN_POINT('Ctrl Pts',(13.9837133047971,-9.74613607726721,7.38918223972257));
#93999=CARTESIAN_POINT('Ctrl Pts',(14.1726181730569,-11.9211450660727,2.72569989767666));
#94000=CARTESIAN_POINT('Ctrl Pts',(14.3615117518733,-11.988121384906,-2.41692924665857));
#94001=CARTESIAN_POINT('Ctrl Pts',(14.5503884862477,-9.93140392485721,-7.13237619420355));
#94002=CARTESIAN_POINT('Ctrl Pts',(14.7392452066992,-6.11998765128524,-10.5836631714223));
#94003=CARTESIAN_POINT('Ctrl Pts',(14.9280778158491,-1.22412417528949,-12.1624991437306));
#94004=CARTESIAN_POINT('Ctrl Pts',(15.1168834927693,3.88253460149443,-11.5882300272317));
#94005=CARTESIAN_POINT('Ctrl Pts',(15.3371190205423,9.04745529657373,-8.53078661826523));
#94006=CARTESIAN_POINT('Ctrl Pts',(15.5415710603206,11.8168749142472,-3.52716602342221));
#94007=CARTESIAN_POINT('Ctrl Pts',(15.7302511825858,11.950835437091,1.56286779537959));
#94008=CARTESIAN_POINT('Ctrl Pts',(15.8953162505218,10.6855628547944,5.82871724506087));
#94009=CARTESIAN_POINT('Ctrl Pts',(16.0839158470169,7.41047732554085,9.8251853488451));
#94010=CARTESIAN_POINT('Ctrl Pts',(16.2960238194692,2.07226966928086,12.1265039457095));
#94011=CARTESIAN_POINT('Ctrl Pts',(16.5080591542134,-3.71851480918685,11.7200354231081));
#94012=CARTESIAN_POINT('Ctrl Pts',(16.7435666491117,-9.24138915696723,8.37276765492118));
#94013=CARTESIAN_POINT('Ctrl Pts',(17.0025061938178,-12.5070246239786,1.90348792745417));
#94014=CARTESIAN_POINT('Ctrl Pts',(17.2848235291397,-11.1937440869041,-5.89791089480221));
#94015=CARTESIAN_POINT('Ctrl Pts',(17.5434502580148,-5.9727692152997,-10.917765370183));
#94016=CARTESIAN_POINT('Ctrl Pts',(17.7784330357828,0.325439291644578,-12.2585604897127));
#94017=CARTESIAN_POINT('Ctrl Pts',(17.9897960153653,5.91125375060957,-10.7388470513632));
#94018=CARTESIAN_POINT('Ctrl Pts',(18.2010656267775,10.1746651964443,-6.82324727932377));
#94019=CARTESIAN_POINT('Ctrl Pts',(18.4121556179949,12.1639803531377,-1.39254738980368));
#94020=CARTESIAN_POINT('Ctrl Pts',(18.623249012421,11.439407044246,4.34255520019844));
#94021=CARTESIAN_POINT('Ctrl Pts',(18.833930169963,8.16546807026437,9.10231198480979));
#94022=CARTESIAN_POINT('Ctrl Pts',(19.0450003933591,3.07545188059067,11.8261473540039));
#94023=CARTESIAN_POINT('Ctrl Pts',(19.2550466668237,-2.69287874609835,11.911356465016));
#94024=CARTESIAN_POINT('Ctrl Pts',(19.4663250727336,-7.85339118005448,9.33825389834762));
#94025=CARTESIAN_POINT('Ctrl Pts',(19.674563394974,-11.2548968968117,4.6933339960141));
#94026=CARTESIAN_POINT('Ctrl Pts',(19.8947281535767,-12.1430001285698,-1.00131534254292));
#94027=CARTESIAN_POINT('Ctrl Pts',(20.0302869032443,-10.3227462744336,-6.46036505053996));
#94028=CARTESIAN_POINT('Ctrl Pts',(20.2028081276818,-6.20191802184683,-10.470307721667));
#94029=CARTESIAN_POINT('Ctrl Pts',(20.3572959081572,-0.703609801586646,
-12.1417469327381));
#94030=CARTESIAN_POINT('Ctrl Pts',(20.5204610212607,4.94483734805194,-11.1026481640325));
#94031=CARTESIAN_POINT('Ctrl Pts',(20.6793382723823,9.48304514425589,-7.58922197930745));
#94032=CARTESIAN_POINT('Ctrl Pts',(20.8400261065306,11.9004900835925,-2.38841591491118));
#94033=CARTESIAN_POINT('Ctrl Pts',(20.9997527597285,11.6611545549498,3.33902598665685));
#94034=CARTESIAN_POINT('Ctrl Pts',(21.1597380220168,8.82116047529457,8.31122758162113));
#94035=CARTESIAN_POINT('Ctrl Pts',(21.3194635002342,4.01963780285365,11.4293273846779));
#94036=CARTESIAN_POINT('Ctrl Pts',(21.4790975980088,-1.67397197125274,11.9812737524744));
#94037=CARTESIAN_POINT('Ctrl Pts',(21.6387068761042,-6.98053832771844,9.88862498096864));
#94038=CARTESIAN_POINT('Ctrl Pts',(21.8210381178984,-11.2768707271801,4.90577138996948));
#94039=CARTESIAN_POINT('Ctrl Pts',(21.950736446027,-11.9279866435774,0.298808494733318));
#94040=CARTESIAN_POINT('Ctrl Pts',(22.0258906953141,-11.3845340025562,-2.4770968460111));
#94041=CARTESIAN_POINT('Ctrl Pts',(-0.342078111258781,10.5385239376104,
-2.30907696986698));
#94042=CARTESIAN_POINT('Ctrl Pts',(-0.271391112954986,11.0413243101621,
0.300787646455928));
#94043=CARTESIAN_POINT('Ctrl Pts',(-0.151790900733858,10.4391275085012,
4.54845706796136));
#94044=CARTESIAN_POINT('Ctrl Pts',(0.0173289685761135,6.45898872181764,
9.17301359026322));
#94045=CARTESIAN_POINT('Ctrl Pts',(0.165184575802352,1.54017202925644,11.1089082992411));
#94046=CARTESIAN_POINT('Ctrl Pts',(0.313274054906384,-3.74035295571867,
10.5993670185937));
#94047=CARTESIAN_POINT('Ctrl Pts',(0.461480450893154,-8.19638378875494,
7.70499910147591));
#94048=CARTESIAN_POINT('Ctrl Pts',(0.610033066368199,-10.8335607401376,
3.08895036516842));
#94049=CARTESIAN_POINT('Ctrl Pts',(0.758425688373396,-11.0563640988628,
-2.23239233265665));
#94050=CARTESIAN_POINT('Ctrl Pts',(0.907805392951706,-8.80936728323739,
-7.06721474411051));
#94051=CARTESIAN_POINT('Ctrl Pts',(1.05558749393355,-4.5883542812499,-10.3355905940881));
#94052=CARTESIAN_POINT('Ctrl Pts',(1.20745702701853,0.669020108857811,-11.3033060660648));
#94053=CARTESIAN_POINT('Ctrl Pts',(1.35134080974254,5.789809206371,-9.74664754437023));
#94054=CARTESIAN_POINT('Ctrl Pts',(1.51211172233338,9.63072280992876,-6.01039119164893));
#94055=CARTESIAN_POINT('Ctrl Pts',(1.63852912473268,11.3281842217455,-0.919880530777273));
#94056=CARTESIAN_POINT('Ctrl Pts',(1.84422696532119,10.4999572635067,4.40380525519473));
#94057=CARTESIAN_POINT('Ctrl Pts',(2.03864904197804,7.32344207081827,8.73590098616535));
#94058=CARTESIAN_POINT('Ctrl Pts',(2.25804528095925,1.96228541100584,11.4192375806519));
#94059=CARTESIAN_POINT('Ctrl Pts',(2.49859694289973,-4.75177863315334,10.7907046256551));
#94060=CARTESIAN_POINT('Ctrl Pts',(2.76217572136555,-10.2585538162154,5.87169453114436));
#94061=CARTESIAN_POINT('Ctrl Pts',(3.02606783573862,-11.7594204097944,-1.36721213881776));
#94062=CARTESIAN_POINT('Ctrl Pts',(3.2906456441965,-8.67140560944054,-8.10074009311899));
#94063=CARTESIAN_POINT('Ctrl Pts',(3.55573137608955,-2.16878112255051,-11.6938502007532));
#94064=CARTESIAN_POINT('Ctrl Pts',(3.79188453176902,4.38335528919225,-10.8228371958529));
#94065=CARTESIAN_POINT('Ctrl Pts',(3.9988685297872,8.83037624726696,-7.35382587376631));
#94066=CARTESIAN_POINT('Ctrl Pts',(4.17653174548993,11.0892681298178,-3.07977873822734));
#94067=CARTESIAN_POINT('Ctrl Pts',(4.38408991959369,11.4462359752871,2.56580322371247));
#94068=CARTESIAN_POINT('Ctrl Pts',(4.62170526191261,8.45420647422841,8.50527953784366));
#94069=CARTESIAN_POINT('Ctrl Pts',(4.88956462289703,1.75175609268675,11.8868850409351));
#94070=CARTESIAN_POINT('Ctrl Pts',(5.1579605953482,-5.65803149243908,10.6261941333783));
#94071=CARTESIAN_POINT('Ctrl Pts',(5.426889583736,-10.8847053678964,5.20087057403979));
#94072=CARTESIAN_POINT('Ctrl Pts',(5.6963440916033,-11.8684406358239,-2.28303986368077));
#94073=CARTESIAN_POINT('Ctrl Pts',(5.96631928763454,-8.21135175237803,-8.90018015900593));
#94074=CARTESIAN_POINT('Ctrl Pts',(6.23680942051052,-1.3219346212245,-12.0618160834734));
#94075=CARTESIAN_POINT('Ctrl Pts',(6.47769576851895,5.27793256781067,-10.677406515464));
#94076=CARTESIAN_POINT('Ctrl Pts',(6.68879639076236,9.53602370145207,-6.81177563294094));
#94077=CARTESIAN_POINT('Ctrl Pts',(6.86996019641698,11.5100899515073,-2.29118021789925));
#94078=CARTESIAN_POINT('Ctrl Pts',(7.05134297697175,11.4451001779805,2.64619255534257));
#94079=CARTESIAN_POINT('Ctrl Pts',(7.25311916862402,9.12734611943007,7.6316750467065));
#94080=CARTESIAN_POINT('Ctrl Pts',(7.43496751499411,5.08789384860659,10.6381766966852));
#94081=CARTESIAN_POINT('Ctrl Pts',(7.61702685389441,0.301013202030219,11.6811996322699));
#94082=CARTESIAN_POINT('Ctrl Pts',(7.77901346572604,-4.06831574126187,11.0836178899377));
#94083=CARTESIAN_POINT('Ctrl Pts',(7.96145422098787,-8.27209638982045,8.43595842149749));
#94084=CARTESIAN_POINT('Ctrl Pts',(8.1745399784263,-11.4878311447154,3.60551009010721));
#94085=CARTESIAN_POINT('Ctrl Pts',(8.41840722616007,-11.8804344880585,-3.21286435233645));
#94086=CARTESIAN_POINT('Ctrl Pts',(8.64740235484385,-8.36083904060513,-8.57653734389561));
#94087=CARTESIAN_POINT('Ctrl Pts',(8.8308165934691,-4.05002414261445,-10.9987567640481));
#94088=CARTESIAN_POINT('Ctrl Pts',(9.01437446933271,0.804983153667267,-11.9767120191619));
#94089=CARTESIAN_POINT('Ctrl Pts',(9.21346374406834,6.15713977460773,-10.432629123365));
#94090=CARTESIAN_POINT('Ctrl Pts',(9.42813593686045,10.1831972076906,-6.19012228467193));
#94091=CARTESIAN_POINT('Ctrl Pts',(9.61232353302086,11.8416906339914,-1.45667444959611));
#94092=CARTESIAN_POINT('Ctrl Pts',(9.7762080275955,11.4486469482307,2.98714889568544));
#94093=CARTESIAN_POINT('Ctrl Pts',(9.96072433801779,9.33761180924535,7.48126572599483));
#94094=CARTESIAN_POINT('Ctrl Pts',(10.1454158537006,5.44905605214366,10.8018176189898));
#94095=CARTESIAN_POINT('Ctrl Pts',(10.3508522783911,-0.0259045708147128,
11.9726580271132));
#94096=CARTESIAN_POINT('Ctrl Pts',(10.535911563002,-4.95140312035918,10.9172233439656));
#94097=CARTESIAN_POINT('Ctrl Pts',(10.7211379748348,-9.00820528356076,7.92003054877835));
#94098=CARTESIAN_POINT('Ctrl Pts',(10.9374220425718,-11.8983876651759,2.78562722922065));
#94099=CARTESIAN_POINT('Ctrl Pts',(11.1848729346765,-11.7777413136033,-4.14068320944885));
#94100=CARTESIAN_POINT('Ctrl Pts',(11.4635980779861,-7.02331972060775,-10.338030997822));
#94101=CARTESIAN_POINT('Ctrl Pts',(11.74265928929,0.485771185227506,-12.5031515715995));
#94102=CARTESIAN_POINT('Ctrl Pts',(12.0220452423349,7.82452146813134,-9.78373091459582));
#94103=CARTESIAN_POINT('Ctrl Pts',(12.3017414264954,12.1176670139685,-3.22947077724254));
#94104=CARTESIAN_POINT('Ctrl Pts',(12.5817404915373,11.6811207583279,4.59955148712552));
#94105=CARTESIAN_POINT('Ctrl Pts',(12.8620270450134,6.67296756288785,10.6506950365554));
#94106=CARTESIAN_POINT('Ctrl Pts',(13.1114181050387,-0.10457717046341,12.3264734729167));
#94107=CARTESIAN_POINT('Ctrl Pts',(13.3298047978312,-5.80925739830131,10.6374828466507));
#94108=CARTESIAN_POINT('Ctrl Pts',(13.5171085156676,-9.67623713023754,7.31489439723108));
#94109=CARTESIAN_POINT('Ctrl Pts',(13.7045226807009,-11.8343851470158,2.68839440087991));
#94110=CARTESIAN_POINT('Ctrl Pts',(13.8920417432291,-11.9012035933258,-2.41678325350551));
#94111=CARTESIAN_POINT('Ctrl Pts',(14.079665958182,-9.85846808915857,-7.10106027918717));
#94112=CARTESIAN_POINT('Ctrl Pts',(14.2673878802831,-6.07020448910423,-10.5318302742615));
#94113=CARTESIAN_POINT('Ctrl Pts',(14.4552057276401,-1.20080043304805,-12.1025206353879));
#94114=CARTESIAN_POINT('Ctrl Pts',(14.6431142432908,3.8816049546317,-11.5313035488319));
#94115=CARTESIAN_POINT('Ctrl Pts',(14.8624426279901,9.0254261845754,-8.48686288050747));
#94116=CARTESIAN_POINT('Ctrl Pts',(15.0662215925831,11.7864106250798,-3.50019926818456));
#94117=CARTESIAN_POINT('Ctrl Pts',(15.254409406039,11.9202349594292,1.5765729310934));
#94118=CARTESIAN_POINT('Ctrl Pts',(15.4191235409337,10.6578227800216,5.83335525776536));
#94119=CARTESIAN_POINT('Ctrl Pts',(15.6074366748314,7.38808957059488,9.82399360787681));
#94120=CARTESIAN_POINT('Ctrl Pts',(15.8193743748441,2.05440533968246,12.1239164257433));
#94121=CARTESIAN_POINT('Ctrl Pts',(16.0313917910744,-3.73589016362928,11.717970713382));
#94122=CARTESIAN_POINT('Ctrl Pts',(16.267050002056,-9.26251206309682,8.36911230129259));
#94123=CARTESIAN_POINT('Ctrl Pts',(16.5263714569448,-12.533929235738,1.89081660411466));
#94124=CARTESIAN_POINT('Ctrl Pts',(16.8093751255442,-11.2186654351146,-5.92967881388903));
#94125=CARTESIAN_POINT('Ctrl Pts',(17.0688842231128,-5.98069892529497,-10.9674338194529));
#94126=CARTESIAN_POINT('Ctrl Pts',(17.3048617982993,0.344066224609658,-12.3144477215541));
#94127=CARTESIAN_POINT('Ctrl Pts',(17.5172733718789,5.95765915627426,-10.7876969598574));
#94128=CARTESIAN_POINT('Ctrl Pts',(17.7297418565277,10.2455913891075,-6.85024088753073));
#94129=CARTESIAN_POINT('Ctrl Pts',(17.9421831783442,12.248073460281,-1.38505961147241));
#94130=CARTESIAN_POINT('Ctrl Pts',(18.1547754227988,11.5188638260364,4.39096010934591));
#94131=CARTESIAN_POINT('Ctrl Pts',(18.3671125344183,8.21967595083557,9.1880203878024));
#94132=CARTESIAN_POINT('Ctrl Pts',(18.5799708194115,3.08654720046552,11.9359926983551));
#94133=CARTESIAN_POINT('Ctrl Pts',(18.7919954923611,-2.73535569069524,12.0215380695732));
#94134=CARTESIAN_POINT('Ctrl Pts',(19.0053084385149,-7.94711295728738,9.42520690240711));
#94135=CARTESIAN_POINT('Ctrl Pts',(19.2159056093561,-11.3857266012703,4.72718457448586));
#94136=CARTESIAN_POINT('Ctrl Pts',(19.4383538857774,-12.2844643908536,-1.02563854021835));
#94137=CARTESIAN_POINT('Ctrl Pts',(19.5755497693638,-10.4423848684627,-6.54989237074188));
#94138=CARTESIAN_POINT('Ctrl Pts',(19.7502330266567,-6.27044368623733,-10.6109788360224));
#94139=CARTESIAN_POINT('Ctrl Pts',(19.9067401471095,-0.700332527302415,
-12.304166099507));
#94140=CARTESIAN_POINT('Ctrl Pts',(20.0721200843413,5.02482750250949,-11.2515282704222));
#94141=CARTESIAN_POINT('Ctrl Pts',(20.2332449466593,9.62741902390977,-7.68867788673749));
#94142=CARTESIAN_POINT('Ctrl Pts',(20.3962864578522,12.0805747843324,-2.41184681685216));
#94143=CARTESIAN_POINT('Ctrl Pts',(20.5584408125953,11.8380006987581,3.40253336230924));
#94144=CARTESIAN_POINT('Ctrl Pts',(20.7209391746282,8.95366751262233,8.45314344278682));
#94145=CARTESIAN_POINT('Ctrl Pts',(20.8832633852329,4.07441140443369,11.6219108468804));
#94146=CARTESIAN_POINT('Ctrl Pts',(21.0455652300593,-1.7146252320768,12.1839430152868));
#94147=CARTESIAN_POINT('Ctrl Pts',(21.2079576291958,-7.11302875026615,10.0544459268831));
#94148=CARTESIAN_POINT('Ctrl Pts',(21.3934853478725,-11.4861546019893,4.98512765023302));
#94149=CARTESIAN_POINT('Ctrl Pts',(21.5257040221825,-12.1499364246399,0.288695447581215));
#94150=CARTESIAN_POINT('Ctrl Pts',(21.6019507193,-11.5961781364247,-2.52793074198454));
#94151=CARTESIAN_POINT('Ctrl Pts',(-0.185619006479058,10.0933261135196,
-2.22965916229763));
#94152=CARTESIAN_POINT('Ctrl Pts',(-0.117300790501088,10.5748062538398,
0.292199444285957));
#94153=CARTESIAN_POINT('Ctrl Pts',(-0.00302478330723105,9.99803717212611,
4.35034456802874));
#94154=CARTESIAN_POINT('Ctrl Pts',(0.159034371049183,6.18659475687002,8.78323627108909));
#94155=CARTESIAN_POINT('Ctrl Pts',(0.300544972038591,1.47700746620311,10.6342663436784));
#94156=CARTESIAN_POINT('Ctrl Pts',(0.442337090194551,-3.57821420110069,
10.1475684647875));
#94157=CARTESIAN_POINT('Ctrl Pts',(0.584195829308131,-7.84371227150242,
7.37625010341519));
#94158=CARTESIAN_POINT('Ctrl Pts',(0.72638210808798,-10.367739942029,2.95834583624723));
#94159=CARTESIAN_POINT('Ctrl Pts',(0.868398654429114,-10.5809430214755,
-2.13457721884431));
#94160=CARTESIAN_POINT('Ctrl Pts',(1.01134841234015,-8.43060470673339,-6.76121401375651));
#94161=CARTESIAN_POINT('Ctrl Pts',(1.15275825406684,-4.39155286462621,-9.88868216121412));
#94162=CARTESIAN_POINT('Ctrl Pts',(1.29806892103168,0.638793885868586,-10.8145395134698));
#94163=CARTESIAN_POINT('Ctrl Pts',(1.43573014356304,5.53815777824442,-9.32520081283725));
#94164=CARTESIAN_POINT('Ctrl Pts',(1.58954140736491,9.21275358259364,-5.75061203927714));
#94165=CARTESIAN_POINT('Ctrl Pts',(1.71047817919196,10.8366639978476,-0.88074887746556));
#94166=CARTESIAN_POINT('Ctrl Pts',(1.90724751534395,10.04431618838,4.21181408041434));
#94167=CARTESIAN_POINT('Ctrl Pts',(2.09324214724154,7.00555778279355,8.35618508415984));
#94168=CARTESIAN_POINT('Ctrl Pts',(2.30311330738613,1.87705741752283,10.9229722067622));
#94169=CARTESIAN_POINT('Ctrl Pts',(2.5332257405624,-4.54561841310713,10.3217734068532));
#94170=CARTESIAN_POINT('Ctrl Pts',(2.78536647948873,-9.81351567061726,5.61618222831888));
#94171=CARTESIAN_POINT('Ctrl Pts',(3.03782338103716,-11.2494025829444,-1.3090245995979));
#94172=CARTESIAN_POINT('Ctrl Pts',(3.29095008907448,-8.29511055112181,-7.75122091179339));
#94173=CARTESIAN_POINT('Ctrl Pts',(3.54458903946069,-2.07331878640508,-11.1892909019698));
#94174=CARTESIAN_POINT('Ctrl Pts',(3.77056982278458,4.19665237318481,-10.3559315238114));
#94175=CARTESIAN_POINT('Ctrl Pts',(3.96866456430814,8.45273696730399,-7.03593621691386));
#94176=CARTESIAN_POINT('Ctrl Pts',(4.13871597273587,10.6149061400342,-2.94502419387331));
#94177=CARTESIAN_POINT('Ctrl Pts',(4.33740334598655,10.9566874777779,2.45929408029225));
#94178=CARTESIAN_POINT('Ctrl Pts',(4.56489938943493,8.09225092751257,8.14593648910699));
#94179=CARTESIAN_POINT('Ctrl Pts',(4.82140674035802,1.67392883349891,11.3844888654692));
#94180=CARTESIAN_POINT('Ctrl Pts',(5.0784905353754,-5.42364562133815,10.1772068941644));
#94181=CARTESIAN_POINT('Ctrl Pts',(5.336151281316,-10.4315834824905,4.9793900503427));
#94182=CARTESIAN_POINT('Ctrl Pts',(5.59439033959415,-11.3747242087523,-2.19301745790991));
#94183=CARTESIAN_POINT('Ctrl Pts',(5.85320774256082,-7.86907925564315,-8.53689977516254));
#94184=CARTESIAN_POINT('Ctrl Pts',(6.11260412203838,-1.26235022387817,-11.5692530353362));
#94185=CARTESIAN_POINT('Ctrl Pts',(6.34369227098713,5.06919294204147,-10.2415176535993));
#94186=CARTESIAN_POINT('Ctrl Pts',(6.54627005947845,9.15551290375705,-6.53203957187647));
#94187=CARTESIAN_POINT('Ctrl Pts',(6.72016445010838,11.0505027548576,-2.19287267091472));
#94188=CARTESIAN_POINT('Ctrl Pts',(6.89431529161194,10.9882369915932,2.54767804033175));
#94189=CARTESIAN_POINT('Ctrl Pts',(7.08810135472563,8.76241579151075,7.33582397855815));
#94190=CARTESIAN_POINT('Ctrl Pts',(7.2628065037542,4.88176934217404,10.224447229933));
#94191=CARTESIAN_POINT('Ctrl Pts',(7.43776736394009,0.281512668682108,11.2268839659177));
#94192=CARTESIAN_POINT('Ctrl Pts',(7.59347538540535,-3.91850390490377,10.6525957197084));
#94193=CARTESIAN_POINT('Ctrl Pts',(7.76890244595317,-7.96078056106154,8.1068360055412));
#94194=CARTESIAN_POINT('Ctrl Pts',(7.97386284239987,-11.0540605057285,3.46069251756181));
#94195=CARTESIAN_POINT('Ctrl Pts',(8.20852292562262,-11.4323534240288,-3.10028647612775));
#94196=CARTESIAN_POINT('Ctrl Pts',(8.42898801261747,-8.04427720537063,-8.26450393249604));
#94197=CARTESIAN_POINT('Ctrl Pts',(8.60564238755027,-3.89233801355417,-10.5975657495071));
#94198=CARTESIAN_POINT('Ctrl Pts',(8.78248401029939,0.784991099698641,-11.5398447216046));
#94199=CARTESIAN_POINT('Ctrl Pts',(8.97436271810468,5.94350829980616,-10.0521140215687));
#94200=CARTESIAN_POINT('Ctrl Pts',(9.18136388578912,9.82591071360329,-5.96135288429516));
#94201=CARTESIAN_POINT('Ctrl Pts',(9.35903887805549,11.4259511373913,-1.39532146785222));
#94202=CARTESIAN_POINT('Ctrl Pts',(9.51718886382132,11.046839530257,2.89306782909364));
#94203=CARTESIAN_POINT('Ctrl Pts',(9.69531065618581,9.00905509810931,7.23148778947319));
#94204=CARTESIAN_POINT('Ctrl Pts',(9.87367490207668,5.2539372050763,10.4385707953799));
#94205=CARTESIAN_POINT('Ctrl Pts',(10.0721679770359,-0.0359846706333819,
11.5700988759545));
#94206=CARTESIAN_POINT('Ctrl Pts',(10.2510516766973,-4.79716825546636,10.5500969177149));
#94207=CARTESIAN_POINT('Ctrl Pts',(10.4301715895454,-8.72039401479544,7.65185637941947));
#94208=CARTESIAN_POINT('Ctrl Pts',(10.6394202628606,-11.5168011966333,2.68460959360604));
#94209=CARTESIAN_POINT('Ctrl Pts',(10.8789516349422,-11.4007138619713,-4.02009897255846));
#94210=CARTESIAN_POINT('Ctrl Pts',(11.1489446719379,-6.79589583934775,-10.0238491212784));
#94211=CARTESIAN_POINT('Ctrl Pts',(11.4194521684921,0.482857387799818,-12.1234364564696));
#94212=CARTESIAN_POINT('Ctrl Pts',(11.6904683222343,7.60210633467787,-9.48629381739815));
#94213=CARTESIAN_POINT('Ctrl Pts',(11.9619844318012,11.7704714210056,-3.12417202096832));
#94214=CARTESIAN_POINT('Ctrl Pts',(12.2339955399624,11.3472899568952,4.48161077014586));
#94215=CARTESIAN_POINT('Ctrl Pts',(12.5064934469842,6.47900806171408,10.3652310553541));
#94216=CARTESIAN_POINT('Ctrl Pts',(12.7491382824443,-0.115092593871167,
11.9965207438775));
#94217=CARTESIAN_POINT('Ctrl Pts',(12.9617604208479,-5.66932712881705,10.3524164038613));
#94218=CARTESIAN_POINT('Ctrl Pts',(13.1442139405268,-9.43637405277016,7.11605841772142));
#94219=CARTESIAN_POINT('Ctrl Pts',(13.3268721736923,-11.5400301082066,2.60705350414733));
#94220=CARTESIAN_POINT('Ctrl Pts',(13.5097329412205,-11.6054789249675,-2.3713096424544));
#94221=CARTESIAN_POINT('Ctrl Pts',(13.6927926573215,-9.61268254417223,-6.94178412299867));
#94222=CARTESIAN_POINT('Ctrl Pts',(13.8760493751974,-5.91470652543587,-10.2911833251264));
#94223=CARTESIAN_POINT('Ctrl Pts',(14.0595003754106,-1.15857060513477,-11.8256418676525));
#94224=CARTESIAN_POINT('Ctrl Pts',(14.2431438187993,3.80852772916814,-11.2676768952274));
#94225=CARTESIAN_POINT('Ctrl Pts',(14.4576147034959,8.83860998669587,-8.29097831594669));
#94226=CARTESIAN_POINT('Ctrl Pts',(14.6570160689187,11.5409394968827,-3.41172603447321));
#94227=CARTESIAN_POINT('Ctrl Pts',(14.8412851520698,11.6721745564983,1.55937792284147));
#94228=CARTESIAN_POINT('Ctrl Pts',(15.0026382754732,10.4356527910619,5.72934455817101));
#94229=CARTESIAN_POINT('Ctrl Pts',(15.1872075685466,7.23121856863992,9.64091306653126));
#94230=CARTESIAN_POINT('Ctrl Pts',(15.3950684928386,2.00027267799374,11.8970379868734));
#94231=CARTESIAN_POINT('Ctrl Pts',(15.6031452748645,-3.68246582260826,11.4990590640796));
#94232=CARTESIAN_POINT('Ctrl Pts',(15.8345765195311,-9.11024577131713,8.2107324415602));
#94233=CARTESIAN_POINT('Ctrl Pts',(16.0894467450161,-12.326401693567,1.84403017349057));
#94234=CARTESIAN_POINT('Ctrl Pts',(16.3678445378864,-11.0336854894674,-5.84936519393046));
#94235=CARTESIAN_POINT('Ctrl Pts',(16.6233577253131,-5.87699554144271,-10.8103679738959));
#94236=CARTESIAN_POINT('Ctrl Pts',(16.8558911710288,0.355399540435648,-12.1382610506978));
#94237=CARTESIAN_POINT('Ctrl Pts',(17.0653460588931,5.89099933966217,-10.6332079424033));
#94238=CARTESIAN_POINT('Ctrl Pts',(17.2750019757892,10.1225327187077,-6.74818253139266));
#94239=CARTESIAN_POINT('Ctrl Pts',(17.4847784853901,12.1003364385946,-1.35176206524406));
#94240=CARTESIAN_POINT('Ctrl Pts',(17.6948470084932,11.3802690665637,4.35595591482899));
#94241=CARTESIAN_POINT('Ctrl Pts',(17.9048201429876,8.11824693147351,9.09954721971294));
#94242=CARTESIAN_POINT('Ctrl Pts',(18.1154347704745,3.03915862004288,11.8196545783736));
#94243=CARTESIAN_POINT('Ctrl Pts',(18.325423469146,-2.72613110987367,11.9038913215774));
#94244=CARTESIAN_POINT('Ctrl Pts',(18.5367299625652,-7.89050873461128,9.33351651045655));
#94245=CARTESIAN_POINT('Ctrl Pts',(18.7457054460238,-11.3012202672818,4.67113223677404));
#94246=CARTESIAN_POINT('Ctrl Pts',(18.9662251567336,-12.193620628485,-1.03097537473009));
#94247=CARTESIAN_POINT('Ctrl Pts',(19.1024647483826,-10.3645021296875,-6.51607209457868));
#94248=CARTESIAN_POINT('Ctrl Pts',(19.2760119384225,-6.22017837815075,-10.5517199199323));
#94249=CARTESIAN_POINT('Ctrl Pts',(19.4315873565836,-0.683226350082178,
-12.2347432990342));
#94250=CARTESIAN_POINT('Ctrl Pts',(19.5960678744438,5.0109095220934,-11.1884067790233));
#94251=CARTESIAN_POINT('Ctrl Pts',(19.7564113157442,9.59142240873504,-7.64306850438877));
#94252=CARTESIAN_POINT('Ctrl Pts',(19.9187466440103,12.0343012504836,-2.3892255621501));
#94253=CARTESIAN_POINT('Ctrl Pts',(20.0802909525939,11.793043994749,3.4033212507376));
#94254=CARTESIAN_POINT('Ctrl Pts',(20.2422658654157,8.91830151793921,8.43786839370665));
#94255=CARTESIAN_POINT('Ctrl Pts',(20.4041575536249,4.05224680745339,11.5985615600057));
#94256=CARTESIAN_POINT('Ctrl Pts',(20.5661165762954,-1.72455343266205,12.1597439014428));
#94257=CARTESIAN_POINT('Ctrl Pts',(20.7282547450467,-7.11467144874381,10.0339938166866));
#94258=CARTESIAN_POINT('Ctrl Pts',(20.9135960702887,-11.4837610123811,4.96998028147232));
#94259=CARTESIAN_POINT('Ctrl Pts',(21.0457773344246,-12.1478998213886,0.275052131649602));
#94260=CARTESIAN_POINT('Ctrl Pts',(21.121985606656,-11.5941213892729,-2.54022968745642));
#94261=CARTESIAN_POINT('Ctrl Pts',(0.0468883190715043,9.87513244460898,
-2.19475014191929));
#94262=CARTESIAN_POINT('Ctrl Pts',(0.114030713978885,10.3462550411863,0.283509053294733));
#94263=CARTESIAN_POINT('Ctrl Pts',(0.225696291009577,9.78169823289018,4.24859024618672));
#94264=CARTESIAN_POINT('Ctrl Pts',(0.38424441193138,6.05401391249468,8.58604538141497));
#94265=CARTESIAN_POINT('Ctrl Pts',(0.522572982615551,1.4493723242407,10.39438467727));
#94266=CARTESIAN_POINT('Ctrl Pts',(0.661176886801409,-3.49174235122776,
9.91912528151));
#94267=CARTESIAN_POINT('Ctrl Pts',(0.799793926350337,-7.65981690416216,
7.21058321160161));
#94268=CARTESIAN_POINT('Ctrl Pts',(0.938699675819258,-10.1254171052646,
2.89475805670008));
#94269=CARTESIAN_POINT('Ctrl Pts',(1.0774028348938,-10.3334998105185,-2.07940899395324));
#94270=CARTESIAN_POINT('Ctrl Pts',(1.21698159467311,-8.23375157199671,-6.59680525048484));
#94271=CARTESIAN_POINT('Ctrl Pts',(1.35502420317193,-4.29082503876726,-9.6497000433534));
#94272=CARTESIAN_POINT('Ctrl Pts',(1.49683806736127,0.61845798375215,-10.5530464314786));
#94273=CARTESIAN_POINT('Ctrl Pts',(1.63115645888639,5.39880279485396,-9.09992044033476));
#94274=CARTESIAN_POINT('Ctrl Pts',(1.78119823087382,8.98311851124421,-5.61262810702319));
#94275=CARTESIAN_POINT('Ctrl Pts',(1.89914716909541,10.5668634406556,-0.863359736108471));
#94276=CARTESIAN_POINT('Ctrl Pts',(2.09092707093951,9.79411297578629,4.09974224607044));
#94277=CARTESIAN_POINT('Ctrl Pts',(2.27227504460956,6.83178142521456,8.1407345402975));
#94278=CARTESIAN_POINT('Ctrl Pts',(2.47677050336701,1.8341135810532,10.6412176269922));
#94279=CARTESIAN_POINT('Ctrl Pts',(2.70096262760981,-4.42295544725151,10.0555858579246));
#94280=CARTESIAN_POINT('Ctrl Pts',(2.94651424708369,-9.55296973843427,5.47242477730225));
#94281=CARTESIAN_POINT('Ctrl Pts',(3.19230186483792,-10.9506117802351,-1.26972603849257));
#94282=CARTESIAN_POINT('Ctrl Pts',(3.43866776969254,-8.07492744395638,-7.53972790059379));
#94283=CARTESIAN_POINT('Ctrl Pts',(3.68546398000364,-2.02091240779182,-10.8847378569879));
#94284=CARTESIAN_POINT('Ctrl Pts',(3.90529255407266,4.07825689510438,-10.0738326461541));
#94285=CARTESIAN_POINT('Ctrl Pts',(4.09795042603787,8.21745567231149,-6.84490401927142));
#94286=CARTESIAN_POINT('Ctrl Pts',(4.26330957581834,10.319891481976,-2.86685448795266));
#94287=CARTESIAN_POINT('Ctrl Pts',(4.45648701258071,10.6521098287859,2.3875741469057));
#94288=CARTESIAN_POINT('Ctrl Pts',(4.67763710085154,7.86743005469358,7.91545385483815));
#94289=CARTESIAN_POINT('Ctrl Pts',(4.926939430199,1.62934305813083,11.0628341733645));
#94290=CARTESIAN_POINT('Ctrl Pts',(5.17675887001051,-5.26758965195953,9.8894979002806));
#94291=CARTESIAN_POINT('Ctrl Pts',(5.4270982839676,-10.133076375223,4.8392917781549));
#94292=CARTESIAN_POINT('Ctrl Pts',(5.67796487531094,-11.0491418208461,-2.12831927355943));
#94293=CARTESIAN_POINT('Ctrl Pts',(5.92936241374252,-7.64390736818979,-8.29022018966899));
#94294=CARTESIAN_POINT('Ctrl Pts',(6.18129477974471,-1.22728028249969,-11.23520053354));
#94295=CARTESIAN_POINT('Ctrl Pts',(6.40571582591634,4.92150724239765,-9.9457051776774));
#94296=CARTESIAN_POINT('Ctrl Pts',(6.60243453809443,8.88960333168464,-6.34350746355418));
#94297=CARTESIAN_POINT('Ctrl Pts',(6.77129389446513,10.7296919156058,-2.1300022505958));
#94298=CARTESIAN_POINT('Ctrl Pts',(6.94039652441011,10.6692178625933,2.47310728894808));
#94299=CARTESIAN_POINT('Ctrl Pts',(7.12855930053127,8.50797601358858,7.12228923056046));
#94300=CARTESIAN_POINT('Ctrl Pts',(7.29819263731241,4.7400095745379,9.92702859165824));
#94301=CARTESIAN_POINT('Ctrl Pts',(7.46807153457936,0.273380586784091,10.9003466502549));
#94302=CARTESIAN_POINT('Ctrl Pts',(7.61925924909045,-3.80466580324696,10.3427388138934));
#94303=CARTESIAN_POINT('Ctrl Pts',(7.78959139326839,-7.72954127611913,7.87093104257765));
#94304=CARTESIAN_POINT('Ctrl Pts',(7.98860172481287,-10.7330126993619,3.35968762659343));
#94305=CARTESIAN_POINT('Ctrl Pts',(8.2164580403836,-11.1003918261383,-3.01100747504486));
#94306=CARTESIAN_POINT('Ctrl Pts',(8.43054075733716,-7.81046194370647,-8.02571834499739));
#94307=CARTESIAN_POINT('Ctrl Pts',(8.60208730154287,-3.77859473411447,-10.2913249526089));
#94308=CARTESIAN_POINT('Ctrl Pts',(8.77382123972295,0.763621927493125,-11.2064020023924));
#94309=CARTESIAN_POINT('Ctrl Pts',(8.96017336877873,5.77352570649464,-9.76160039398119));
#94310=CARTESIAN_POINT('Ctrl Pts',(9.16122393237721,9.54433910015271,-5.78846853353381));
#94311=CARTESIAN_POINT('Ctrl Pts',(9.33380383741733,11.0985302356744,-1.35340417939127));
#94312=CARTESIAN_POINT('Ctrl Pts',(9.48743167162671,10.7302913508911,2.81235066996444));
#94313=CARTESIAN_POINT('Ctrl Pts',(9.66047154404099,8.75067522278089,7.02698063644771));
#94314=CARTESIAN_POINT('Ctrl Pts',(9.83376200706454,5.10244018493771,10.1428909049288));
#94315=CARTESIAN_POINT('Ctrl Pts',(10.0266323623159,-0.0375966260133391,
11.2424270292935));
#94316=CARTESIAN_POINT('Ctrl Pts',(10.200465347967,-4.66435103389636,10.2512760419087));
#94317=CARTESIAN_POINT('Ctrl Pts',(10.3745490662983,-8.47729079196604,7.43459200187802));
#94318=CARTESIAN_POINT('Ctrl Pts',(10.5779374592024,-11.1954312635547,2.60651789413556));
#94319=CARTESIAN_POINT('Ctrl Pts',(10.8107978298792,-11.0827892717403,-3.91143012134676));
#94320=CARTESIAN_POINT('Ctrl Pts',(11.0733244705727,-6.60553148650756,-9.74928532905834));
#94321=CARTESIAN_POINT('Ctrl Pts',(11.3364087177861,0.473374528820086,-11.7915043150319));
#94322=CARTESIAN_POINT('Ctrl Pts',(11.6000483863509,7.39892601293791,-9.22641799008054));
#94323=CARTESIAN_POINT('Ctrl Pts',(11.8642402274303,11.4550878200309,-3.03610638012168));
#94324=CARTESIAN_POINT('Ctrl Pts',(12.1289822792327,11.0435290122831,4.36640970745214));
#94325=CARTESIAN_POINT('Ctrl Pts',(12.3942707801871,6.30432840493419,10.0945732748139));
#94326=CARTESIAN_POINT('Ctrl Pts',(12.6305653527167,-0.117105282786375,
11.6834591349301));
#94327=CARTESIAN_POINT('Ctrl Pts',(12.8376729609091,-5.52732785933807,10.0821181565203));
#94328=CARTESIAN_POINT('Ctrl Pts',(13.0154321048852,-9.19750920314661,6.92911563257701));
#94329=CARTESIAN_POINT('Ctrl Pts',(13.1934285394712,-11.2475761619162,2.53524663869076));
#94330=CARTESIAN_POINT('Ctrl Pts',(13.3716607445812,-11.3114796153966,-2.31709443318142));
#94331=CARTESIAN_POINT('Ctrl Pts',(13.5501275727524,-9.36879757076698,-6.77293750521516));
#94332=CARTESIAN_POINT('Ctrl Pts',(13.7288272740876,-5.76286586238848,-10.0391279784165));
#94333=CARTESIAN_POINT('Ctrl Pts',(13.9077586256967,-1.12395467957662,-11.5359049681128));
#94334=CARTESIAN_POINT('Ctrl Pts',(14.086920220302,3.72193056449534,-10.991676187186));
#94335=CARTESIAN_POINT('Ctrl Pts',(14.2962084781089,8.63052987121803,-8.08705962566316));
#94336=CARTESIAN_POINT('Ctrl Pts',(14.4908538017284,11.2686759469096,-3.32435546363631));
#94337=CARTESIAN_POINT('Ctrl Pts',(14.6707791287713,11.3969035793279,1.52957519084057));
#94338=CARTESIAN_POINT('Ctrl Pts',(14.8283599138058,10.1893571480635,5.60205724013665));
#94339=CARTESIAN_POINT('Ctrl Pts',(15.0086594519658,7.05920045221355,9.4232425043886));
#94340=CARTESIAN_POINT('Ctrl Pts',(15.211773956704,1.94778936772532,11.6280440864309));
#94341=CARTESIAN_POINT('Ctrl Pts',(15.4151630308288,-3.60693517107769,11.2392351797925));
#94342=CARTESIAN_POINT('Ctrl Pts',(15.6414526624567,-8.91423786935106,8.02419552881062));
#94343=CARTESIAN_POINT('Ctrl Pts',(15.8907548211699,-12.0605597097748,1.79679831518536));
#94344=CARTESIAN_POINT('Ctrl Pts',(16.163191580604,-10.7960738679334,-5.73193800227007));
#94345=CARTESIAN_POINT('Ctrl Pts',(16.41334739475,-5.74785323359727,-10.5893059881456));
#94346=CARTESIAN_POINT('Ctrl Pts',(16.6410977293422,0.356304475045441,-11.8901509760637));
#94347=CARTESIAN_POINT('Ctrl Pts',(16.8463169597766,5.78001582433962,-10.4157688994121));
#94348=CARTESIAN_POINT('Ctrl Pts',(17.0518065043981,9.92763508001442,-6.60811463582451));
#94349=CARTESIAN_POINT('Ctrl Pts',(17.2574901073631,11.8670731514498,-1.31710918465926));
#94350=CARTESIAN_POINT('Ctrl Pts',(17.4635339299854,11.161059099898,4.28138607926673));
#94351=CARTESIAN_POINT('Ctrl Pts',(17.6695666131704,7.96049490837238,8.93590314995754));
#94352=CARTESIAN_POINT('Ctrl Pts',(17.8762947475351,2.97510156392891,11.6064115606909));
#94353=CARTESIAN_POINT('Ctrl Pts',(18.0825158331318,-2.68633915899874,11.6888620853711));
#94354=CARTESIAN_POINT('Ctrl Pts',(18.2900516890882,-7.75946435507434,9.16520199964202));
#94355=CARTESIAN_POINT('Ctrl Pts',(18.4954960228899,-11.1117450252379,4.58131790262806));
#94356=CARTESIAN_POINT('Ctrl Pts',(18.7121686537848,-11.9893823770525,-1.02085731366645));
#94357=CARTESIAN_POINT('Ctrl Pts',(18.8461604978706,-10.1905191614686,-6.4150574092785));
#94358=CARTESIAN_POINT('Ctrl Pts',(19.0168888857437,-6.11378020764086,-10.3857054152766));
#94359=CARTESIAN_POINT('Ctrl Pts',(19.1699862042231,-0.665040585986461,
-12.0418702738763));
#94360=CARTESIAN_POINT('Ctrl Pts',(19.3318944658821,4.94010577090635,-11.0122286489555));
#94361=CARTESIAN_POINT('Ctrl Pts',(19.4897842633542,9.45065765391111,-7.52127249356902));
#94362=CARTESIAN_POINT('Ctrl Pts',(19.6496837846903,11.8570837283046,-2.34636545288141));
#94363=CARTESIAN_POINT('Ctrl Pts',(19.8088568555673,11.6195942596276,3.36123155851592));
#94364=CARTESIAN_POINT('Ctrl Pts',(19.9685059338027,8.78633570480602,8.32349554013287));
#94365=CARTESIAN_POINT('Ctrl Pts',(20.1281223497918,3.98869219334678,11.4402304690933));
#94366=CARTESIAN_POINT('Ctrl Pts',(20.2878661710919,-1.70886274984082,11.9935718342937));
#94367=CARTESIAN_POINT('Ctrl Pts',(20.4478171504923,-7.02689664581043,9.89725056153651));
#94368=CARTESIAN_POINT('Ctrl Pts',(20.6307713581253,-11.3391595667794,4.89815896715976));
#94369=CARTESIAN_POINT('Ctrl Pts',(20.7612036626925,-11.9952158857887,0.265588695805443));
#94370=CARTESIAN_POINT('Ctrl Pts',(20.8366222476259,-11.448353871513,-2.52040522030094));
#94371=CARTESIAN_POINT('Ctrl Pts',(0.183614459124478,9.79786316135237,-2.18390363605074));
#94372=CARTESIAN_POINT('Ctrl Pts',(0.250341770018844,10.2652923627661,0.278931271446855));
#94373=CARTESIAN_POINT('Ctrl Pts',(0.361079149189646,9.70507677462218,4.21096420845386));
#94374=CARTESIAN_POINT('Ctrl Pts',(0.518366888107835,6.00740767582931,8.51416777379075));
#94375=CARTESIAN_POINT('Ctrl Pts',(0.655542474297922,1.44074519809565,10.3070121042654));
#94376=CARTESIAN_POINT('Ctrl Pts',(0.792981618713115,-3.4587220983823,9.83588618154369));
#94377=CARTESIAN_POINT('Ctrl Pts',(0.930404605240617,-7.59092267674199,
7.15040523375962));
#94378=CARTESIAN_POINT('Ctrl Pts',(1.06809234888974,-10.0348185367602,2.87241801630468));
#94379=CARTESIAN_POINT('Ctrl Pts',(1.20555599039251,-10.2409431246026,-2.05737109410186));
#94380=CARTESIAN_POINT('Ctrl Pts',(1.34386398892466,-8.16021043925077,-6.53361307400495));
#94381=CARTESIAN_POINT('Ctrl Pts',(1.48062853400263,-4.25370717449432,-9.55820608939274));
#94382=CARTESIAN_POINT('Ctrl Pts',(1.62110525372889,0.609335041197672,-10.4528924440852));
#94383=CARTESIAN_POINT('Ctrl Pts',(1.75413692600142,5.34391651279451,-9.01369845472587));
#94384=CARTESIAN_POINT('Ctrl Pts',(1.90271849574803,8.89323649719505,-5.5600974036933));
#94385=CARTESIAN_POINT('Ctrl Pts',(2.01950257907449,10.461335073174,-0.857833757076778));
#94386=CARTESIAN_POINT('Ctrl Pts',(2.20930202147911,9.69621420838626,4.05382364169921));
#94387=CARTESIAN_POINT('Ctrl Pts',(2.38882434817707,6.76402558143954,8.05427559657762));
#94388=CARTESIAN_POINT('Ctrl Pts',(2.5911696751643,1.81848501841292,10.528109479656));
#94389=CARTESIAN_POINT('Ctrl Pts',(2.81298349260819,-4.37201424850356,9.94872151500545));
#94390=CARTESIAN_POINT('Ctrl Pts',(3.05585519071514,-9.4459783465168,5.41513931684729));
#94391=CARTESIAN_POINT('Ctrl Pts',(3.29891245926674,-10.8278396352703,-1.25208481677035));
#94392=CARTESIAN_POINT('Ctrl Pts',(3.54248087609222,-7.98456011415915,-7.45088636332916));
#94393=CARTESIAN_POINT('Ctrl Pts',(3.78642356161324,-2.00041219665082,-10.756998482402));
#94394=CARTESIAN_POINT('Ctrl Pts',(4.00366193024937,4.02691199090365,-9.95545715254609));
#94395=CARTESIAN_POINT('Ctrl Pts',(4.1940202968856,8.11665682827487,-6.76499932942405));
#94396=CARTESIAN_POINT('Ctrl Pts',(4.3573838136257,10.1936786032613,-2.83492279490684));
#94397=CARTESIAN_POINT('Ctrl Pts',(4.54820422110693,10.5217640364167,2.35542955113606));
#94398=CARTESIAN_POINT('Ctrl Pts',(4.76662107188633,7.7713273867228,7.81493817752817));
#94399=CARTESIAN_POINT('Ctrl Pts',(5.01279825332115,1.6113145881985,10.9227010562467));
#94400=CARTESIAN_POINT('Ctrl Pts',(5.25944392263343,-5.19799627007342,9.76407920684044));
#94401=CARTESIAN_POINT('Ctrl Pts',(5.50656218450572,-10.0007734626784,4.77870524483264));
#94402=CARTESIAN_POINT('Ctrl Pts',(5.75416271454751,-10.9047480542855,-2.09824403734041));
#94403=CARTESIAN_POINT('Ctrl Pts',(6.00225064241072,-7.54418842815771,-8.17897689802922));
#94404=CARTESIAN_POINT('Ctrl Pts',(6.25083187444897,-1.21282426517761,-11.0846551043006));
#94405=CARTESIAN_POINT('Ctrl Pts',(6.47223861252284,4.85337527232899,-9.81235965589673));
#94406=CARTESIAN_POINT('Ctrl Pts',(6.66629611401229,8.76777044247514,-6.25884918518984));
#94407=CARTESIAN_POINT('Ctrl Pts',(6.8328580147061,10.5827983584686,-2.10264444945471));
#94408=CARTESIAN_POINT('Ctrl Pts',(6.99964746572987,10.5231160301507,2.43751391214038));
#94409=CARTESIAN_POINT('Ctrl Pts',(7.18522401361308,8.39154110993935,7.02279159226047));
#94410=CARTESIAN_POINT('Ctrl Pts',(7.35251256900072,4.67561428720135,9.7887253479214));
#94411=CARTESIAN_POINT('Ctrl Pts',(7.52003349787157,0.270973981687257,10.7485202607095));
#94412=CARTESIAN_POINT('Ctrl Pts',(7.66911434284302,-3.75025726686191,10.19865478183));
#94413=CARTESIAN_POINT('Ctrl Pts',(7.83706491325344,-7.62024552686739,7.76137857280017));
#94414=CARTESIAN_POINT('Ctrl Pts',(8.03328290043577,-10.5815581157576,3.31340924681337));
#94415=CARTESIAN_POINT('Ctrl Pts',(8.25792683192658,-10.9436830883588,-2.9675090618203));
#94416=CARTESIAN_POINT('Ctrl Pts',(8.46897913755438,-7.70027205447012,-7.91121797030631));
#94417=CARTESIAN_POINT('Ctrl Pts',(8.63809112468196,-3.7256112018197,-10.1446667494925));
#94418=CARTESIAN_POINT('Ctrl Pts',(8.80738397054104,0.752049767529649,-11.0467272685672));
#94419=CARTESIAN_POINT('Ctrl Pts',(8.99107917523528,5.69053692893971,-9.62248736715413));
#94420=CARTESIAN_POINT('Ctrl Pts',(9.1892589915876,9.40750408742455,-5.70607502743658));
#94421=CARTESIAN_POINT('Ctrl Pts',(9.35937116238761,10.9394620207273,-1.33441905354762));
#94422=CARTESIAN_POINT('Ctrl Pts',(9.51079897972392,10.5764897772339,2.77169008628882));
#94423=CARTESIAN_POINT('Ctrl Pts',(9.68135954194658,8.62523117889842,6.92593653995051));
#94424=CARTESIAN_POINT('Ctrl Pts',(9.85216535947771,5.02929449040856,9.99716749705792));
#94425=CARTESIAN_POINT('Ctrl Pts',(10.0422684509943,-0.0370046278410104,
11.0809239533146));
#94426=CARTESIAN_POINT('Ctrl Pts',(10.2136076308811,-4.59738656225664,10.1039913431277));
#94427=CARTESIAN_POINT('Ctrl Pts',(10.3851935207641,-8.35562322052339,7.32771401866009));
#94428=CARTESIAN_POINT('Ctrl Pts',(10.5856653585996,-11.0347880660269,2.56887395258143));
#94429=CARTESIAN_POINT('Ctrl Pts',(10.8151879901628,-10.9237726058889,-3.8556653985514));
#94430=CARTESIAN_POINT('Ctrl Pts',(11.0739580396521,-6.5106008392871,-9.61000610749268));
#94431=CARTESIAN_POINT('Ctrl Pts',(11.3332851299844,0.467209227920453,-11.6230950570897));
#94432=CARTESIAN_POINT('Ctrl Pts',(11.5931693281801,7.2941286449926,-9.09458958873076));
#94433=CARTESIAN_POINT('Ctrl Pts',(11.853609980442,11.2927459882514,-2.99220026576765));
#94434=CARTESIAN_POINT('Ctrl Pts',(12.1146065789635,10.8870722493502,4.30559358746303));
#94435=CARTESIAN_POINT('Ctrl Pts',(12.3761579386682,6.21469160094993,9.95311235977421));
#94436=CARTESIAN_POINT('Ctrl Pts',(12.6091398388233,-0.116703708482184,
11.5197928369494));
#94437=CARTESIAN_POINT('Ctrl Pts',(12.8133567685166,-5.45142549612194,9.94083145824057));
#94438=CARTESIAN_POINT('Ctrl Pts',(12.9886444160827,-9.07059415929487,6.83168724086131));
#94439=CARTESIAN_POINT('Ctrl Pts',(13.1641760934311,-11.092299460829,2.4986734042833));
#94440=CARTESIAN_POINT('Ctrl Pts',(13.3399509622567,-11.1553520037565,-2.28676417024083));
#94441=CARTESIAN_POINT('Ctrl Pts',(13.5159684793945,-9.23936112946262,-6.68146663577346));
#94442=CARTESIAN_POINT('Ctrl Pts',(13.6922275712029,-5.68270256836087,-9.90307032808977));
#94443=CARTESIAN_POINT('Ctrl Pts',(13.8687275286725,-1.10683977756436,-11.3795432290739));
#94444=CARTESIAN_POINT('Ctrl Pts',(14.0454674390564,3.67354689666366,-10.8427052739739));
#94445=CARTESIAN_POINT('Ctrl Pts',(14.2519425858938,8.51618802247031,-7.977176725935));
#94446=CARTESIAN_POINT('Ctrl Pts',(14.4439915267229,11.1192240057796,-3.27805817500437));
#94447=CARTESIAN_POINT('Ctrl Pts',(14.6215329808132,11.2457792395615,1.51156293289995));
#94448=CARTESIAN_POINT('Ctrl Pts',(14.7770361230669,10.0541750259763,5.53035051060673));
#94449=CARTESIAN_POINT('Ctrl Pts',(14.9549735676819,6.965075696007,9.30150472580482));
#94450=CARTESIAN_POINT('Ctrl Pts',(15.1554478199515,1.92014154542388,11.4777065223719));
#94451=CARTESIAN_POINT('Ctrl Pts',(15.3562146123695,-3.56296549636649,11.0939794920203));
#94452=CARTESIAN_POINT('Ctrl Pts',(15.5796118099573,-8.80245651644644,7.92011556461129));
#94453=CARTESIAN_POINT('Ctrl Pts',(15.8257599378043,-11.9091213200236,1.77158588855571));
#94454=CARTESIAN_POINT('Ctrl Pts',(16.0947928420177,-10.6606265159978,-5.66310190677918));
#94455=CARTESIAN_POINT('Ctrl Pts',(16.3418651896297,-5.67477284967232,-10.460720415196));
#94456=CARTESIAN_POINT('Ctrl Pts',(16.5668411838028,0.35500497682303,-11.7458113053674));
#94457=CARTESIAN_POINT('Ctrl Pts',(16.7695877632996,5.7133734584233,-10.2892834180772));
#94458=CARTESIAN_POINT('Ctrl Pts',(16.9726287036363,9.81162565530563,-6.52706848478553));
#94459=CARTESIAN_POINT('Ctrl Pts',(17.175890110972,11.7283013091856,-1.29843299398321));
#94460=CARTESIAN_POINT('Ctrl Pts',(17.3795355657123,11.0306030975541,4.23493323563435));
#94461=CARTESIAN_POINT('Ctrl Pts',(17.5832017988026,7.86690031490684,8.83595145758763));
#94462=CARTESIAN_POINT('Ctrl Pts',(17.7875808547236,2.93815531618296,11.476341011785));
#94463=CARTESIAN_POINT('Ctrl Pts',(17.9915008910348,-2.65993296615087,11.5577566949746));
#94464=CARTESIAN_POINT('Ctrl Pts',(18.1967285688977,-7.6769832497116,9.0625069894267));
#94465=CARTESIAN_POINT('Ctrl Pts',(18.3999671286159,-10.9929383413539,4.52773913144796));
#94466=CARTESIAN_POINT('Ctrl Pts',(18.6142643904826,-11.8612734120244,-1.01283062439117));
#94467=CARTESIAN_POINT('Ctrl Pts',(18.746839574998,-10.0814706687781,-6.34979580437877));
#94468=CARTESIAN_POINT('Ctrl Pts',(18.9157801590528,-6.04754161886867,-10.2790745664293));
#94469=CARTESIAN_POINT('Ctrl Pts',(19.0672944337368,-0.655174918774475,
-11.9180843893191));
#94470=CARTESIAN_POINT('Ctrl Pts',(19.2275478343006,4.89268465504261,-10.8991049408004));
#94471=CARTESIAN_POINT('Ctrl Pts',(19.3838460285229,9.3578015813762,-7.44340319910321));
#94472=CARTESIAN_POINT('Ctrl Pts',(19.5421535987863,11.7403421743398,-2.32008648120949));
#94473=CARTESIAN_POINT('Ctrl Pts',(19.6997636988169,11.5052746138427,3.33148982193097));
#94474=CARTESIAN_POINT('Ctrl Pts',(19.8578668941574,8.69955374686446,8.24565437927413));
#94475=CARTESIAN_POINT('Ctrl Pts',(20.0159574924546,3.94777155655652,11.3328450679878));
#94476=CARTESIAN_POINT('Ctrl Pts',(20.1742022741564,-1.69613308293156,11.8808152256684));
#94477=CARTESIAN_POINT('Ctrl Pts',(20.3326590484748,-6.96488480194656,9.80454780154648));
#94478=CARTESIAN_POINT('Ctrl Pts',(20.5139662157656,-11.237866859747,4.85022961102954));
#94479=CARTESIAN_POINT('Ctrl Pts',(20.6431763802473,-11.8882199022414,0.261240555255304));
#94480=CARTESIAN_POINT('Ctrl Pts',(20.7180435334305,-11.3462020984903,-2.50431251217421));
#94481=CARTESIAN_POINT('Ctrl Pts',(21.8012598463038,-10.0131352633455,0.0110692926695161));
#94482=CARTESIAN_POINT('Ctrl Pts',(21.7552321039728,-10.0072228406033,1.65687208126129));
#94483=CARTESIAN_POINT('Ctrl Pts',(21.7096578718089,-9.62567683521378,3.2083740442833));
#94484=CARTESIAN_POINT('Ctrl Pts',(21.6639548339268,-8.89621852178167,4.61102195828347));
#94485=CARTESIAN_POINT('Ctrl Pts',(21.6639546335718,-8.8962153239491,4.61102810727525));
#94486=CARTESIAN_POINT('Ctrl Pts',(21.6639544332167,-8.89621212610985,4.61103425626419));
#94487=CARTESIAN_POINT('Ctrl Pts',(21.6639542328617,-8.89620892826391,4.61104040525026));
#94488=CARTESIAN_POINT('Ctrl Pts',(21.6182513942267,-8.16675076227458,6.01368086513788));
#94489=CARTESIAN_POINT('Ctrl Pts',(21.5724221870221,-7.08938010597456,7.26746591912194));
#94490=CARTESIAN_POINT('Ctrl Pts',(21.526625916955,-5.78896373027067,8.1934202438268));
#94491=CARTESIAN_POINT('Ctrl Pts',(21.5266257407303,-5.78895872624974,8.19342380691236));
#94492=CARTESIAN_POINT('Ctrl Pts',(21.5266255645056,-5.78895372222556,8.19342736999304));
#94493=CARTESIAN_POINT('Ctrl Pts',(21.5266253882809,-5.78894871819804,8.19343093306889));
#94494=CARTESIAN_POINT('Ctrl Pts',(21.4808290939245,-4.48852992910524,9.11938323095388));
#94495=CARTESIAN_POINT('Ctrl Pts',(21.4350653781105,-2.96506634557888,9.71750451332759));
#94496=CARTESIAN_POINT('Ctrl Pts',(21.3892587628962,-1.38607543009952,9.93797605507653));
#94497=CARTESIAN_POINT('Ctrl Pts',(21.3892586998405,-1.38607325652168,9.93797635856913));
#94498=CARTESIAN_POINT('Ctrl Pts',(21.3892586367849,-1.38607108294374,9.93797666206101));
#94499=CARTESIAN_POINT('Ctrl Pts',(21.3892585737293,-1.38606890936569,9.93797696555218));
#94500=CARTESIAN_POINT('Ctrl Pts',(21.3434518723909,0.192925123692123,10.1584478815394));
#94501=CARTESIAN_POINT('Ctrl Pts',(21.2976024042792,1.82744571608953,10.0012674688134));
#94502=CARTESIAN_POINT('Ctrl Pts',(21.2517547214262,3.33399312150951,9.47471961389721));
#94503=CARTESIAN_POINT('Ctrl Pts',(21.2517546941993,3.3339940161786,9.4747193012047));
#94504=CARTESIAN_POINT('Ctrl Pts',(21.2517546669725,3.33399491084763,9.47471898851206));
#94505=CARTESIAN_POINT('Ctrl Pts',(21.2517546397457,3.33399580551663,9.47471867581929));
#94506=CARTESIAN_POINT('Ctrl Pts',(21.205906928113,4.84054400470364,8.94817005165259));
#94507=CARTESIAN_POINT('Ctrl Pts',(21.1600609297291,6.21911907103573,8.05225365383932));
#94508=CARTESIAN_POINT('Ctrl Pts',(21.114170584641,7.31607797187692,6.89067769931178));
#94509=CARTESIAN_POINT('Ctrl Pts',(21.1141705230266,7.31607944470209,6.89067613972892));
#94510=CARTESIAN_POINT('Ctrl Pts',(21.1141704614123,7.31608091752672,6.89067458014561));
#94511=CARTESIAN_POINT('Ctrl Pts',(21.1141703997979,7.31608239035088,6.89067302056179));
#94512=CARTESIAN_POINT('Ctrl Pts',(21.0682800523852,8.41304058769296,5.72909629683467));
#94513=CARTESIAN_POINT('Ctrl Pts',(21.0223453621309,9.22838215118901,4.3018603581543));
#94514=CARTESIAN_POINT('Ctrl Pts',(20.9764473487262,9.67043942004942,2.76588563764872));
#94515=CARTESIAN_POINT('Ctrl Pts',(20.9764472893075,9.67043999232902,2.76588364920274));
#94516=CARTESIAN_POINT('Ctrl Pts',(20.9764472298887,9.67044056460801,2.7658816607565));
#94517=CARTESIAN_POINT('Ctrl Pts',(20.9764471704699,9.67044113688636,2.76587967231016));
#94518=CARTESIAN_POINT('Ctrl Pts',(20.9305491360636,10.11249764244,1.22990396426352));
#94519=CARTESIAN_POINT('Ctrl Pts',(20.8846874736051,10.1812698512961,-0.414810572222863));
#94520=CARTESIAN_POINT('Ctrl Pts',(20.8386848325414,9.86855581097698,-1.9838833732313));
#94521=CARTESIAN_POINT('Ctrl Pts',(20.838684794132,9.86855554987952,-1.98388468331296));
#94522=CARTESIAN_POINT('Ctrl Pts',(20.8386847557225,9.86855528878179,-1.98388599339458));
#94523=CARTESIAN_POINT('Ctrl Pts',(20.8386847173131,9.86855502768379,-1.98388730347614));
#94524=CARTESIAN_POINT('Ctrl Pts',(20.7926820752953,9.55584034544212,-3.55296000268544));
#94525=CARTESIAN_POINT('Ctrl Pts',(20.7465380004342,8.86163811437252,-5.04638936815762));
#94526=CARTESIAN_POINT('Ctrl Pts',(20.7006508715133,7.86285962965014,-6.29766374980489));
#94527=CARTESIAN_POINT('Ctrl Pts',(20.7006508339172,7.86285881133398,-6.29766477499523));
#94528=CARTESIAN_POINT('Ctrl Pts',(20.7006507963211,7.8628579930176,-6.29766580018542));
#94529=CARTESIAN_POINT('Ctrl Pts',(20.700650758725,7.86285717470103,-6.29766682537543));
#94530=CARTESIAN_POINT('Ctrl Pts',(20.654763592629,6.864077372574,-7.54894183541054));
#94531=CARTESIAN_POINT('Ctrl Pts',(20.6091309971028,5.56071904099251,-8.55806363998203));
#94532=CARTESIAN_POINT('Ctrl Pts',(20.5628824954473,4.09777307274928,-9.21188334086465));
#94533=CARTESIAN_POINT('Ctrl Pts',(20.5166339937918,2.63482710450628,-9.86570304174717));
#94534=CARTESIAN_POINT('Ctrl Pts',(20.4697652785271,1.01230003976588,-10.1642142991518));
#94535=CARTESIAN_POINT('Ctrl Pts',(20.4241375419168,-0.588808414128353,
-10.0733777577267));
#94536=CARTESIAN_POINT('Ctrl Pts',(20.4241375049837,-0.588809710136394,
-10.0733776841996));
#94537=CARTESIAN_POINT('Ctrl Pts',(20.4241374680506,-0.588811006144456,
-10.0733776106722));
#94538=CARTESIAN_POINT('Ctrl Pts',(20.4241374311175,-0.588812302152469,
-10.0733775371446));
#94539=CARTESIAN_POINT('Ctrl Pts',(20.3869849920578,-1.89251680263734,-9.99941325827055));
#94540=CARTESIAN_POINT('Ctrl Pts',(20.3506467756454,-3.18203022746201,-9.66729770391613));
#94541=CARTESIAN_POINT('Ctrl Pts',(20.3130702272109,-4.36215581350889,-9.10582210716729));
#94542=CARTESIAN_POINT('Ctrl Pts',(20.3044982202458,-4.63136746717885,-8.97773762558053));
#94543=CARTESIAN_POINT('Ctrl Pts',(20.2958617694733,-4.89488680516154,-8.83771756778075));
#94544=CARTESIAN_POINT('Ctrl Pts',(20.2871365063085,-5.15158403690282,-8.68610395029341));
#94545=CARTESIAN_POINT('Ctrl Pts',(20.2577530055678,-6.01604659310811,-8.17552464081054));
#94546=CARTESIAN_POINT('Ctrl Pts',(20.2273530245799,-6.80312796209644,-7.53346619228489));
#94547=CARTESIAN_POINT('Ctrl Pts',(20.1978687745464,-7.48035522254219,-6.79116690820229));
#94548=CARTESIAN_POINT('Ctrl Pts',(20.1802182937909,-7.88577122308478,-6.34679612673033));
#94549=CARTESIAN_POINT('Ctrl Pts',(20.1628959739862,-8.25181824281081,-5.86650099312686));
#94550=CARTESIAN_POINT('Ctrl Pts',(20.1463164348685,-8.57152250286074,-5.35697778778339));
#94551=CARTESIAN_POINT('Ctrl Pts',(20.1463158899337,-8.57153301087137,-5.35696104082088));
#94552=CARTESIAN_POINT('Ctrl Pts',(20.1463153449997,-8.57154351883193,-5.35694429382681));
#94553=CARTESIAN_POINT('Ctrl Pts',(20.1463148000665,-8.57155402674243,-5.35692754680115));
#94554=CARTESIAN_POINT('Ctrl Pts',(20.124177885672,-8.9984186839762,-4.67661024045451));
#94555=CARTESIAN_POINT('Ctrl Pts',(20.1033676350582,-9.34266561105165,-3.94417968405986));
#94556=CARTESIAN_POINT('Ctrl Pts',(20.0816978875363,-9.59692940229535,-3.18135205301605));
#94557=CARTESIAN_POINT('Ctrl Pts',(20.0600281400144,-9.85119319353904,-2.41852442197224));
#94558=CARTESIAN_POINT('Ctrl Pts',(20.0374986949878,-10.0154731210975,-1.6253016744882));
#94559=CARTESIAN_POINT('Ctrl Pts',(20.0119245448109,-10.0824548219061,-0.823411832214975));
#94560=CARTESIAN_POINT('Ctrl Pts',(20.0119241634875,-10.0824558206367,-0.823399875636732));
#94561=CARTESIAN_POINT('Ctrl Pts',(20.0119237821635,-10.0824568193457,-0.823387919056553));
#94562=CARTESIAN_POINT('Ctrl Pts',(20.0119234008388,-10.0824578180331,-0.823375962474456));
#94563=CARTESIAN_POINT('Ctrl Pts',(19.9903962735522,-10.1388372485164,-0.148384658059219));
#94564=CARTESIAN_POINT('Ctrl Pts',(19.9666927510919,-10.1262680360043,0.532755007697934));
#94565=CARTESIAN_POINT('Ctrl Pts',(19.941867359469,-10.0468329681363,1.20616332848875));
#94566=CARTESIAN_POINT('Ctrl Pts',(19.9174215132727,-9.96861235106805,1.86927618034265));
#94567=CARTESIAN_POINT('Ctrl Pts',(19.8918877223371,-9.82555490974834,2.52489398467586));
#94568=CARTESIAN_POINT('Ctrl Pts',(19.8662718761862,-9.61960087318472,3.15976851342234));
#94569=CARTESIAN_POINT('Ctrl Pts',(19.8560918131859,-9.53775212007169,3.41207572442991));
#94570=CARTESIAN_POINT('Ctrl Pts',(19.8458987889727,-9.44596912518285,3.66110671853785));
#94571=CARTESIAN_POINT('Ctrl Pts',(19.835755958896,-9.34437144790041,3.90602921000172));
#94572=CARTESIAN_POINT('Ctrl Pts',(19.8357530127888,-9.34434193763071,3.90610035069086));
#94573=CARTESIAN_POINT('Ctrl Pts',(19.8357500666855,-9.34431242653295,3.90617149103258));
#94574=CARTESIAN_POINT('Ctrl Pts',(19.8357471205861,-9.34428291460712,3.90624263102687));
#94575=CARTESIAN_POINT('Ctrl Pts',(19.8117357691311,-9.10375429369162,4.48604907321725));
#94576=CARTESIAN_POINT('Ctrl Pts',(19.7879846941381,-8.80821627629863,5.04277518921063));
#94577=CARTESIAN_POINT('Ctrl Pts',(19.7643605893076,-8.4641163047614,5.56782142106315));
#94578=CARTESIAN_POINT('Ctrl Pts',(19.7410989170983,-8.12529539270751,6.08481258020796));
#94579=CARTESIAN_POINT('Ctrl Pts',(19.7179603319782,-7.73939199826957,6.57108722534719));
#94580=CARTESIAN_POINT('Ctrl Pts',(19.6948177172066,-7.31260286916265,7.01846154723225));
#94581=CARTESIAN_POINT('Ctrl Pts',(19.6811884207982,-7.06125549109592,7.28193208842314));
#94582=CARTESIAN_POINT('Ctrl Pts',(19.6675577307813,-6.7957282621181,7.5319112443041));
#94583=CARTESIAN_POINT('Ctrl Pts',(19.6538997436435,-6.51729200697241,7.76673429501901));
#94584=CARTESIAN_POINT('Ctrl Pts',(19.6538977922536,-6.51725222529157,7.76676784544746));
#94585=CARTESIAN_POINT('Ctrl Pts',(19.6538958408632,-6.51721244334721,7.76680139556654));
#94586=CARTESIAN_POINT('Ctrl Pts',(19.6538938894722,-6.51717266113936,7.76683494537624));
#94587=CARTESIAN_POINT('Ctrl Pts',(19.634469850311,-6.1211827374716,8.10078791825245));
#94588=CARTESIAN_POINT('Ctrl Pts',(19.6148942435515,-5.69895233032108,8.40408527570492));
#94589=CARTESIAN_POINT('Ctrl Pts',(19.595280716088,-5.25602148926852,8.67378800972723));
#94590=CARTESIAN_POINT('Ctrl Pts',(19.5757664198158,-4.81533157887535,8.94212623021926));
#94591=CARTESIAN_POINT('Ctrl Pts',(19.5562145820723,-4.35415070186316,9.17721014280609));
#94592=CARTESIAN_POINT('Ctrl Pts',(19.5367352573205,-3.87788785491096,9.37616483050553));
#94593=CARTESIAN_POINT('Ctrl Pts',(19.5175565925449,-3.40897604184072,9.57204868734002));
#94594=CARTESIAN_POINT('Ctrl Pts',(19.4984482568019,-2.92544428516652,9.73291139569341));
#94595=CARTESIAN_POINT('Ctrl Pts',(19.479513211645,-2.43240488101956,9.8560087263723));
#94596=CARTESIAN_POINT('Ctrl Pts',(19.4768973989063,-2.36429314728155,9.87301420816653));
#94597=CARTESIAN_POINT('Ctrl Pts',(19.4742848894049,-2.29599988597296,9.88929893672284));
#94598=CARTESIAN_POINT('Ctrl Pts',(19.47167595057,-2.22753849970242,9.90485565245439));
#94599=CARTESIAN_POINT('Ctrl Pts',(19.4716749594633,-2.22751249198904,9.90486156227635));
#94600=CARTESIAN_POINT('Ctrl Pts',(19.4716739683572,-2.22748648425137,9.90486747199325));
#94601=CARTESIAN_POINT('Ctrl Pts',(19.4716729772516,-2.22746047648946,9.90487338160508));
#94602=CARTESIAN_POINT('Ctrl Pts',(19.4526695341822,-1.72878805869038,10.0181841859249));
#94603=CARTESIAN_POINT('Ctrl Pts',(19.4335943739675,-1.22127886684315,10.0925805320568));
#94604=CARTESIAN_POINT('Ctrl Pts',(19.4144573514764,-0.710925040065703,
10.1285809678906));
#94605=CARTESIAN_POINT('Ctrl Pts',(19.4034059597798,-0.416202073304849,
10.1493707703706));
#94606=CARTESIAN_POINT('Ctrl Pts',(19.3923339298187,-0.120530316333381,
10.1573568038));
#94607=CARTESIAN_POINT('Ctrl Pts',(19.3812431031346,0.174938904745155,10.1526464163313));
#94608=CARTESIAN_POINT('Ctrl Pts',(19.367234298816,0.54814557527839,10.1466967339322));
#94609=CARTESIAN_POINT('Ctrl Pts',(19.3532302365177,0.921032258087055,10.1205304950431));
#94610=CARTESIAN_POINT('Ctrl Pts',(19.339224780055,1.29144034910869,10.0743364254749));
#94611=CARTESIAN_POINT('Ctrl Pts',(19.3253210843792,1.6591571305744,10.0284779925837));
#94612=CARTESIAN_POINT('Ctrl Pts',(19.3114160154,2.02443215356254,9.96288156953981));
#94613=CARTESIAN_POINT('Ctrl Pts',(19.297503567475,2.38514521264296,9.8776815478027));
#94614=CARTESIAN_POINT('Ctrl Pts',(19.2951223254824,2.44688453329987,9.86309878920945));
#94615=CARTESIAN_POINT('Ctrl Pts',(19.292740867301,2.50849016982679,9.84794161757506));
#94616=CARTESIAN_POINT('Ctrl Pts',(19.2903591627888,2.56995143539188,9.83221056223149));
#94617=CARTESIAN_POINT('Ctrl Pts',(19.2813733359762,2.80183590519031,9.7728595645881));
#94618=CARTESIAN_POINT('Ctrl Pts',(19.2721417232226,3.03161724004271,9.70509961279013));
#94619=CARTESIAN_POINT('Ctrl Pts',(19.2628557069655,3.25871007913323,9.62915773747277));
#94620=CARTESIAN_POINT('Ctrl Pts',(19.2564784511862,3.41466814343352,9.57700396670104));
#94621=CARTESIAN_POINT('Ctrl Pts',(19.2500754855842,3.56935930716621,9.52099122486019));
#94622=CARTESIAN_POINT('Ctrl Pts',(19.2437084341844,3.7226077917393,9.46118958148128));
#94623=CARTESIAN_POINT('Ctrl Pts',(19.2384963879363,3.84805647102597,9.41223616310356));
#94624=CARTESIAN_POINT('Ctrl Pts',(19.2333426313397,3.9725439656621,9.36077843730233));
#94625=CARTESIAN_POINT('Ctrl Pts',(19.2282358010473,4.09595243702679,9.30681574951009));
#94626=CARTESIAN_POINT('Ctrl Pts',(19.2172042602722,4.36253376162538,9.19024802420344));
#94627=CARTESIAN_POINT('Ctrl Pts',(19.206391616527,4.62408128943517,9.06198823680086));
#94628=CARTESIAN_POINT('Ctrl Pts',(19.1956845759001,4.87965142449191,8.92270348980286));
#94629=CARTESIAN_POINT('Ctrl Pts',(19.1890405303381,5.03824049506218,8.83627305235708));
#94630=CARTESIAN_POINT('Ctrl Pts',(19.1824371599625,5.19452748575743,8.7455983281303));
#94631=CARTESIAN_POINT('Ctrl Pts',(19.1758476884273,5.34828392190368,8.65084831487406));
#94632=CARTESIAN_POINT('Ctrl Pts',(19.1642510595093,5.61887562629458,8.48410038405133));
#94633=CARTESIAN_POINT('Ctrl Pts',(19.1524794813995,5.88150243049401,8.30454934728981));
#94634=CARTESIAN_POINT('Ctrl Pts',(19.1406254170227,6.13522621453266,8.11322353794057));
#94635=CARTESIAN_POINT('Ctrl Pts',(19.1298638760916,6.36556568294915,7.93953116855219));
#94636=CARTESIAN_POINT('Ctrl Pts',(19.1190342942608,6.58856830199439,7.75613396617955));
#94637=CARTESIAN_POINT('Ctrl Pts',(19.108204579914,6.80354429825768,7.56376615684175));
#94638=CARTESIAN_POINT('Ctrl Pts',(19.0919038331487,7.12712340325566,7.2742166040642));
#94639=CARTESIAN_POINT('Ctrl Pts',(19.0754871645745,7.43259455463111,6.96412257454898));
#94640=CARTESIAN_POINT('Ctrl Pts',(19.0589508125994,7.71724725468761,6.63579139086323));
#94641=CARTESIAN_POINT('Ctrl Pts',(19.0447034020989,7.96249867857266,6.35290740525968));
#94642=CARTESIAN_POINT('Ctrl Pts',(19.0303671439565,8.19229576213723,6.05648491838939));
#94643=CARTESIAN_POINT('Ctrl Pts',(19.0159394491088,8.40487491321349,5.74799131248794));
#94644=CARTESIAN_POINT('Ctrl Pts',(19.0055524005619,8.55791876294694,5.52589498353811));
#94645=CARTESIAN_POINT('Ctrl Pts',(18.9953172726759,8.70218781720836,5.29768840615742));
#94646=CARTESIAN_POINT('Ctrl Pts',(18.9852673388218,8.83701581138607,5.06402271675237));
#94647=CARTESIAN_POINT('Ctrl Pts',(18.9802364943451,8.90450866055792,4.94705321625779));
#94648=CARTESIAN_POINT('Ctrl Pts',(18.9752520388962,8.96963621777626,4.82871589318936));
#94649=CARTESIAN_POINT('Ctrl Pts',(18.9703179714697,9.03237656637081,4.70912775998958));
#94650=CARTESIAN_POINT('Ctrl Pts',(18.9617751113042,9.14100540713056,4.50207248265815));
#94651=CARTESIAN_POINT('Ctrl Pts',(18.9533225967343,9.242415344085,4.29124763660322));
#94652=CARTESIAN_POINT('Ctrl Pts',(18.944777313324,9.33632158440304,4.07713252975304));
#94653=CARTESIAN_POINT('Ctrl Pts',(18.9385277279412,9.40499982930891,3.92053963777375));
#94654=CARTESIAN_POINT('Ctrl Pts',(18.9322286104738,9.46966391058422,3.76218776214099));
#94655=CARTESIAN_POINT('Ctrl Pts',(18.9258092124385,9.53019546327616,3.602280621641));
#94656=CARTESIAN_POINT('Ctrl Pts',(18.9121976210768,9.65854562246522,3.26321601771301));
#94657=CARTESIAN_POINT('Ctrl Pts',(18.8985893188567,9.76890358393514,2.91729476422134));
#94658=CARTESIAN_POINT('Ctrl Pts',(18.8849695342091,9.86087135309376,2.56646304735015));
#94659=CARTESIAN_POINT('Ctrl Pts',(18.8713326158262,9.95295481801741,2.21518998299113));
#94660=CARTESIAN_POINT('Ctrl Pts',(18.8576841867703,10.0266019242977,1.85899313727757));
#94661=CARTESIAN_POINT('Ctrl Pts',(18.8440095841095,10.0813622058563,1.49981740195999));
#94662=CARTESIAN_POINT('Ctrl Pts',(18.8408455278202,10.0940327468269,1.41671061834878));
#94663=CARTESIAN_POINT('Ctrl Pts',(18.8376800709236,10.1056919125858,1.33344435017619));
#94664=CARTESIAN_POINT('Ctrl Pts',(18.8345130329549,10.1163337231934,1.25004270792199));
#94665=CARTESIAN_POINT('Ctrl Pts',(18.8214905737337,10.1600915012969,0.907105712539461));
#94666=CARTESIAN_POINT('Ctrl Pts',(18.8083373000925,10.1865317447387,0.561871096406014));
#94667=CARTESIAN_POINT('Ctrl Pts',(18.7951789993763,10.1953684639573,0.216188414535579));
#94668=CARTESIAN_POINT('Ctrl Pts',(18.7820567714032,10.2041809578062,-0.128546597662148));
#94669=CARTESIAN_POINT('Ctrl Pts',(18.7689295439125,10.1954871963454,-0.473726922080629));
#94670=CARTESIAN_POINT('Ctrl Pts',(18.7559203408355,10.1690199689852,-0.817567059789181));
#94671=CARTESIAN_POINT('Ctrl Pts',(18.7513969361009,10.1598171007662,-0.937123046242575));
#94672=CARTESIAN_POINT('Ctrl Pts',(18.7468877842316,10.148465489433,-1.05651745587199));
#94673=CARTESIAN_POINT('Ctrl Pts',(18.7423979944009,10.1349540741866,-1.17567670015723));
#94674=CARTESIAN_POINT('Ctrl Pts',(18.7423966095271,10.1349499065963,-1.17571345477601));
#94675=CARTESIAN_POINT('Ctrl Pts',(18.7423952246546,10.1349457387999,-1.17575020937153));
#94676=CARTESIAN_POINT('Ctrl Pts',(18.7423938397834,10.1349415707974,-1.17578696394395));
#94677=CARTESIAN_POINT('Ctrl Pts',(18.7293207128352,10.0955957997368,-1.5227486117345));
#94678=CARTESIAN_POINT('Ctrl Pts',(18.7163628972734,10.0378869685745,-1.86764796597857));
#94679=CARTESIAN_POINT('Ctrl Pts',(18.703411088082,9.96250064782994,-2.20873737228892));
#94680=CARTESIAN_POINT('Ctrl Pts',(18.6904833212053,9.88725426596347,-2.54919361772379));
#94681=CARTESIAN_POINT('Ctrl Pts',(18.6775615325368,9.79439528578715,-2.88585351530137));
#94682=CARTESIAN_POINT('Ctrl Pts',(18.6645392706148,9.68463728913615,-3.21693841612392));
#94683=CARTESIAN_POINT('Ctrl Pts',(18.6603209734357,9.649083416051,-3.32418664316367));
#94684=CARTESIAN_POINT('Ctrl Pts',(18.6560921506786,9.61175661398904,-3.43084959950089));
#94685=CARTESIAN_POINT('Ctrl Pts',(18.6518492277839,9.57268203809672,-3.53686607171212));
#94686=CARTESIAN_POINT('Ctrl Pts',(18.6381474504394,9.44649752991839,-3.87922772501948));
#94687=CARTESIAN_POINT('Ctrl Pts',(18.6244496581371,9.30225079458742,-4.21491485204093));
#94688=CARTESIAN_POINT('Ctrl Pts',(18.6107369118527,9.14080367032811,-4.54213068876285));
#94689=CARTESIAN_POINT('Ctrl Pts',(18.5970130610206,8.97922580659091,-4.86961150405186));
#94690=CARTESIAN_POINT('Ctrl Pts',(18.583274233299,8.80041916864338,-5.188608118226));
#94691=CARTESIAN_POINT('Ctrl Pts',(18.569501693905,8.60520333982285,-5.4972929078017));
#94692=CARTESIAN_POINT('Ctrl Pts',(18.5664378308966,8.56177528785086,-5.56596346164793));
#94693=CARTESIAN_POINT('Ctrl Pts',(18.5633723004489,8.5175350014068,-5.63412356014589));
#94694=CARTESIAN_POINT('Ctrl Pts',(18.560304897842,8.47249124519888,-5.70175284157591));
#94695=CARTESIAN_POINT('Ctrl Pts',(18.5451573471326,8.25005465348676,-6.03572203348332));
#94696=CARTESIAN_POINT('Ctrl Pts',(18.5300479666999,8.00805772463506,-6.35687179147185));
#94697=CARTESIAN_POINT('Ctrl Pts',(18.5149615377423,7.74768798431707,-6.66252915693987));
#94698=CARTESIAN_POINT('Ctrl Pts',(18.5097041125412,7.65695250024724,-6.76904679213579));
#94699=CARTESIAN_POINT('Ctrl Pts',(18.5044494775643,7.56398621837468,-6.87368306948572));
#94700=CARTESIAN_POINT('Ctrl Pts',(18.4991969987272,7.46884082764176,-6.97632527323337));
#94701=CARTESIAN_POINT('Ctrl Pts',(18.4842276610716,7.1976805765599,-7.2688511173695));
#94702=CARTESIAN_POINT('Ctrl Pts',(18.4692758071308,6.90881780322808,-7.54517844328599));
#94703=CARTESIAN_POINT('Ctrl Pts',(18.4543266982082,6.60466043780798,-7.80369363392125));
#94704=CARTESIAN_POINT('Ctrl Pts',(18.439392442126,6.30080527105759,-8.06195197413765));
#94705=CARTESIAN_POINT('Ctrl Pts',(18.4244609248482,5.98168662098567,-8.30243285908742));
#94706=CARTESIAN_POINT('Ctrl Pts',(18.4095178565894,5.64974343316438,-8.52356187903403));
#94707=CARTESIAN_POINT('Ctrl Pts',(18.3988128677656,5.41194433767359,-8.68197537525669));
#94708=CARTESIAN_POINT('Ctrl Pts',(18.3881019597623,5.1675644243093,-8.8304580363769));
#94709=CARTESIAN_POINT('Ctrl Pts',(18.3773800048889,4.91750920954781,-8.96844496388976));
#94710=CARTESIAN_POINT('Ctrl Pts',(18.3638173439019,4.60120363412619,-9.14299055194817));
#94711=CARTESIAN_POINT('Ctrl Pts',(18.3502497557113,4.27559261611256,-9.30089922915152));
#94712=CARTESIAN_POINT('Ctrl Pts',(18.3366746234865,3.94241652222267,-9.44101520914165));
#94713=CARTESIAN_POINT('Ctrl Pts',(18.3153574710193,3.41922709951646,-9.66104059519825));
#94714=CARTESIAN_POINT('Ctrl Pts',(18.2940216981756,2.87738122411373,-9.83718946395088));
#94715=CARTESIAN_POINT('Ctrl Pts',(18.2726580888735,2.32458303169984,-9.96772456439307));
#94716=CARTESIAN_POINT('Ctrl Pts',(18.250729396379,1.75716292016651,-10.1017124143325));
#94717=CARTESIAN_POINT('Ctrl Pts',(18.2287713755917,1.17820441143369,-10.1876408285472));
#94718=CARTESIAN_POINT('Ctrl Pts',(18.2067744407027,0.59607679853009,-10.2236697840988));
#94719=CARTESIAN_POINT('Ctrl Pts',(18.2024571223697,0.481823143279075,-10.2307411543196));
#94720=CARTESIAN_POINT('Ctrl Pts',(18.1981383061371,0.367447494538484,-10.2358904563959));
#94721=CARTESIAN_POINT('Ctrl Pts',(18.1938179211529,0.253013238920589,-10.2391039859528));
#94722=CARTESIAN_POINT('Ctrl Pts',(18.1869926579869,0.072232148197292,-10.2441806596746));
#94723=CARTESIAN_POINT('Ctrl Pts',(18.1801772901769,-0.108689414234473,
-10.2444430843383));
#94724=CARTESIAN_POINT('Ctrl Pts',(18.1733699101441,-0.28950481593069,-10.2398365230604));
#94725=CARTESIAN_POINT('Ctrl Pts',(18.1505110747668,-0.896673723967822,
-10.2243679249506));
#94726=CARTESIAN_POINT('Ctrl Pts',(18.1277421344973,-1.5026493854274,-10.1539963544201));
#94727=CARTESIAN_POINT('Ctrl Pts',(18.1049918601463,-2.09793712912939,-10.0310006372786));
#94728=CARTESIAN_POINT('Ctrl Pts',(18.0826179976676,-2.68337561252395,-9.91003993068066));
#94729=CARTESIAN_POINT('Ctrl Pts',(18.0602621798692,-3.25847588047912,-9.73818053721335));
#94730=CARTESIAN_POINT('Ctrl Pts',(18.0378589922131,-3.81416626982286,-9.51761782230471));
#94731=CARTESIAN_POINT('Ctrl Pts',(18.0287633782693,-4.03977457750649,-9.42807015007052));
#94732=CARTESIAN_POINT('Ctrl Pts',(18.0196599837846,-4.26218311516417,-9.33049500578815));
#94733=CARTESIAN_POINT('Ctrl Pts',(18.0105445400155,-4.48078356598075,-9.22504148541237));
#94734=CARTESIAN_POINT('Ctrl Pts',(18.0105443969714,-4.48078699636842,-9.22503983058296));
#94735=CARTESIAN_POINT('Ctrl Pts',(18.0105442539273,-4.48079042675514,-9.22503817575162));
#94736=CARTESIAN_POINT('Ctrl Pts',(18.0105441108832,-4.48079385714093,-9.22503652091832));
#94737=CARTESIAN_POINT('Ctrl Pts',(17.9947726209851,-4.85901491375055,-9.04258100869975));
#94738=CARTESIAN_POINT('Ctrl Pts',(17.9788511214764,-5.22592814798086,-8.83634109782422));
#94739=CARTESIAN_POINT('Ctrl Pts',(17.9628770807745,-5.57902035708451,-8.60833729963736));
#94740=CARTESIAN_POINT('Ctrl Pts',(17.9468726103616,-5.93278518835648,-8.3798991661546));
#94741=CARTESIAN_POINT('Ctrl Pts',(17.9308153584739,-6.27267695388216,-8.12961526102735));
#94742=CARTESIAN_POINT('Ctrl Pts',(17.914801353746,-6.5962127162598,-7.85949148218387));
#94743=CARTESIAN_POINT('Ctrl Pts',(17.9131347589807,-6.62988343243225,-7.83137940881668));
#94744=CARTESIAN_POINT('Ctrl Pts',(17.9114686310051,-6.66337703423234,-7.8030524221574));
#94745=CARTESIAN_POINT('Ctrl Pts',(17.9098030769116,-6.69669074562728,-7.77451275984648));
#94746=CARTESIAN_POINT('Ctrl Pts',(17.8965015877788,-6.96274152825989,-7.54658860561832));
#94747=CARTESIAN_POINT('Ctrl Pts',(17.8833189848059,-7.21737240451834,-7.30519034945689));
#94748=CARTESIAN_POINT('Ctrl Pts',(17.8702570945366,-7.45904810393093,-7.05150363832918));
#94749=CARTESIAN_POINT('Ctrl Pts',(17.862275778808,-7.60672122176878,-6.89649133184858));
#94750=CARTESIAN_POINT('Ctrl Pts',(17.8543395215989,-7.74955791441653,-6.73689169375406));
#94751=CARTESIAN_POINT('Ctrl Pts',(17.8464486327562,-7.88721516077749,-6.57298155457178));
#94752=CARTESIAN_POINT('Ctrl Pts',(17.8434686957871,-7.9392004219654,-6.5110820787215));
#94753=CARTESIAN_POINT('Ctrl Pts',(17.8404952281761,-7.99044708500258,-6.44856790943521));
#94754=CARTESIAN_POINT('Ctrl Pts',(17.8375282434978,-8.04094407617035,-6.38546053050246));
#94755=CARTESIAN_POINT('Ctrl Pts',(17.8256875700402,-8.24246799619445,-6.13361094321279));
#94756=CARTESIAN_POINT('Ctrl Pts',(17.8137158795033,-8.43175580671531,-5.87217915639835));
#94757=CARTESIAN_POINT('Ctrl Pts',(17.801679482491,-8.6082791557546,-5.60247192802518));
#94758=CARTESIAN_POINT('Ctrl Pts',(17.7896430854786,-8.78480250479389,-5.33276469965201));
#94759=CARTESIAN_POINT('Ctrl Pts',(17.7775419369184,-8.94856212650403,-5.05478186072294));
#94760=CARTESIAN_POINT('Ctrl Pts',(17.7654406557367,-9.09902413406252,-4.76977631388784));
#94761=CARTESIAN_POINT('Ctrl Pts',(17.7411908055945,-9.40053610462235,-4.1986515134074));
#94762=CARTESIAN_POINT('Ctrl Pts',(17.7166586862939,-9.64865843917535,-3.59854123922697));
#94763=CARTESIAN_POINT('Ctrl Pts',(17.6919981760056,-9.83778134329656,-2.97969614991501));
#94764=CARTESIAN_POINT('Ctrl Pts',(17.6889624280202,-9.8610626731826,-2.90351533649331));
#94765=CARTESIAN_POINT('Ctrl Pts',(17.6859247268684,-9.88344988947285,-2.82705055961025));
#94766=CARTESIAN_POINT('Ctrl Pts',(17.6828853537619,-9.90493248426554,-2.75032089323));
#94767=CARTESIAN_POINT('Ctrl Pts',(17.6769842082569,-9.94664237418528,-2.60134513079617));
#94768=CARTESIAN_POINT('Ctrl Pts',(17.6710767608705,-9.98494213149595,-2.4513708248295));
#94769=CARTESIAN_POINT('Ctrl Pts',(17.6651650595282,-10.0198195814703,-2.30055459795124));
#94770=CARTESIAN_POINT('Ctrl Pts',(17.6522973219507,-10.0957357767686,-1.97227961964137));
#94771=CARTESIAN_POINT('Ctrl Pts',(17.6396119481788,-10.1556767585313,-1.6401897808721));
#94772=CARTESIAN_POINT('Ctrl Pts',(17.6270298268239,-10.1994143540277,-1.30593710606664));
#94773=CARTESIAN_POINT('Ctrl Pts',(17.6153714576621,-10.239940829664,-0.996224541209333));
#94774=CARTESIAN_POINT('Ctrl Pts',(17.6038016807299,-10.2665555446432,-0.684655874297618));
#94775=CARTESIAN_POINT('Ctrl Pts',(17.592258525595,-10.2790961038348,-0.372580399566067));
#94776=CARTESIAN_POINT('Ctrl Pts',(17.5770275132283,-10.2956431752291,0.0391983004023063));
#94777=CARTESIAN_POINT('Ctrl Pts',(17.5617901530121,-10.2876170727355,0.45185830932181));
#94778=CARTESIAN_POINT('Ctrl Pts',(17.5464539621659,-10.2547463325197,0.862452069769172));
#94779=CARTESIAN_POINT('Ctrl Pts',(17.5376242304394,-10.2358211756363,1.09884928141659));
#94780=CARTESIAN_POINT('Ctrl Pts',(17.5287617958741,-10.2086600559606,1.33456068044002));
#94781=CARTESIAN_POINT('Ctrl Pts',(17.5198493665046,-10.1732095241468,1.56901604699944));
#94782=CARTESIAN_POINT('Ctrl Pts',(17.5198486089956,-10.1732065110404,1.56903597445689));
#94783=CARTESIAN_POINT('Ctrl Pts',(17.5198478514862,-10.1732034978741,1.56905590190525));
#94784=CARTESIAN_POINT('Ctrl Pts',(17.5198470939764,-10.173200484648,1.56907582934455));
#94785=CARTESIAN_POINT('Ctrl Pts',(17.5073558585623,-10.1235127845277,1.89767666268265));
#94786=CARTESIAN_POINT('Ctrl Pts',(17.4947058589523,-10.0574516897075,2.22385097079879));
#94787=CARTESIAN_POINT('Ctrl Pts',(17.4819881459334,-9.97568559399591,2.54614782892651));
#94788=CARTESIAN_POINT('Ctrl Pts',(17.4692759110215,-9.89395471872187,2.86830585889723));
#94789=CARTESIAN_POINT('Ctrl Pts',(17.4564959558442,-9.79653311063687,3.18659026499953));
#94790=CARTESIAN_POINT('Ctrl Pts',(17.4437376902098,-9.68405996070656,3.49959551421119));
#94791=CARTESIAN_POINT('Ctrl Pts',(17.435309506378,-9.60975954943429,3.70636858637299));
#94792=CARTESIAN_POINT('Ctrl Pts',(17.4268907678939,-9.52889003367656,3.91083872808492));
#94793=CARTESIAN_POINT('Ctrl Pts',(17.4185069695538,-9.44162666556968,4.11260939061742));
#94794=CARTESIAN_POINT('Ctrl Pts',(17.4056815386412,-9.30813224532637,4.42127565231723));
#94795=CARTESIAN_POINT('Ctrl Pts',(17.3929528110469,-9.1596979908372,4.72361317346604));
#94796=CARTESIAN_POINT('Ctrl Pts',(17.3803993074446,-8.99699031080038,5.01807797662169));
#94797=CARTESIAN_POINT('Ctrl Pts',(17.3716642666606,-8.88377425048699,5.22297392810165));
#94798=CARTESIAN_POINT('Ctrl Pts',(17.3630140391623,-8.76364774845,5.42405912621152));
#94799=CARTESIAN_POINT('Ctrl Pts',(17.3544741344264,-8.63683711837772,5.62082821221169));
#94800=CARTESIAN_POINT('Ctrl Pts',(17.3515975246203,-8.59412180558889,5.68710856308511));
#94801=CARTESIAN_POINT('Ctrl Pts',(17.3487334237889,-8.55064809122632,5.75289929874202));
#94802=CARTESIAN_POINT('Ctrl Pts',(17.3458827774153,-8.50643221126271,5.81818680387046));
#94803=CARTESIAN_POINT('Ctrl Pts',(17.333387457021,-8.31261947048099,6.10436340644308));
#94804=CARTESIAN_POINT('Ctrl Pts',(17.3206960069218,-8.1040504070193,6.38039507946295));
#94805=CARTESIAN_POINT('Ctrl Pts',(17.3078818058807,-7.88208910730421,6.64515211263132));
#94806=CARTESIAN_POINT('Ctrl Pts',(17.2966211407256,-7.68703739354777,6.87781119831359));
#94807=CARTESIAN_POINT('Ctrl Pts',(17.2852655739288,-7.48164344051485,7.10176455976691));
#94808=CARTESIAN_POINT('Ctrl Pts',(17.2738630253563,-7.26680488894806,7.31626338617272));
#94809=CARTESIAN_POINT('Ctrl Pts',(17.2601931479087,-7.0092469708878,7.573414026747));
#94810=CARTESIAN_POINT('Ctrl Pts',(17.246519862059,-6.73811367023367,7.81712741973527));
#94811=CARTESIAN_POINT('Ctrl Pts',(17.232838571973,-6.45474920951727,8.04604258360217));
#94812=CARTESIAN_POINT('Ctrl Pts',(17.2311296270908,-6.4193538453433,8.07463662665728));
#94813=CARTESIAN_POINT('Ctrl Pts',(17.2294205573127,-6.38376760392316,8.10299972063845));
#94814=CARTESIAN_POINT('Ctrl Pts',(17.2277113536755,-6.34799307482937,8.1311291639497));
#94815=CARTESIAN_POINT('Ctrl Pts',(17.2157248791348,-6.09710987235723,8.32839814275821));
#94816=CARTESIAN_POINT('Ctrl Pts',(17.2037337009365,-5.83700500887216,8.51414434313586));
#94817=CARTESIAN_POINT('Ctrl Pts',(17.1917362801185,-5.56867428550647,8.68737258916926));
#94818=CARTESIAN_POINT('Ctrl Pts',(17.1746250574966,-5.18596980147988,8.93443794823621));
#94819=CARTESIAN_POINT('Ctrl Pts',(17.157501125857,-4.78653121196277,9.1560375088926));
#94820=CARTESIAN_POINT('Ctrl Pts',(17.1403602309021,-4.37418424228961,9.35048218560049));
#94821=CARTESIAN_POINT('Ctrl Pts',(17.1232193359472,-3.96183727261646,9.54492686230837));
#94822=CARTESIAN_POINT('Ctrl Pts',(17.1060614790304,-3.53658299214965,9.71221603175966));
#94823=CARTESIAN_POINT('Ctrl Pts',(17.088882648315,-3.1022762544726,9.85070806374306));
#94824=CARTESIAN_POINT('Ctrl Pts',(17.0798919309307,-2.87497736543456,9.92318929021174));
#94825=CARTESIAN_POINT('Ctrl Pts',(17.0707785452362,-2.6451035355068,9.98762468745663));
#94826=CARTESIAN_POINT('Ctrl Pts',(17.0616638621188,-2.41324806760956,10.0439612834198));
#94827=CARTESIAN_POINT('Ctrl Pts',(17.0550977813797,-2.24622287294053,10.0845453205058));
#94828=CARTESIAN_POINT('Ctrl Pts',(17.0485309919751,-2.07816827881241,10.1209268635885));
#94829=CARTESIAN_POINT('Ctrl Pts',(17.0420084069395,-1.90928964157372,10.1530893845166));
#94830=CARTESIAN_POINT('Ctrl Pts',(17.0368192409607,-1.77493504533108,10.178676886785));
#94831=CARTESIAN_POINT('Ctrl Pts',(17.0316753337053,-1.64006844984146,10.2016195926033));
#94832=CARTESIAN_POINT('Ctrl Pts',(17.0265606532138,-1.50478892215686,10.2218482631423));
#94833=CARTESIAN_POINT('Ctrl Pts',(17.0169201874437,-1.24980571094689,10.2599765110806));
#94834=CARTESIAN_POINT('Ctrl Pts',(17.0073834009016,-0.993352406314393,
10.2884619906838));
#94835=CARTESIAN_POINT('Ctrl Pts',(16.9978442181521,-0.736177067748153,
10.3072445951958));
#94836=CARTESIAN_POINT('Ctrl Pts',(16.9896563520273,-0.515433079705401,
10.3233664638358));
#94837=CARTESIAN_POINT('Ctrl Pts',(16.9814667573228,-0.294158037725752,
10.332339608172));
#94838=CARTESIAN_POINT('Ctrl Pts',(16.973209772397,-0.0728546445390353,
10.3341336755772));
#94839=CARTESIAN_POINT('Ctrl Pts',(16.9607343221617,0.261511894023068,10.336844325873));
#94840=CARTESIAN_POINT('Ctrl Pts',(16.9482197472632,0.595934418746781,10.3233565855621));
#94841=CARTESIAN_POINT('Ctrl Pts',(16.9356858030079,0.92896255063804,10.2939768071048));
#94842=CARTESIAN_POINT('Ctrl Pts',(16.9251316367267,1.20938778699667,10.2692376618822));
#94843=CARTESIAN_POINT('Ctrl Pts',(16.9145637222918,1.48882505774369,10.2332295968734));
#94844=CARTESIAN_POINT('Ctrl Pts',(16.9039935118895,1.76641698560807,10.1861081975525));
#94845=CARTESIAN_POINT('Ctrl Pts',(16.8906069793433,2.11797038289025,10.1264317936188));
#94846=CARTESIAN_POINT('Ctrl Pts',(16.8771989382669,2.46670015958735,10.0488841547053));
#94847=CARTESIAN_POINT('Ctrl Pts',(16.8637111621511,2.8106670883483,9.95360013039481));
#94848=CARTESIAN_POINT('Ctrl Pts',(16.8502653922987,3.15356276820557,9.85861285817887));
#94849=CARTESIAN_POINT('Ctrl Pts',(16.836740438657,3.49172508490791,9.74599881830258));
#94850=CARTESIAN_POINT('Ctrl Pts',(16.8230795479737,3.82318234957965,9.61590290219076));
#94851=CARTESIAN_POINT('Ctrl Pts',(16.8188828865038,3.92500689117315,9.5759370953336));
#94852=CARTESIAN_POINT('Ctrl Pts',(16.814673399183,4.02619830248631,9.53432158410991));
#94853=CARTESIAN_POINT('Ctrl Pts',(16.8104494423104,4.12669850269955,9.49106093869667));
#94854=CARTESIAN_POINT('Ctrl Pts',(16.7998612020997,4.37862348516496,9.38261899217268));
#94855=CARTESIAN_POINT('Ctrl Pts',(16.7894225580707,4.62632461651229,9.26421710021958));
#94856=CARTESIAN_POINT('Ctrl Pts',(16.779164157344,4.86888897051797,9.13605335050842));
#94857=CARTESIAN_POINT('Ctrl Pts',(16.7740341448704,4.99019035022373,9.07196132951896));
#94858=CARTESIAN_POINT('Ctrl Pts',(16.7689491755291,5.11020755854454,9.00542848872651));
#94859=CARTESIAN_POINT('Ctrl Pts',(16.763912847087,5.22886012688302,8.93654589424496));
#94860=CARTESIAN_POINT('Ctrl Pts',(16.7561547036587,5.41163685677494,8.83043664147353));
#94861=CARTESIAN_POINT('Ctrl Pts',(16.7484773850953,5.59114098951574,8.71870478050094));
#94862=CARTESIAN_POINT('Ctrl Pts',(16.7407503797405,5.7669795739698,8.60146812722601));
#94863=CARTESIAN_POINT('Ctrl Pts',(16.7334306293306,5.93355051465727,8.49041047921498));
#94864=CARTESIAN_POINT('Ctrl Pts',(16.7260663875089,6.096831513901,8.37441282019649));
#94865=CARTESIAN_POINT('Ctrl Pts',(16.7185490576543,6.25645321374314,8.25360003215423));
#94866=CARTESIAN_POINT('Ctrl Pts',(16.7050907291846,6.54222506477346,8.03730804866381));
#94867=CARTESIAN_POINT('Ctrl Pts',(16.6916366227093,6.81683913927164,7.80621957500194));
#94868=CARTESIAN_POINT('Ctrl Pts',(16.678178118772,7.07903371690306,7.56169564596312));
#94869=CARTESIAN_POINT('Ctrl Pts',(16.6646383037058,7.34281237380756,7.3156943969459));
#94870=CARTESIAN_POINT('Ctrl Pts',(16.6510940379693,7.5940216671676,7.05609418330936));
#94871=CARTESIAN_POINT('Ctrl Pts',(16.6375366443296,7.83134159126811,6.78424238248881));
#94872=CARTESIAN_POINT('Ctrl Pts',(16.6336236717245,7.89983752686763,6.70577976072541));
#94873=CARTESIAN_POINT('Ctrl Pts',(16.6297096061469,7.9671761768322,6.62629633588331));
#94874=CARTESIAN_POINT('Ctrl Pts',(16.6257942404647,8.03332514219299,6.54582403594911));
#94875=CARTESIAN_POINT('Ctrl Pts',(16.6137509363714,8.23679326495746,6.29829865572819));
#94876=CARTESIAN_POINT('Ctrl Pts',(16.6016014173788,8.42887435709483,6.04131725621301));
#94877=CARTESIAN_POINT('Ctrl Pts',(16.5894318446657,8.60865950196754,5.77600887199669));
#94878=CARTESIAN_POINT('Ctrl Pts',(16.5772785966527,8.78820347661546,5.51105638193783));
#94879=CARTESIAN_POINT('Ctrl Pts',(16.565105327834,8.95548506186407,5.23779982601913));
#94880=CARTESIAN_POINT('Ctrl Pts',(16.5529962083458,9.10963578220361,4.9573272331238));
#94881=CARTESIAN_POINT('Ctrl Pts',(16.546054400568,9.19800592921988,4.79654041218904));
#94882=CARTESIAN_POINT('Ctrl Pts',(16.5391336504345,9.28206138381152,4.633381391311));
#94883=CARTESIAN_POINT('Ctrl Pts',(16.5322495270048,9.3616427939792,4.4680487041676));
#94884=CARTESIAN_POINT('Ctrl Pts',(16.5322421302684,9.3617283012663,4.46787106029931));
#94885=CARTESIAN_POINT('Ctrl Pts',(16.5322347335515,9.36181380333707,4.46769341393065));
#94886=CARTESIAN_POINT('Ctrl Pts',(16.5322273368541,9.36189930019134,4.46751576506169));
#94887=CARTESIAN_POINT('Ctrl Pts',(16.5170311457259,9.53754884622812,4.10254393712876));
#94888=CARTESIAN_POINT('Ctrl Pts',(16.5019172397916,9.69118368878955,3.72701619034863));
#94889=CARTESIAN_POINT('Ctrl Pts',(16.4868192787626,9.82235262384252,3.34363337215857));
#94890=CARTESIAN_POINT('Ctrl Pts',(16.4717015541957,9.95369326169836,2.95974869806468));
#94891=CARTESIAN_POINT('Ctrl Pts',(16.4565997965269,10.0625082017002,2.56798774771891));
#94892=CARTESIAN_POINT('Ctrl Pts',(16.4414497127382,10.148314464651,2.17110439390891));
#94893=CARTESIAN_POINT('Ctrl Pts',(16.4306934647361,10.2092351471575,1.88932537267978));
#94894=CARTESIAN_POINT('Ctrl Pts',(16.4199129149323,10.2585571610524,1.60496520114311));
#94895=CARTESIAN_POINT('Ctrl Pts',(16.4090857225671,10.2961025663235,1.31902458207523));
#94896=CARTESIAN_POINT('Ctrl Pts',(16.3935638465982,10.3499277043803,0.909099767406544));
#94897=CARTESIAN_POINT('Ctrl Pts',(16.3780342325787,10.3797334643755,0.495806927140564));
#94898=CARTESIAN_POINT('Ctrl Pts',(16.3624725822917,10.3850267082106,0.0821820927440673));
#94899=CARTESIAN_POINT('Ctrl Pts',(16.347062775554,10.390268302965,-0.327406777482861));
#94900=CARTESIAN_POINT('Ctrl Pts',(16.3316215680962,10.3714728916886,-0.737320326153107));
#94901=CARTESIAN_POINT('Ctrl Pts',(16.3161261538691,10.3282038630816,-1.14458308412128));
#94902=CARTESIAN_POINT('Ctrl Pts',(16.3056238364201,10.2988774399556,-1.42061331517058));
#94903=CARTESIAN_POINT('Ctrl Pts',(16.2950966355493,10.2583094116598,-1.69542527755611));
#94904=CARTESIAN_POINT('Ctrl Pts',(16.2845375939976,10.2063769096049,-1.96808849315878));
#94905=CARTESIAN_POINT('Ctrl Pts',(16.2845327402885,10.2063530376221,-1.96821382914944));
#94906=CARTESIAN_POINT('Ctrl Pts',(16.2845278865727,10.2063291632382,-1.968339164686));
#94907=CARTESIAN_POINT('Ctrl Pts',(16.2845230328501,10.2063052864533,-1.96846449976846));
#94908=CARTESIAN_POINT('Ctrl Pts',(16.2675935855644,10.123024718359,-2.40562456484032));
#94909=CARTESIAN_POINT('Ctrl Pts',(16.2506612866968,10.0106855389608,-2.83726190886183));
#94910=CARTESIAN_POINT('Ctrl Pts',(16.233745990735,9.87114738724374,-3.26013776798451));
#94911=CARTESIAN_POINT('Ctrl Pts',(16.216491482196,9.72881099326279,-3.69149381038911));
#94912=CARTESIAN_POINT('Ctrl Pts',(16.1992546745454,9.55817403403809,-4.1137343165391));
#94913=CARTESIAN_POINT('Ctrl Pts',(16.1820559763094,9.36115909406157,-4.52343959234944));
#94914=CARTESIAN_POINT('Ctrl Pts',(16.164890733688,9.16452739564169,-4.93234789262239));
#94915=CARTESIAN_POINT('Ctrl Pts',(16.1477634692771,8.94162021511415,-5.3287707485719));
#94916=CARTESIAN_POINT('Ctrl Pts',(16.130693624495,8.69429725958992,-5.70931127112533));
#94917=CARTESIAN_POINT('Ctrl Pts',(16.1141347970773,8.45437837402047,-6.0784596095459));
#94918=CARTESIAN_POINT('Ctrl Pts',(16.0976300219097,8.19148340162108,-6.43266330773966));
#94919=CARTESIAN_POINT('Ctrl Pts',(16.0811959875537,7.9072640299243,-6.76880915533248));
#94920=CARTESIAN_POINT('Ctrl Pts',(16.0658638493284,7.64210146552994,-7.08241654397072));
#94921=CARTESIAN_POINT('Ctrl Pts',(16.0505932952338,7.35837773213623,-7.38030705297337));
#94922=CARTESIAN_POINT('Ctrl Pts',(16.0353967360999,7.05739941319241,-7.65993078023443));
#94923=CARTESIAN_POINT('Ctrl Pts',(16.0353826375841,7.05712018237657,-7.66019019945693));
#94924=CARTESIAN_POINT('Ctrl Pts',(16.0353685391679,7.05684093680483,-7.66044960295446));
#94925=CARTESIAN_POINT('Ctrl Pts',(16.0353544408512,7.05656167647816,-7.66070899072457));
#94926=CARTESIAN_POINT('Ctrl Pts',(16.0247062135628,6.84564093307695,-7.85662031816399));
#94927=CARTESIAN_POINT('Ctrl Pts',(16.0141145376293,6.62629924338843,-8.04356174782181));
#94928=CARTESIAN_POINT('Ctrl Pts',(16.0035064641038,6.39938093475859,-8.22098427349818));
#94929=CARTESIAN_POINT('Ctrl Pts',(15.9929182041099,6.17288645926429,-8.39807541319768));
#94930=CARTESIAN_POINT('Ctrl Pts',(15.9823136262558,5.9388434237568,-8.56568254415566));
#94931=CARTESIAN_POINT('Ctrl Pts',(15.9716228343142,5.69814046512725,-8.7232431399173));
#94932=CARTESIAN_POINT('Ctrl Pts',(15.9656811223411,5.56436294340201,-8.81081192653526));
#94933=CARTESIAN_POINT('Ctrl Pts',(15.9597128284198,5.42852913428555,-8.8952771974175));
#94934=CARTESIAN_POINT('Ctrl Pts',(15.9537062016035,5.29079848157823,-8.97654131976764));
#94935=CARTESIAN_POINT('Ctrl Pts',(15.9372437511037,4.91331805507004,-9.19926309565096));
#94936=CARTESIAN_POINT('Ctrl Pts',(15.9207847232432,4.52189152109994,-9.39845519891271));
#94937=CARTESIAN_POINT('Ctrl Pts',(15.9043256130699,4.11966267623208,-9.57279360603444));
#94938=CARTESIAN_POINT('Ctrl Pts',(15.8931339644216,3.84616041149253,-9.69133793667424));
#94939=CARTESIAN_POINT('Ctrl Pts',(15.8819422773134,3.56766274531486,-9.79839028808058));
#94940=CARTESIAN_POINT('Ctrl Pts',(15.8707494446982,3.28515006290952,-9.89352326144506));
#94941=CARTESIAN_POINT('Ctrl Pts',(15.8542197930833,2.86793340494329,-10.0340162859408));
#94942=CARTESIAN_POINT('Ctrl Pts',(15.8376603167854,2.44177297052336,-10.148525138475));
#94943=CARTESIAN_POINT('Ctrl Pts',(15.8210904408439,2.01002203189374,-10.235577364366));
#94944=CARTESIAN_POINT('Ctrl Pts',(15.8099406797445,1.71949965036582,-10.2941542375593));
#94945=CARTESIAN_POINT('Ctrl Pts',(15.7987861972866,1.42644628402294,-10.3403001921712));
#94946=CARTESIAN_POINT('Ctrl Pts',(15.7876327631621,1.13188391954781,-10.3735799091102));
#94947=CARTESIAN_POINT('Ctrl Pts',(15.771130668305,0.696063343958851,-10.422819007994));
#94948=CARTESIAN_POINT('Ctrl Pts',(15.7546308957414,0.256940656409019,-10.4438908172818));
#94949=CARTESIAN_POINT('Ctrl Pts',(15.7381516557369,-0.181833886135203,
-10.437269986716));
#94950=CARTESIAN_POINT('Ctrl Pts',(15.726937850918,-0.48041149518777,-10.43276463928));
#94951=CARTESIAN_POINT('Ctrl Pts',(15.7157335424594,-0.778828137337496,
-10.4154371764929));
#94952=CARTESIAN_POINT('Ctrl Pts',(15.7045443026975,-1.07594033927089,-10.3854492430376));
#94953=CARTESIAN_POINT('Ctrl Pts',(15.6907228568828,-1.44294652443974,-10.3484068160121));
#94954=CARTESIAN_POINT('Ctrl Pts',(15.6768856301063,-1.80819298526913,-10.2919584362545));
#94955=CARTESIAN_POINT('Ctrl Pts',(15.6630372227924,-2.16952225816341,-10.2163385634445));
#94956=CARTESIAN_POINT('Ctrl Pts',(15.6446444371282,-2.64942234486199,-10.1159039011018));
#94957=CARTESIAN_POINT('Ctrl Pts',(15.6262319401275,-3.12241154657823,-9.98164920097705));
#94958=CARTESIAN_POINT('Ctrl Pts',(15.6078102070798,-3.58380281291204,-9.81505615852526));
#94959=CARTESIAN_POINT('Ctrl Pts',(15.5893310518789,-4.04663227617918,-9.64794383098888));
#94960=CARTESIAN_POINT('Ctrl Pts',(15.5708426027203,-4.49779029758976,-9.44829177668541));
#94961=CARTESIAN_POINT('Ctrl Pts',(15.5523551122187,-4.93256648390252,-9.21764286844699));
#94962=CARTESIAN_POINT('Ctrl Pts',(15.5476710210738,-5.04272374316576,-9.1592044065821));
#94963=CARTESIAN_POINT('Ctrl Pts',(15.5429869898688,-5.15182953511281,-9.09877634468125));
#94964=CARTESIAN_POINT('Ctrl Pts',(15.5383031820876,-5.25980758410986,-9.03638419374356));
#94965=CARTESIAN_POINT('Ctrl Pts',(15.5382992206031,-5.2598989100963,-9.03633142352976));
#94966=CARTESIAN_POINT('Ctrl Pts',(15.5382952591187,-5.25999023527604,-9.03627865191097));
#94967=CARTESIAN_POINT('Ctrl Pts',(15.5382912976346,-5.26008155964901,-9.0362258788872));
#94968=CARTESIAN_POINT('Ctrl Pts',(15.5171750148634,-5.74687671076682,-8.75492471862091));
#94969=CARTESIAN_POINT('Ctrl Pts',(15.4960560699421,-6.21070130947555,-8.43371373452666));
#94970=CARTESIAN_POINT('Ctrl Pts',(15.474932053349,-6.64612860392156,-8.07752024759905));
#94971=CARTESIAN_POINT('Ctrl Pts',(15.4534657601675,-7.08861121231323,-7.71555528766612));
#94972=CARTESIAN_POINT('Ctrl Pts',(15.4319942296936,-7.50176993470843,-7.31746417752711));
#94973=CARTESIAN_POINT('Ctrl Pts',(15.4105149040284,-7.87988533001615,-6.88837076383642));
#94974=CARTESIAN_POINT('Ctrl Pts',(15.3975983738548,-8.10726392600793,-6.63033668438587));
#94975=CARTESIAN_POINT('Ctrl Pts',(15.3846790242293,-8.3219696627552,-6.36109075811446));
#94976=CARTESIAN_POINT('Ctrl Pts',(15.3717562937892,-8.52275198993461,-6.08174115861502));
#94977=CARTESIAN_POINT('Ctrl Pts',(15.3717550334894,-8.52277157139504,-6.0817139148172));
#94978=CARTESIAN_POINT('Ctrl Pts',(15.3717537731895,-8.52279115272298,-6.08168667092321));
#94979=CARTESIAN_POINT('Ctrl Pts',(15.3717525128895,-8.5228107339184,-6.08165942693309));
#94980=CARTESIAN_POINT('Ctrl Pts',(15.3467310365703,-8.91156771833097,-5.54076847442808));
#94981=CARTESIAN_POINT('Ctrl Pts',(15.3216830068258,-9.24809282431701,-4.96197684085428));
#94982=CARTESIAN_POINT('Ctrl Pts',(15.2966257752012,-9.52733228393928,-4.35651691105738));
#94983=CARTESIAN_POINT('Ctrl Pts',(15.2712591734181,-9.81001938523021,-3.74358164491119));
#94984=CARTESIAN_POINT('Ctrl Pts',(15.2458831434973,-10.033997612566,-3.10331726827767));
#94985=CARTESIAN_POINT('Ctrl Pts',(15.220514661223,-10.1940753908267,-2.44737864135056));
#94986=CARTESIAN_POINT('Ctrl Pts',(15.2153027494342,-10.2269630997016,-2.31261715954723));
#94987=CARTESIAN_POINT('Ctrl Pts',(15.2100911527011,-10.2571538033918,-2.17719403680014));
#94988=CARTESIAN_POINT('Ctrl Pts',(15.2048800126993,-10.284602740453,-2.04121024681705));
#94989=CARTESIAN_POINT('Ctrl Pts',(15.2048778801433,-10.2846139733877,-2.04115459813993));
#94990=CARTESIAN_POINT('Ctrl Pts',(15.2048757475874,-10.2846252058633,-2.04109894936894));
#94991=CARTESIAN_POINT('Ctrl Pts',(15.2048736150315,-10.2846364378797,-2.04104330050404));
#94992=CARTESIAN_POINT('Ctrl Pts',(15.1746996600235,-10.4435604621839,-1.25365649080174));
#94993=CARTESIAN_POINT('Ctrl Pts',(15.1445280227636,-10.5105303001057,-0.447479827685317));
#94994=CARTESIAN_POINT('Ctrl Pts',(15.1143457843457,-10.4858083682396,0.356187421247338));
#94995=CARTESIAN_POINT('Ctrl Pts',(15.0888798080307,-10.4649494735928,1.0342740112203));
#94996=CARTESIAN_POINT('Ctrl Pts',(15.0634062998675,-10.3788140387298,1.71057487855672));
#94997=CARTESIAN_POINT('Ctrl Pts',(15.0379180035962,-10.2275328575131,2.37228587195548));
#94998=CARTESIAN_POINT('Ctrl Pts',(15.0379163092748,-10.2275228011743,2.37232985885346));
#94999=CARTESIAN_POINT('Ctrl Pts',(15.0379146149534,-10.2275127445477,2.37237384568694));
#95000=CARTESIAN_POINT('Ctrl Pts',(15.0379129206319,-10.2275026876333,2.37241783245596));
#95001=CARTESIAN_POINT('Ctrl Pts',(15.0014002445382,-10.0107758993464,3.32033393562414));
#95002=CARTESIAN_POINT('Ctrl Pts',(14.9648672981753,-9.66037793399265,4.23831865808117));
#95003=CARTESIAN_POINT('Ctrl Pts',(14.9283181376167,-9.19199335040588,5.09164640273109));
#95004=CARTESIAN_POINT('Ctrl Pts',(14.9091157361511,-8.9459108501002,5.53997248420801));
#95005=CARTESIAN_POINT('Ctrl Pts',(14.8899088549882,-8.66726141839536,5.97045145954754));
#95006=CARTESIAN_POINT('Ctrl Pts',(14.8706980550175,-8.35832468417983,6.37805012061861));
#95007=CARTESIAN_POINT('Ctrl Pts',(14.8706952732979,-8.35827995021,6.37810914081331));
#95008=CARTESIAN_POINT('Ctrl Pts',(14.8706924915783,-8.35823521560515,6.37816816052829));
#95009=CARTESIAN_POINT('Ctrl Pts',(14.8706897098586,-8.35819048036528,6.37822717976354));
#95010=CARTESIAN_POINT('Ctrl Pts',(14.8215160136613,-7.56738574854429,7.42153645083545));
#95011=CARTESIAN_POINT('Ctrl Pts',(14.7723101054862,-6.57812722396956,8.31492006499422));
#95012=CARTESIAN_POINT('Ctrl Pts',(14.7230696429686,-5.45991725204736,8.99943735221583));
#95013=CARTESIAN_POINT('Ctrl Pts',(14.7164572422931,-5.30975512936079,9.09135977416325));
#95014=CARTESIAN_POINT('Ctrl Pts',(14.7098442193276,-5.15726760390441,9.17951573392545));
#95015=CARTESIAN_POINT('Ctrl Pts',(14.703230569178,-5.00262299218413,9.26376257707146));
#95016=CARTESIAN_POINT('Ctrl Pts',(14.7032289667057,-5.00258552214691,9.26378298988968));
#95017=CARTESIAN_POINT('Ctrl Pts',(14.7032273642332,-5.0025480519831,9.26380340247838));
#95018=CARTESIAN_POINT('Ctrl Pts',(14.7032257617608,-5.0025105816926,9.26382381483761));
#95019=CARTESIAN_POINT('Ctrl Pts',(14.669244157884,-4.20792557978978,9.696682868843));
#95020=CARTESIAN_POINT('Ctrl Pts',(14.635240371231,-3.35638823792469,10.0263304665229));
#95021=CARTESIAN_POINT('Ctrl Pts',(14.6012204808335,-2.47697562262436,10.2427935754682));
#95022=CARTESIAN_POINT('Ctrl Pts',(14.5793124068725,-1.91065290985073,10.3821911380463));
#95023=CARTESIAN_POINT('Ctrl Pts',(14.5573976373706,-1.33276908367124,10.4746496677617));
#95024=CARTESIAN_POINT('Ctrl Pts',(14.5354776096679,-0.751083147259138,
10.5174961589306));
#95025=CARTESIAN_POINT('Ctrl Pts',(14.5354752857554,-0.751021478212826,
10.5175007014201));
#95026=CARTESIAN_POINT('Ctrl Pts',(14.5354729618429,-0.750959809123862,
10.517505243352));
#95027=CARTESIAN_POINT('Ctrl Pts',(14.5354706379304,-0.750898139992239,
10.5175097847264));
#95028=CARTESIAN_POINT('Ctrl Pts',(14.4977727039571,0.249483258113779,10.5911788369562));
#95029=CARTESIAN_POINT('Ctrl Pts',(14.4600691123741,1.26109171283965,10.5181313904752));
#95030=CARTESIAN_POINT('Ctrl Pts',(14.4223521457816,2.243651747854,10.307475847821));
#95031=CARTESIAN_POINT('Ctrl Pts',(14.3839984443421,3.24279928366774,10.0932640349567));
#95032=CARTESIAN_POINT('Ctrl Pts',(14.3456309067135,4.21190728518531,9.73675766133124));
#95033=CARTESIAN_POINT('Ctrl Pts',(14.3072425487459,5.10859782900886,9.24757723114086));
#95034=CARTESIAN_POINT('Ctrl Pts',(14.2993282970171,5.29346207073116,9.14672641932464));
#95035=CARTESIAN_POINT('Ctrl Pts',(14.2914131642866,5.47524831837985,9.04023672261371));
#95036=CARTESIAN_POINT('Ctrl Pts',(14.2834970954803,5.65358523092099,8.92819272516899));
#95037=CARTESIAN_POINT('Ctrl Pts',(14.2834970378564,5.65358652909998,8.92819190956014));
#95038=CARTESIAN_POINT('Ctrl Pts',(14.2834969802325,5.65358782727877,8.92819109395101));
#95039=CARTESIAN_POINT('Ctrl Pts',(14.2834969226085,5.65358912545739,8.92819027834158));
#95040=CARTESIAN_POINT('Ctrl Pts',(14.2310050134086,6.8361511516281,8.18521952881629));
#95041=CARTESIAN_POINT('Ctrl Pts',(14.1784678415063,7.86707443414694,7.19799366623765));
#95042=CARTESIAN_POINT('Ctrl Pts',(14.125894307937,8.67403110736602,6.05305298708846));
#95043=CARTESIAN_POINT('Ctrl Pts',(14.0942621071495,9.15955707035689,5.36417036890058));
#95044=CARTESIAN_POINT('Ctrl Pts',(14.062616708956,9.56400502859731,4.6181920265712));
#95045=CARTESIAN_POINT('Ctrl Pts',(14.030959744161,9.87162305591945,3.83395878718145));
#95046=CARTESIAN_POINT('Ctrl Pts',(14.0309595161733,9.87162527132882,3.83395313927558));
#95047=CARTESIAN_POINT('Ctrl Pts',(14.0309592881856,9.87162748673317,3.83394749136769));
#95048=CARTESIAN_POINT('Ctrl Pts',(14.0309590601978,9.8716297021325,3.83394184345784));
#95049=CARTESIAN_POINT('Ctrl Pts',(13.9708935521266,10.4552974463881,2.34594698595516));
#95050=CARTESIAN_POINT('Ctrl Pts',(13.9107899888404,10.6903708731197,0.720259109315623));
#95051=CARTESIAN_POINT('Ctrl Pts',(13.8506391863266,10.5665434814408,-0.876732594070744));
#95052=CARTESIAN_POINT('Ctrl Pts',(13.8263984315185,10.5166410808947,-1.52031975657813));
#95053=CARTESIAN_POINT('Ctrl Pts',(13.8021500272319,10.4084495920086,-2.15924596122222));
#95054=CARTESIAN_POINT('Ctrl Pts',(13.777893464215,10.2412934788638,-2.78261871014446));
#95055=CARTESIAN_POINT('Ctrl Pts',(13.7778934103748,10.2412931078421,-2.78262009378993));
#95056=CARTESIAN_POINT('Ctrl Pts',(13.7778933565347,10.2412927368201,-2.78262147743535));
#95057=CARTESIAN_POINT('Ctrl Pts',(13.7778933026945,10.2412923657979,-2.78262286108066));
#95058=CARTESIAN_POINT('Ctrl Pts',(13.7049944159232,9.73893291691786,-4.65606116753667));
#95059=CARTESIAN_POINT('Ctrl Pts',(13.6320253888064,8.70401339334478,-6.38903511110609));
#95060=CARTESIAN_POINT('Ctrl Pts',(13.5589900344303,7.29765576143082,-7.73099682974251));
#95061=CARTESIAN_POINT('Ctrl Pts',(13.5474207740948,7.07487985095129,-7.94357202179451));
#95062=CARTESIAN_POINT('Ctrl Pts',(13.5358498473615,6.84278367381023,-8.14633580197754));
#95063=CARTESIAN_POINT('Ctrl Pts',(13.5242772670359,6.60200771009854,-8.33829239537025));
#95064=CARTESIAN_POINT('Ctrl Pts',(13.524277150712,6.60200528989507,-8.33829432485693));
#95065=CARTESIAN_POINT('Ctrl Pts',(13.5242770343881,6.60200286969076,-8.33829625434248));
#95066=CARTESIAN_POINT('Ctrl Pts',(13.5242769180642,6.60200044948554,-8.33829818382697));
#95067=CARTESIAN_POINT('Ctrl Pts',(13.4396479365417,4.84123157000304,-9.74205362168631));
#95068=CARTESIAN_POINT('Ctrl Pts',(13.3549284631214,2.61628154009548,-10.5678525763947));
#95069=CARTESIAN_POINT('Ctrl Pts',(13.2701176421097,0.361346148799453,-10.6519993370047));
#95070=CARTESIAN_POINT('Ctrl Pts',(13.2701176136022,0.361345390846792,-10.651999365289));
#95071=CARTESIAN_POINT('Ctrl Pts',(13.2701175850947,0.361344632894097,-10.6519993935732));
#95072=CARTESIAN_POINT('Ctrl Pts',(13.2701175565871,0.361343874941429,-10.6519994218574));
#95073=CARTESIAN_POINT('Ctrl Pts',(13.1853067394119,-1.89359143287809,-10.7361456800139));
#95074=CARTESIAN_POINT('Ctrl Pts',(13.100405505491,-4.17851204919358,-10.0786394971838));
#95075=CARTESIAN_POINT('Ctrl Pts',(13.0154126752357,-6.04716707214536,-8.80437263473603));
#95076=CARTESIAN_POINT('Ctrl Pts',(13.0154126427607,-6.04716778613988,-8.80437214785132));
#95077=CARTESIAN_POINT('Ctrl Pts',(13.0154126102858,-6.04716850013435,-8.80437166096652));
#95078=CARTESIAN_POINT('Ctrl Pts',(13.0154125778109,-6.04716921412875,-8.80437117408163));
#95079=CARTESIAN_POINT('Ctrl Pts',(12.9304197333074,-7.91582423070209,-7.53010362774895));
#95080=CARTESIAN_POINT('Ctrl Pts',(12.8453353201699,-9.36821421426481,-5.63907631050066));
#95081=CARTESIAN_POINT('Ctrl Pts',(12.7601592286344,-10.115835605735,-3.50019255496931));
#95082=CARTESIAN_POINT('Ctrl Pts',(12.7601592102983,-10.1158357666775,-3.50019209452601));
#95083=CARTESIAN_POINT('Ctrl Pts',(12.7601591919622,-10.11583592762,-3.50019163408269));
#95084=CARTESIAN_POINT('Ctrl Pts',(12.7601591736261,-10.1158360885624,-3.50019117363937));
#95085=CARTESIAN_POINT('Ctrl Pts',(12.674983063715,-10.8634573375402,-1.36130685095101));
#95086=CARTESIAN_POINT('Ctrl Pts',(12.5897152272118,-10.9063092390295,1.02543387185629));
#95087=CARTESIAN_POINT('Ctrl Pts',(12.5043551624473,-10.2388599315667,3.19702913316979));
#95088=CARTESIAN_POINT('Ctrl Pts',(12.4474484526043,-9.79389372659145,4.64475930737875));
#95089=CARTESIAN_POINT('Ctrl Pts',(12.3905007264825,-9.03323813748135,5.99686930213596));
#95090=CARTESIAN_POINT('Ctrl Pts',(12.3335121832258,-8.02849753094572,7.13448234478132));
#95091=CARTESIAN_POINT('Ctrl Pts',(12.2765236756013,-7.02375755262432,8.27209467613394));
#95092=CARTESIAN_POINT('Ctrl Pts',(12.2194943956609,-5.77493250040647,9.19520997384836));
#95093=CARTESIAN_POINT('Ctrl Pts',(12.1624238991661,-4.39051675511366,9.81981072751928));
#95094=CARTESIAN_POINT('Ctrl Pts',(12.1624238634828,-4.39051588950701,9.81981111805122));
#95095=CARTESIAN_POINT('Ctrl Pts',(12.1624238277994,-4.39051502390029,9.81981150858305));
#95096=CARTESIAN_POINT('Ctrl Pts',(12.1624237921161,-4.39051415829352,9.81981189911476));
#95097=CARTESIAN_POINT('Ctrl Pts',(12.1053532598864,-3.00609737783877,10.4444126700251));
#95098=CARTESIAN_POINT('Ctrl Pts',(12.0482416553095,-1.48609015210989,10.7705020422654));
#95099=CARTESIAN_POINT('Ctrl Pts',(11.9910889029797,0.0360657324407392,
10.7707675453198));
#95100=CARTESIAN_POINT('Ctrl Pts',(11.991088873251,0.0360665242078553,10.7707675454579));
#95101=CARTESIAN_POINT('Ctrl Pts',(11.9910888435224,0.0360673159750026,
10.7707675455959));
#95102=CARTESIAN_POINT('Ctrl Pts',(11.9910888137937,0.0360681077421199,
10.7707675457339));
#95103=CARTESIAN_POINT('Ctrl Pts',(11.9339360911498,1.55822320275625,10.7710327096852));
#95104=CARTESIAN_POINT('Ctrl Pts',(11.876742229104,3.08252202922973,10.4454709204958));
#95105=CARTESIAN_POINT('Ctrl Pts',(11.8195073882191,4.47068816216161,9.81823304479766));
#95106=CARTESIAN_POINT('Ctrl Pts',(11.8195072882203,4.47069058751851,9.81823194890887));
#95107=CARTESIAN_POINT('Ctrl Pts',(11.8195071882216,4.47069301287499,9.81823085301915));
#95108=CARTESIAN_POINT('Ctrl Pts',(11.8195070882228,4.47069543823106,9.81822975712852));
#95109=CARTESIAN_POINT('Ctrl Pts',(11.7647262028572,5.79934320531001,9.21788382628587));
#95110=CARTESIAN_POINT('Ctrl Pts',(11.7099064063734,7.00328222838745,8.34115772527208));
#95111=CARTESIAN_POINT('Ctrl Pts',(11.6550500153073,7.99116085304476,7.26550933943654));
#95112=CARTESIAN_POINT('Ctrl Pts',(11.6334881613261,8.37945644161783,6.84271496708076));
#95113=CARTESIAN_POINT('Ctrl Pts',(11.6119206340189,8.73437210179503,6.38918775421612));
#95114=CARTESIAN_POINT('Ctrl Pts',(11.5903474976357,9.05036237110234,5.90963037900502));
#95115=CARTESIAN_POINT('Ctrl Pts',(11.5903472031011,9.05036668526645,5.90962383168564));
#95116=CARTESIAN_POINT('Ctrl Pts',(11.5903469085666,9.05037099942332,5.90961728436137));
#95117=CARTESIAN_POINT('Ctrl Pts',(11.590346614032,9.05037531357291,5.90961073703228));
#95118=CARTESIAN_POINT('Ctrl Pts',(11.5521177424565,9.6103268421719,5.05980549672893));
#95119=CARTESIAN_POINT('Ctrl Pts',(11.5138705621619,10.04802451717,4.12825797978597));
#95120=CARTESIAN_POINT('Ctrl Pts',(11.4756033482928,10.3475045060857,3.15400626050042));
#95121=CARTESIAN_POINT('Ctrl Pts',(11.4756027701249,10.3475090308397,3.15399154082099));
#95122=CARTESIAN_POINT('Ctrl Pts',(11.4756021919569,10.3475135555622,3.15397682113182));
#95123=CARTESIAN_POINT('Ctrl Pts',(11.4756016137889,10.3475180802532,3.15396210143288));
#95124=CARTESIAN_POINT('Ctrl Pts',(11.4445194665227,10.5907641957754,2.36263521950445));
#95125=CARTESIAN_POINT('Ctrl Pts',(11.413423181403,10.7428069207936,1.54311887101492));
#95126=CARTESIAN_POINT('Ctrl Pts',(11.3823157836203,10.8009630036407,0.716963741758189));
#95127=CARTESIAN_POINT('Ctrl Pts',(11.3559768003265,10.8502044125571,0.0174489093190168));
#95128=CARTESIAN_POINT('Ctrl Pts',(11.3296298305488,10.8321379003915,-0.686825019406177));
#95129=CARTESIAN_POINT('Ctrl Pts',(11.3032760407308,10.7451581043584,-1.3827939101456));
#95130=CARTESIAN_POINT('Ctrl Pts',(11.3032751042502,10.7451550135354,-1.38281864136757));
#95131=CARTESIAN_POINT('Ctrl Pts',(11.3032741677695,10.7451519226254,-1.38284337257904));
#95132=CARTESIAN_POINT('Ctrl Pts',(11.3032732312888,10.7451488316284,-1.38286810378004));
#95133=CARTESIAN_POINT('Ctrl Pts',(11.276427626827,10.6565408306116,-2.09182455745042));
#95134=CARTESIAN_POINT('Ctrl Pts',(11.2495747669126,10.4964033124759,-2.7921500741643));
#95135=CARTESIAN_POINT('Ctrl Pts',(11.2227120936351,10.2695128164393,-3.47058196733028));
#95136=CARTESIAN_POINT('Ctrl Pts',(11.1961226945325,10.0449304791044,-4.14211216780692));
#95137=CARTESIAN_POINT('Ctrl Pts',(11.1695236812975,9.75494559229498,-4.79219337877807));
#95138=CARTESIAN_POINT('Ctrl Pts',(11.1429127933632,9.40414738125851,-5.40793884114943));
#95139=CARTESIAN_POINT('Ctrl Pts',(11.1388448428612,9.35052159612138,-5.50206655567435));
#95140=CARTESIAN_POINT('Ctrl Pts',(11.1347766152765,9.29547462001186,-5.59539182062596));
#95141=CARTESIAN_POINT('Ctrl Pts',(11.1307081029784,9.23902277573395,-5.68786851634614));
#95142=CARTESIAN_POINT('Ctrl Pts',(11.1307077878792,9.23901840363643,-5.68787567850598));
#95143=CARTESIAN_POINT('Ctrl Pts',(11.1307074727799,9.23901403153045,-5.6878828406608));
#95144=CARTESIAN_POINT('Ctrl Pts',(11.1307071576807,9.23900965941608,-5.68789000281049));
#95145=CARTESIAN_POINT('Ctrl Pts',(11.1087126902279,8.93382856876452,-6.18782034961866));
#95146=CARTESIAN_POINT('Ctrl Pts',(11.0867101411768,8.58762339757433,-6.66296969610626));
#95147=CARTESIAN_POINT('Ctrl Pts',(11.0647020280532,8.20552966826705,-7.10739697135233));
#95148=CARTESIAN_POINT('Ctrl Pts',(11.0430057911313,7.82885057584139,-7.54552628321619));
#95149=CARTESIAN_POINT('Ctrl Pts',(11.021304148256,7.41729343552421,-7.95379682567712));
#95150=CARTESIAN_POINT('Ctrl Pts',(10.9996002320039,6.97582456482181,-8.32653423594124));
#95151=CARTESIAN_POINT('Ctrl Pts',(10.9856977369036,6.69304063124135,-8.56529206930643));
#95152=CARTESIAN_POINT('Ctrl Pts',(10.9717943237775,6.39798460599023,-8.7894707983027));
#95153=CARTESIAN_POINT('Ctrl Pts',(10.9578909660409,6.09197018180152,-8.99758667411823));
#95154=CARTESIAN_POINT('Ctrl Pts',(10.9578863159333,6.09186783242472,-8.99765628041293));
#95155=CARTESIAN_POINT('Ctrl Pts',(10.9578816658257,6.09176548182219,-8.99772588491082));
#95156=CARTESIAN_POINT('Ctrl Pts',(10.9578770157181,6.09166312999389,-8.99779548761196));
#95157=CARTESIAN_POINT('Ctrl Pts',(10.9383945955149,5.66284265850238,-9.28940789567403));
#95158=CARTESIAN_POINT('Ctrl Pts',(10.918910893143,5.2124075741954,-9.54944778025722));
#95159=CARTESIAN_POINT('Ctrl Pts',(10.8994243975854,4.74555262774488,-9.77638020724774));
#95160=CARTESIAN_POINT('Ctrl Pts',(10.8798301960368,4.27611727505877,-10.0045669378589));
#95161=CARTESIAN_POINT('Ctrl Pts',(10.8602331571735,3.79008010926782,-10.1992803732407));
#95162=CARTESIAN_POINT('Ctrl Pts',(10.8406301278026,3.29267026192362,-10.3589639008086));
#95163=CARTESIAN_POINT('Ctrl Pts',(10.8211593846148,2.798617061599,-10.5175698436849));
#95164=CARTESIAN_POINT('Ctrl Pts',(10.8016827442102,2.29334380119201,-10.6416182908074));
#95165=CARTESIAN_POINT('Ctrl Pts',(10.7821955326892,1.78192541675302,-10.7295699425325));
#95166=CARTESIAN_POINT('Ctrl Pts',(10.7633071045453,1.28622138051714,-10.8148191046282));
#95167=CARTESIAN_POINT('Ctrl Pts',(10.7444087737147,0.784743322812868,-10.8661567175532));
#95168=CARTESIAN_POINT('Ctrl Pts',(10.7254944885072,0.282074720709333,-10.8821514898605));
#95169=CARTESIAN_POINT('Ctrl Pts',(10.7164126013939,0.0407132603268094,
-10.8898315430534));
#95170=CARTESIAN_POINT('Ctrl Pts',(10.7073270064101,-0.20092318772183,-10.889362630306));
#95171=CARTESIAN_POINT('Ctrl Pts',(10.6982368407905,-0.442329630350118,
-10.8805826918547));
#95172=CARTESIAN_POINT('Ctrl Pts',(10.6982355033686,-0.442365148102834,
-10.8805814000761));
#95173=CARTESIAN_POINT('Ctrl Pts',(10.6982341659467,-0.442400665849766,
-10.8805801081155));
#95174=CARTESIAN_POINT('Ctrl Pts',(10.6982328285249,-0.442436183590935,
-10.880578815973));
#95175=CARTESIAN_POINT('Ctrl Pts',(10.6817905060337,-0.8790928361865,-10.8646931591655));
#95176=CARTESIAN_POINT('Ctrl Pts',(10.6653483153528,-1.31487411611491,-10.8213005155887));
#95177=CARTESIAN_POINT('Ctrl Pts',(10.6489086997776,-1.74664947052937,-10.7516253321206));
#95178=CARTESIAN_POINT('Ctrl Pts',(10.6324561907571,-2.17876346253965,-10.6818955030217));
#95179=CARTESIAN_POINT('Ctrl Pts',(10.6160062390361,-2.60686458099451,-10.5858427064414));
#95180=CARTESIAN_POINT('Ctrl Pts',(10.5995600031669,-3.02785330284519,-10.4647288798457));
#95181=CARTESIAN_POINT('Ctrl Pts',(10.5890775919128,-3.2961807761276,-10.3875340159854));
#95182=CARTESIAN_POINT('Ctrl Pts',(10.5785966663672,-3.56161967797226,-10.3001588571056));
#95183=CARTESIAN_POINT('Ctrl Pts',(10.5681172994041,-3.82337729854416,-10.202935230923));
#95184=CARTESIAN_POINT('Ctrl Pts',(10.5517035494577,-4.23336619823257,-10.050654630896));
#95185=CARTESIAN_POINT('Ctrl Pts',(10.5352900090993,-4.6344161363684,-9.87418397575912));
#95186=CARTESIAN_POINT('Ctrl Pts',(10.5188765390162,-5.02358347131284,-9.6745851249155));
#95187=CARTESIAN_POINT('Ctrl Pts',(10.5026744444006,-5.40773904293458,-9.47755674212017));
#95188=CARTESIAN_POINT('Ctrl Pts',(10.4864724376194,-5.78031654354983,-9.2579911487857));
#95189=CARTESIAN_POINT('Ctrl Pts',(10.4702713454141,-6.13843979100847,-9.01688710342178));
#95190=CARTESIAN_POINT('Ctrl Pts',(10.4595375757754,-6.37570851287987,-8.85714754703308));
#95191=CARTESIAN_POINT('Ctrl Pts',(10.4488042284911,-6.60663158645119,-8.68795323280413));
#95192=CARTESIAN_POINT('Ctrl Pts',(10.4380716961009,-6.83036021601855,-8.50959177631948));
#95193=CARTESIAN_POINT('Ctrl Pts',(10.4380538739088,-6.83073173454504,-8.50929559345891));
#95194=CARTESIAN_POINT('Ctrl Pts',(10.4380360517174,-6.83110323324723,-8.50899938533706));
#95195=CARTESIAN_POINT('Ctrl Pts',(10.4380182295268,-6.83147471212122,-8.50870315195564));
#95196=CARTESIAN_POINT('Ctrl Pts',(10.4240239199098,-7.12316670974611,-8.27609528959938));
#95197=CARTESIAN_POINT('Ctrl Pts',(10.4100301843033,-7.40262900123163,-8.027914184564));
#95198=CARTESIAN_POINT('Ctrl Pts',(10.3960314849731,-7.66869202103855,-7.76587198354066));
#95199=CARTESIAN_POINT('Ctrl Pts',(10.3813641610424,-7.94746309865262,-7.49131377243469));
#95200=CARTESIAN_POINT('Ctrl Pts',(10.3666914133372,-8.21152444193502,-7.20153998553732));
#95201=CARTESIAN_POINT('Ctrl Pts',(10.3520053807219,-8.4595868661027,-6.89849586245379));
#95202=CARTESIAN_POINT('Ctrl Pts',(10.3373193481065,-8.70764929027039,-6.59545173937024));
#95203=CARTESIAN_POINT('Ctrl Pts',(10.3226201383575,-8.93971350484724,-6.27913822071352));
#95204=CARTESIAN_POINT('Ctrl Pts',(10.307897451588,-9.15453835988915,-5.95146045198642));
#95205=CARTESIAN_POINT('Ctrl Pts',(10.3078926968971,-9.15460773756404,-5.9513546284694));
#95206=CARTESIAN_POINT('Ctrl Pts',(10.3078879422038,-9.15467711344128,-5.95124880376669));
#95207=CARTESIAN_POINT('Ctrl Pts',(10.307883187508,-9.15474648752083,-5.95114297787839));
#95208=CARTESIAN_POINT('Ctrl Pts',(10.2950118141782,-9.34254812824675,-5.66466313436061));
#95209=CARTESIAN_POINT('Ctrl Pts',(10.2821249864793,-9.51713738035586,-5.36954274635421));
#95210=CARTESIAN_POINT('Ctrl Pts',(10.2692307460949,-9.67765166003237,-5.06699870239409));
#95211=CARTESIAN_POINT('Ctrl Pts',(10.2563266189396,-9.83828901542888,-4.76422268015691));
#95212=CARTESIAN_POINT('Ctrl Pts',(10.2434150115707,-9.98482905816014,-4.4540111652875));
#95213=CARTESIAN_POINT('Ctrl Pts',(10.230506763713,-10.1163788997621,-4.1376276009189));
#95214=CARTESIAN_POINT('Ctrl Pts',(10.2176290652104,-10.247617408418,-3.82199280694777));
#95215=CARTESIAN_POINT('Ctrl Pts',(10.2047547508469,-10.363935759884,-3.5002148636008));
#95216=CARTESIAN_POINT('Ctrl Pts',(10.1918974615459,-10.4644310230913,-3.17359719965375));
#95217=CARTESIAN_POINT('Ctrl Pts',(10.1869804590058,-10.5028633436909,-3.04868907589055));
#95218=CARTESIAN_POINT('Ctrl Pts',(10.1820659724405,-10.5389813997489,-2.92307366388694));
#95219=CARTESIAN_POINT('Ctrl Pts',(10.1771548409931,-10.5727344554174,-2.79682587267854));
#95220=CARTESIAN_POINT('Ctrl Pts',(10.1771531125453,-10.5727463346347,-2.79678144040639));
#95221=CARTESIAN_POINT('Ctrl Pts',(10.1771513840978,-10.5727582135592,-2.79673700805592));
#95222=CARTESIAN_POINT('Ctrl Pts',(10.1771496556507,-10.5727700921907,-2.79669257562713));
#95223=CARTESIAN_POINT('Ctrl Pts',(10.1600923132765,-10.6899954840456,-2.35820697423387));
#95224=CARTESIAN_POINT('Ctrl Pts',(10.1430357320927,-10.7791375076164,-1.912114575594));
#95225=CARTESIAN_POINT('Ctrl Pts',(10.125984049529,-10.8402521913098,-1.46190596578374));
#95226=CARTESIAN_POINT('Ctrl Pts',(10.1089323669653,-10.9013668750032,-1.01169735597347));
#95227=CARTESIAN_POINT('Ctrl Pts',(10.0918856236707,-10.9344533695982,-0.557371477539993));
#95228=CARTESIAN_POINT('Ctrl Pts',(10.0748490921613,-10.93952229677,-0.10245759066365));
#95229=CARTESIAN_POINT('Ctrl Pts',(10.0592286476227,-10.9441698915995,0.314643574314747));
#95230=CARTESIAN_POINT('Ctrl Pts',(10.0436100742942,-10.9253234912044,0.732257491259243));
#95231=CARTESIAN_POINT('Ctrl Pts',(10.0279840463942,-10.8831643611597,1.14755960306089));
#95232=CARTESIAN_POINT('Ctrl Pts',(10.0123763869989,-10.8410547894665,1.56237352433246));
#95233=CARTESIAN_POINT('Ctrl Pts',(9.99676130151046,-10.775688316319,1.97488078916013));
#95234=CARTESIAN_POINT('Ctrl Pts',(9.98112802898836,-10.687259935448,2.38231663280635));
#95235=CARTESIAN_POINT('Ctrl Pts',(9.96557287319891,-10.5992734157533,2.78771659069503));
#95236=CARTESIAN_POINT('Ctrl Pts',(9.94999978403184,-10.4884559072605,3.18809569448487));
#95237=CARTESIAN_POINT('Ctrl Pts',(9.93439608171986,-10.3549982254007,3.58078175974953));
#95238=CARTESIAN_POINT('Ctrl Pts',(9.92831144655146,-10.3029566465303,3.73390897245062));
#95239=CARTESIAN_POINT('Ctrl Pts',(9.92222212763273,-10.2474723168187,3.88586693574198));
#95240=CARTESIAN_POINT('Ctrl Pts',(9.91612723880565,-10.1885559866788,4.0364992796125));
#95241=CARTESIAN_POINT('Ctrl Pts',(9.91612511809011,-10.1885354867516,4.03655169211108));
#95242=CARTESIAN_POINT('Ctrl Pts',(9.91612299737397,-10.1885149864093,4.03660410444787));
#95243=CARTESIAN_POINT('Ctrl Pts',(9.91612087665721,-10.1884944856518,4.0366565166229));
#95244=CARTESIAN_POINT('Ctrl Pts',(9.90424230788015,-10.0736655449819,4.33022784125202));
#95245=CARTESIAN_POINT('Ctrl Pts',(9.89234445392564,-9.94580834537035,4.6187281425354));
#95246=CARTESIAN_POINT('Ctrl Pts',(9.8804433786764,-9.80555473114634,4.90117931235152));
#95247=CARTESIAN_POINT('Ctrl Pts',(9.86853193699502,-9.66517894900519,5.18387651127215));
#95248=CARTESIAN_POINT('Ctrl Pts',(9.85661725743133,-9.51238449680269,5.46051361479744));
#95249=CARTESIAN_POINT('Ctrl Pts',(9.84471830064194,-9.34783275583516,5.73006603077023));
#95250=CARTESIAN_POINT('Ctrl Pts',(9.83932807489827,-9.27329084043639,5.85217323710445));
#95251=CARTESIAN_POINT('Ctrl Pts',(9.83394111531266,-9.19633666345336,5.97282604479221));
#95252=CARTESIAN_POINT('Ctrl Pts',(9.8285593516629,-9.11703410606218,6.09192663296797));
#95253=CARTESIAN_POINT('Ctrl Pts',(9.81375791075102,-8.89892863102168,6.41948845715402));
#95254=CARTESIAN_POINT('Ctrl Pts',(9.79897061721313,-8.66324738954729,6.73542959730272));
#95255=CARTESIAN_POINT('Ctrl Pts',(9.78418769195425,-8.41148443703231,7.03808188949212));
#95256=CARTESIAN_POINT('Ctrl Pts',(9.76987296525404,-8.16769521430548,7.33114870624292));
#95257=CARTESIAN_POINT('Ctrl Pts',(9.75556231771307,-7.9088263515839,7.61175589603912));
#95258=CARTESIAN_POINT('Ctrl Pts',(9.74124597042629,-7.63618864220333,7.87838006913979));
#95259=CARTESIAN_POINT('Ctrl Pts',(9.73131841879647,-7.44713029639129,8.06326837837052));
#95260=CARTESIAN_POINT('Ctrl Pts',(9.7213931377954,-7.25139733094209,8.24141573136087));
#95261=CARTESIAN_POINT('Ctrl Pts',(9.71149210718083,-7.04932308698385,8.41213375761355));
#95262=CARTESIAN_POINT('Ctrl Pts',(9.70688153567211,-6.95522401910804,8.49163130675839));
#95263=CARTESIAN_POINT('Ctrl Pts',(9.70227624358616,-6.85975041147126,8.56951733569182));
#95264=CARTESIAN_POINT('Ctrl Pts',(9.69767849528538,-6.76293888476845,8.64571985600731));
#95265=CARTESIAN_POINT('Ctrl Pts',(9.68554012472698,-6.50734982060734,8.846899731147));
#95266=CARTESIAN_POINT('Ctrl Pts',(9.67336295672748,-6.24287541021037,9.03690912957521));
#95267=CARTESIAN_POINT('Ctrl Pts',(9.66113765782758,-5.97046298774467,9.21476964386224));
#95268=CARTESIAN_POINT('Ctrl Pts',(9.65879580270697,-5.91828017964376,9.24884026737405));
#95269=CARTESIAN_POINT('Ctrl Pts',(9.6564521725576,-5.86580607557735,9.28246524616543));
#95270=CARTESIAN_POINT('Ctrl Pts',(9.65410668749291,-5.81304730592889,9.31563792018204));
#95271=CARTESIAN_POINT('Ctrl Pts',(9.64680021884648,-5.64869738016574,9.41897479760209));
#95272=CARTESIAN_POINT('Ctrl Pts',(9.63947579902925,-5.48158521451971,9.51792205096366));
#95273=CARTESIAN_POINT('Ctrl Pts',(9.63213061486297,-5.31200090258064,9.61242722059944));
#95274=CARTESIAN_POINT('Ctrl Pts',(9.62097856935138,-5.05452444971298,9.75591252049098));
#95275=CARTESIAN_POINT('Ctrl Pts',(9.60986719987094,-4.79106445159546,9.88856816815131));
#95276=CARTESIAN_POINT('Ctrl Pts',(9.59877852810167,-4.52266849084066,10.0102947770022));
#95277=CARTESIAN_POINT('Ctrl Pts',(9.58798006298252,-4.26129684231154,10.1288356236519));
#95278=CARTESIAN_POINT('Ctrl Pts',(9.57720302703863,-3.99524420678122,10.2370126121934));
#95279=CARTESIAN_POINT('Ctrl Pts',(9.5664284793928,-3.72543397488881,10.3347516488405));
#95280=CARTESIAN_POINT('Ctrl Pts',(9.55408976253708,-3.4164546872633,10.4466797165962));
#95281=CARTESIAN_POINT('Ctrl Pts',(9.54175218849227,-3.10249573876305,10.5449422787711));
#95282=CARTESIAN_POINT('Ctrl Pts',(9.5294102067266,-2.78471433156453,10.6292485760067));
#95283=CARTESIAN_POINT('Ctrl Pts',(9.52718922994239,-2.72752861040209,10.6444197480663));
#95284=CARTESIAN_POINT('Ctrl Pts',(9.52496811040537,-2.67021906674301,10.659138842928));
#95285=CARTESIAN_POINT('Ctrl Pts',(9.52274681574758,-2.61279239892922,10.6734039929166));
#95286=CARTESIAN_POINT('Ctrl Pts',(9.50957782861494,-2.27233731934088,10.757975202767));
#95287=CARTESIAN_POINT('Ctrl Pts',(9.49640208211643,-1.92774945005703,10.8265966109633));
#95288=CARTESIAN_POINT('Ctrl Pts',(9.4832339184354,-1.58054382301562,10.8787209774921));
#95289=CARTESIAN_POINT('Ctrl Pts',(9.47455588396265,-1.35172965624335,10.9130717845267));
#95290=CARTESIAN_POINT('Ctrl Pts',(9.46588117844456,-1.12177946918322,10.9402572872661));
#95291=CARTESIAN_POINT('Ctrl Pts',(9.45721419258468,-0.891138086337386,
10.9601155441168));
#95292=CARTESIAN_POINT('Ctrl Pts',(9.44738282224253,-0.629510700803001,
10.9826417003384));
#95293=CARTESIAN_POINT('Ctrl Pts',(9.43756127496004,-0.366999143975139,
10.9957394251776));
#95294=CARTESIAN_POINT('Ctrl Pts',(9.42772347258561,-0.104322862781696,
10.9994016033688));
#95295=CARTESIAN_POINT('Ctrl Pts',(9.41789152627671,0.158197057320262,11.0030616016061));
#95296=CARTESIAN_POINT('Ctrl Pts',(9.40804341476379,0.420881371031134,10.9972978968109));
#95297=CARTESIAN_POINT('Ctrl Pts',(9.39815138092922,0.683062679165209,10.9821145355309));
#95298=CARTESIAN_POINT('Ctrl Pts',(9.39597581796097,0.74072442542335,10.978775246656));
#95299=CARTESIAN_POINT('Ctrl Pts',(9.39379812055835,0.798362040111534,10.9749803553368));
#95300=CARTESIAN_POINT('Ctrl Pts',(9.39161797327781,0.855968760489002,10.9707299301633));
#95301=CARTESIAN_POINT('Ctrl Pts',(9.39161740661138,0.855983733695031,10.9707288253879));
#95302=CARTESIAN_POINT('Ctrl Pts',(9.39161683994479,0.85599870689897,10.9707277205816));
#95303=CARTESIAN_POINT('Ctrl Pts',(9.39161627327803,0.856013680100825,10.9707266157446));
#95304=CARTESIAN_POINT('Ctrl Pts',(9.37394596126279,1.32292151416537,10.9362745949034));
#95305=CARTESIAN_POINT('Ctrl Pts',(9.35629746476006,1.78747736955613,10.870794368147));
#95306=CARTESIAN_POINT('Ctrl Pts',(9.33867148090217,2.24598873793039,10.7758863557475));
#95307=CARTESIAN_POINT('Ctrl Pts',(9.3214200148757,2.69475763265044,10.6829949537839));
#95308=CARTESIAN_POINT('Ctrl Pts',(9.30419010193193,3.1377356506204,10.5619136932599));
#95309=CARTESIAN_POINT('Ctrl Pts',(9.28698169162748,3.57150226341286,10.4141705750997));
#95310=CARTESIAN_POINT('Ctrl Pts',(9.28283455480297,3.67603774701233,10.3785652568251));
#95311=CARTESIAN_POINT('Ctrl Pts',(9.27868866402646,3.78003845909759,10.3414115615419));
#95312=CARTESIAN_POINT('Ctrl Pts',(9.27454401349585,3.88345694555816,10.3027310589707));
#95313=CARTESIAN_POINT('Ctrl Pts',(9.26173983131444,4.20295050280404,10.1832343250163));
#95314=CARTESIAN_POINT('Ctrl Pts',(9.24893344583012,4.51708431878307,10.0491376720003));
#95315=CARTESIAN_POINT('Ctrl Pts',(9.23614139349798,4.82448797231439,9.90086735627349));
#95316=CARTESIAN_POINT('Ctrl Pts',(9.22345462903181,5.12936147088459,9.75381741275308));
#95317=CARTESIAN_POINT('Ctrl Pts',(9.21078201863816,5.4276151908266,9.59282545578268));
#95318=CARTESIAN_POINT('Ctrl Pts',(9.19814075939927,5.71786135179877,9.41830487169184));
#95319=CARTESIAN_POINT('Ctrl Pts',(9.1892140139505,5.92282143904346,9.29506550128486));
#95320=CARTESIAN_POINT('Ctrl Pts',(9.18030293369877,6.12378739923758,9.16507986810741));
#95321=CARTESIAN_POINT('Ctrl Pts',(9.1714135761887,6.32025498189214,9.02849560697713));
#95322=CARTESIAN_POINT('Ctrl Pts',(9.15963076376754,6.58067207847463,8.84745364452293));
#95323=CARTESIAN_POINT('Ctrl Pts',(9.14778454022514,6.83347258097126,8.65533909466343));
#95324=CARTESIAN_POINT('Ctrl Pts',(9.1358582875849,7.07756053330412,8.45272405369443));
#95325=CARTESIAN_POINT('Ctrl Pts',(9.13356736965186,7.12444747123071,8.41380366144192));
#95326=CARTESIAN_POINT('Ctrl Pts',(9.13127348637172,7.17101308047551,8.37449583067599));
#95327=CARTESIAN_POINT('Ctrl Pts',(9.12897649995789,7.21724981291642,8.33480463150905));
#95328=CARTESIAN_POINT('Ctrl Pts',(9.12142168216154,7.36932301935194,8.20425976802198));
#95329=CARTESIAN_POINT('Ctrl Pts',(9.11383338299965,7.51783794744756,8.0695678436588));
#95330=CARTESIAN_POINT('Ctrl Pts',(9.10620600819097,7.66265230395864,7.93101579732647));
#95331=CARTESIAN_POINT('Ctrl Pts',(9.08745532896714,8.0186552032591,7.59040778451148));
#95332=CARTESIAN_POINT('Ctrl Pts',(9.06880435751816,8.35096412388481,7.22520305099041));
#95333=CARTESIAN_POINT('Ctrl Pts',(9.05026519954328,8.65724948375359,6.83929469703732));
#95334=CARTESIAN_POINT('Ctrl Pts',(9.04703363894821,8.7106380843115,6.77202701251596));
#95335=CARTESIAN_POINT('Ctrl Pts',(9.04380546309821,8.7632359176161,6.70413016195419));
#95336=CARTESIAN_POINT('Ctrl Pts',(9.04058071946552,8.81503055537896,6.63562463964333));
#95337=CARTESIAN_POINT('Ctrl Pts',(9.02766259082993,9.02251675256724,6.36119564612947));
#95338=CARTESIAN_POINT('Ctrl Pts',(9.01474413415878,9.21737630810118,6.07712410118515));
#95339=CARTESIAN_POINT('Ctrl Pts',(9.00182002655774,9.39887812276248,5.78458511222852));
#95340=CARTESIAN_POINT('Ctrl Pts',(9.00011373135565,9.42284075794672,5.74596288091574));
#95341=CARTESIAN_POINT('Ctrl Pts',(8.99840733764636,9.44657049929936,5.70719301937561));
#95342=CARTESIAN_POINT('Ctrl Pts',(8.99670083317216,9.47006560548064,5.66827819795195));
#95343=CARTESIAN_POINT('Ctrl Pts',(8.98502581887399,9.6308068779185,5.40204326953455));
#95344=CARTESIAN_POINT('Ctrl Pts',(8.97340281255853,9.78033206732416,5.12881471684042));
#95345=CARTESIAN_POINT('Ctrl Pts',(8.96180410195002,9.91811115413175,4.84969521228766));
#95346=CARTESIAN_POINT('Ctrl Pts',(8.95020453516649,10.055900411295,4.57055510413893));
#95347=CARTESIAN_POINT('Ctrl Pts',(8.93862916408886,10.1819423440877,4.28552370912528));
#95348=CARTESIAN_POINT('Ctrl Pts',(8.92704867470572,10.2957451194813,3.99566856776635));
#95349=CARTESIAN_POINT('Ctrl Pts',(8.9154766341582,10.4094648672143,3.70602489747416));
#95350=CARTESIAN_POINT('Ctrl Pts',(8.90389948983685,10.5109639151262,3.41156494279894));
#95351=CARTESIAN_POINT('Ctrl Pts',(8.89228712084619,10.5997813700364,3.11331137960146));
#95352=CARTESIAN_POINT('Ctrl Pts',(8.8834668673401,10.6672432693874,2.88677086589459));
#95353=CARTESIAN_POINT('Ctrl Pts',(8.87462630058372,10.727389516561,2.65804087414844));
#95354=CARTESIAN_POINT('Ctrl Pts',(8.8657515832713,10.7800262063301,2.42755112095466));
#95355=CARTESIAN_POINT('Ctrl Pts',(8.86573523696568,10.7801231576343,2.42712658281845));
#95356=CARTESIAN_POINT('Ctrl Pts',(8.86571889054395,10.7802200834631,2.42670203870736));
#95357=CARTESIAN_POINT('Ctrl Pts',(8.86570254400602,10.7803169838174,2.42627748862456));
#95358=CARTESIAN_POINT('Ctrl Pts',(8.85391139131615,10.8502135501323,2.12003925806498));
#95359=CARTESIAN_POINT('Ctrl Pts',(8.8420497849596,10.9069009882179,1.81079706389893));
#95360=CARTESIAN_POINT('Ctrl Pts',(8.83014882942962,10.9503521553503,1.49965539489733));
#95361=CARTESIAN_POINT('Ctrl Pts',(8.81819935166284,10.9939804803434,1.18724514794795));
#95362=CARTESIAN_POINT('Ctrl Pts',(8.80621005785882,11.0242635506925,0.872919835380537));
#95363=CARTESIAN_POINT('Ctrl Pts',(8.79421476148775,11.0411678356221,0.557849550303085));
#95364=CARTESIAN_POINT('Ctrl Pts',(8.78846357505489,11.0492726536389,0.406788009772473));
#95365=CARTESIAN_POINT('Ctrl Pts',(8.7827110572473,11.0543020041665,0.255555991386337));
#95366=CARTESIAN_POINT('Ctrl Pts',(8.77696122488992,11.0562525456141,0.104286681754343));
#95367=CARTESIAN_POINT('Ctrl Pts',(8.76744115389902,11.059482082042,-0.146171849369996));
#95368=CARTESIAN_POINT('Ctrl Pts',(8.75799061301917,11.0539796414036,-0.396747075555581));
#95369=CARTESIAN_POINT('Ctrl Pts',(8.74857110277678,11.0399950780339,-0.646838836509623));
#95370=CARTESIAN_POINT('Ctrl Pts',(8.7433043604888,11.0321758720048,-0.786672948835796));
#95371=CARTESIAN_POINT('Ctrl Pts',(8.73804724784972,11.0217048656153,-0.926356853973552));
#95372=CARTESIAN_POINT('Ctrl Pts',(8.73279264605785,11.0086247373998,-1.06579266178105));
#95373=CARTESIAN_POINT('Ctrl Pts',(8.72130194515204,10.9800212680816,-1.37070923330026));
#95374=CARTESIAN_POINT('Ctrl Pts',(8.709811581266,10.938995324277,-1.67444970805189));
#95375=CARTESIAN_POINT('Ctrl Pts',(8.69834247180759,10.8855161855157,-1.97602583502142));
#95376=CARTESIAN_POINT('Ctrl Pts',(8.69518671476814,10.870801253269,-2.05900533653078));
#95377=CARTESIAN_POINT('Ctrl Pts',(8.692032574245,10.8551433260322,-2.14182072967303));
#95378=CARTESIAN_POINT('Ctrl Pts',(8.6888805008341,10.8385413880217,-2.22445084384318));
#95379=CARTESIAN_POINT('Ctrl Pts',(8.67427062587417,10.7615913279162,-2.60744180838551));
#95380=CARTESIAN_POINT('Ctrl Pts',(8.65963925766812,10.6645750156873,-2.98669631489204));
#95381=CARTESIAN_POINT('Ctrl Pts',(8.64498787790579,10.5476602194324,-3.35982430183711));
#95382=CARTESIAN_POINT('Ctrl Pts',(8.63033649814347,10.4307454231775,-3.73295228878218));
#95383=CARTESIAN_POINT('Ctrl Pts',(8.6156651102302,10.2939323547083,-4.09995268161777));
#95384=CARTESIAN_POINT('Ctrl Pts',(8.60097492287562,10.1374461559647,-4.45844717160862));
#95385=CARTESIAN_POINT('Ctrl Pts',(8.58628891771984,9.98100450780262,-4.81683960059872));
#95386=CARTESIAN_POINT('Ctrl Pts',(8.57158412839069,9.80490129183946,-5.16672999235309));
#95387=CARTESIAN_POINT('Ctrl Pts',(8.55686143044795,9.61070036994355,-5.50636554871548));
#95388=CARTESIAN_POINT('Ctrl Pts',(8.54213873250521,9.41649944804763,-5.84600110507788));
#95389=CARTESIAN_POINT('Ctrl Pts',(8.52739813169481,9.20420164947267,-6.17538109796706));
#95390=CARTESIAN_POINT('Ctrl Pts',(8.51264009359485,8.9754144165332,-6.49279241538405));
#95391=CARTESIAN_POINT('Ctrl Pts',(8.497227712024,8.73648319080253,-6.82427714972365));
#95392=CARTESIAN_POINT('Ctrl Pts',(8.48185121176318,8.47927918088958,-7.1426891506523));
#95393=CARTESIAN_POINT('Ctrl Pts',(8.46648978902769,8.20552414307779,-7.44626598819801));
#95394=CARTESIAN_POINT('Ctrl Pts',(8.45242853743153,7.95493938093226,-7.72414847115558));
#95395=CARTESIAN_POINT('Ctrl Pts',(8.43837988325975,7.69048611062595,-7.98960150491039));
#95396=CARTESIAN_POINT('Ctrl Pts',(8.42432677244307,7.41344658696125,-8.2412742508201));
#95397=CARTESIAN_POINT('Ctrl Pts',(8.40962405987569,7.12360097630753,-8.50458051036805));
#95398=CARTESIAN_POINT('Ctrl Pts',(8.39491626642312,6.81997188474144,-8.75280416621937));
#95399=CARTESIAN_POINT('Ctrl Pts',(8.38023523264272,6.50398366978781,-8.98416903734638));
#95400=CARTESIAN_POINT('Ctrl Pts',(8.36555419886231,6.18799545483416,-9.2155339084734));
#95401=CARTESIAN_POINT('Ctrl Pts',(8.35089999149063,5.85964777077985,-9.43003908131022));
#95402=CARTESIAN_POINT('Ctrl Pts',(8.33630581874266,5.52041797009034,-9.62588983413724));
#95403=CARTESIAN_POINT('Ctrl Pts',(8.33630560542693,5.52041301173797,-9.62589269678976));
#95404=CARTESIAN_POINT('Ctrl Pts',(8.33630539211122,5.5204080533833,-9.62589555943828));
#95405=CARTESIAN_POINT('Ctrl Pts',(8.33630517879552,5.52040309502629,-9.62589842208283));
#95406=CARTESIAN_POINT('Ctrl Pts',(8.32139797797909,5.17389684229249,-9.82594941329877));
#95407=CARTESIAN_POINT('Ctrl Pts',(8.30650499563908,4.81613020648062,-10.0067024134377));
#95408=CARTESIAN_POINT('Ctrl Pts',(8.29159566636577,4.44948056334772,-10.1676188745158));
#95409=CARTESIAN_POINT('Ctrl Pts',(8.27672502322162,4.08378228799208,-10.3281177960196));
#95410=CARTESIAN_POINT('Ctrl Pts',(8.26183814788653,3.7092474760114,-10.4688838498593));
#95411=CARTESIAN_POINT('Ctrl Pts',(8.24690344554343,3.32818901516837,-10.5894060653215));
#95412=CARTESIAN_POINT('Ctrl Pts',(8.23284526090791,2.96949487608279,-10.7028548317398));
#95413=CARTESIAN_POINT('Ctrl Pts',(8.21874475651843,2.60502013603582,-10.7983670812942));
#95414=CARTESIAN_POINT('Ctrl Pts',(8.20457381338371,2.23665246595822,-10.87552500873));
#95415=CARTESIAN_POINT('Ctrl Pts',(8.20456244779311,2.23635702224024,-10.8755868920787));
#95416=CARTESIAN_POINT('Ctrl Pts',(8.20455108215707,2.23606157601586,-10.8756487636208));
#95417=CARTESIAN_POINT('Ctrl Pts',(8.20453971647558,2.23576612728608,-10.8757106233563));
#95418=CARTESIAN_POINT('Ctrl Pts',(8.19131068089454,1.89187986228734,-10.9477119936699));
#95419=CARTESIAN_POINT('Ctrl Pts',(8.17802314470091,1.54465766477505,-11.0037037525121));
#95420=CARTESIAN_POINT('Ctrl Pts',(8.16471225861559,1.19560697869185,-11.0433202676434));
#95421=CARTESIAN_POINT('Ctrl Pts',(8.1513852003287,0.846132209792844,-11.0829849152779));
#95422=CARTESIAN_POINT('Ctrl Pts',(8.13803468467661,0.494824289630856,-11.1062336694404));
#95423=CARTESIAN_POINT('Ctrl Pts',(8.12469866360721,0.14324613009726,-11.1126845249433));
#95424=CARTESIAN_POINT('Ctrl Pts',(8.11137603138464,-0.207979058628419,
-11.1191289040381));
#95425=CARTESIAN_POINT('Ctrl Pts',(8.09806790537919,-0.559473985274116,
-11.108808265246));
#95426=CARTESIAN_POINT('Ctrl Pts',(8.08481486157169,-0.909628717147954,
-11.0813392565442));
#95427=CARTESIAN_POINT('Ctrl Pts',(8.08018383993,-1.03198356368732,-11.0717407389793));
#95428=CARTESIAN_POINT('Ctrl Pts',(8.07555956469545,-1.15417430605097,-11.0600484092193));
#95429=CARTESIAN_POINT('Ctrl Pts',(8.07094382065994,-1.2761307670632,-11.0462461270049));
#95430=CARTESIAN_POINT('Ctrl Pts',(8.07094256944499,-1.27616382646709,-11.0462423855449));
#95431=CARTESIAN_POINT('Ctrl Pts',(8.07094131823068,-1.27619688585376,-11.0462386439298));
#95432=CARTESIAN_POINT('Ctrl Pts',(8.07094006701699,-1.27622994522321,-11.0462349021597));
#95433=CARTESIAN_POINT('Ctrl Pts',(8.04671457520307,-1.91631204428851,-10.9737882675603));
#95434=CARTESIAN_POINT('Ctrl Pts',(8.02248078127624,-2.55028638804477,-10.8440120921138));
#95435=CARTESIAN_POINT('Ctrl Pts',(7.99824053625373,-3.16902712658607,-10.6607906274779));
#95436=CARTESIAN_POINT('Ctrl Pts',(7.973109117478,-3.81051538709868,-10.4708331682116));
#95437=CARTESIAN_POINT('Ctrl Pts',(7.94797076485528,-4.43562813347157,-10.2234287113763));
#95438=CARTESIAN_POINT('Ctrl Pts',(7.92282746351364,-5.03418592806953,-9.92296298718306));
#95439=CARTESIAN_POINT('Ctrl Pts',(7.89720134970723,-5.64423748636169,-9.61672759118328));
#95440=CARTESIAN_POINT('Ctrl Pts',(7.87157009539991,-6.22670301212677,-9.25537407620778));
#95441=CARTESIAN_POINT('Ctrl Pts',(7.84593572027054,-6.77081614111878,-8.8435975657615));
#95442=CARTESIAN_POINT('Ctrl Pts',(7.83235257565593,-7.0591308466853,-8.62540539754739));
#95443=CARTESIAN_POINT('Ctrl Pts',(7.81876855342073,-7.33667755373648,-8.39305663640217));
#95444=CARTESIAN_POINT('Ctrl Pts',(7.80518394485515,-7.60185783775227,-8.14725473688907));
#95445=CARTESIAN_POINT('Ctrl Pts',(7.80517720761467,-7.60198935301348,-8.14713283227184));
#95446=CARTESIAN_POINT('Ctrl Pts',(7.80517047037404,-7.60212086523309,-8.14701092434567));
#95447=CARTESIAN_POINT('Ctrl Pts',(7.80516373313327,-7.60225237441096,-8.14688901311081));
#95448=CARTESIAN_POINT('Ctrl Pts',(7.78072942945136,-8.07920359217663,-7.70474715751269));
#95449=CARTESIAN_POINT('Ctrl Pts',(7.75628358169676,-8.51608048184164,-7.21921732485523));
#95450=CARTESIAN_POINT('Ctrl Pts',(7.73182870837808,-8.90798904969996,-6.6991970798396));
#95451=CARTESIAN_POINT('Ctrl Pts',(7.7065854677389,-9.31253182357114,-6.16241261111158));
#95452=CARTESIAN_POINT('Ctrl Pts',(7.68133260625059,-9.66916085721407,-5.58887669198447));
#95453=CARTESIAN_POINT('Ctrl Pts',(7.65607339934336,-9.97245221159837,-4.98833609696704));
#95454=CARTESIAN_POINT('Ctrl Pts',(7.63088020110482,-10.2749509892956,-4.38936486575889));
#95455=CARTESIAN_POINT('Ctrl Pts',(7.60568069097792,-10.5243908685266,-3.76352836231937));
#95456=CARTESIAN_POINT('Ctrl Pts',(7.58047863651457,-10.7153424597389,-3.12048150287961));
#95457=CARTESIAN_POINT('Ctrl Pts',(7.56662102963664,-10.8203391411636,-2.76689562379342));
#95458=CARTESIAN_POINT('Ctrl Pts',(7.55276266260403,-10.9076512315918,-2.40810612198082));
#95459=CARTESIAN_POINT('Ctrl Pts',(7.53890422701102,-10.9763693314388,-2.045718580393));
#95460=CARTESIAN_POINT('Ctrl Pts',(7.53889927044658,-10.976393908938,-2.04558897000591));
#95461=CARTESIAN_POINT('Ctrl Pts',(7.53889431388162,-10.9764184840602,-2.0454593591586));
#95462=CARTESIAN_POINT('Ctrl Pts',(7.53888935731614,-10.9764430568053,-2.04532974785116));
#95463=CARTESIAN_POINT('Ctrl Pts',(7.50995500813713,-11.1198884303692,-1.28871332803983));
#95464=CARTESIAN_POINT('Ctrl Pts',(7.481002919287,-11.1823251731434,-0.516413750306353));
#95465=CARTESIAN_POINT('Ctrl Pts',(7.4520371360579,-11.1657699667983,0.254856495553427));
#95466=CARTESIAN_POINT('Ctrl Pts',(7.42206844780455,-11.1486415565634,1.05283103587334));
#95467=CARTESIAN_POINT('Ctrl Pts',(7.39208509902904,-11.0469562263886,1.84970208167534));
#95468=CARTESIAN_POINT('Ctrl Pts',(7.36209180085476,-10.8629991228641,2.62693895094568));
#95469=CARTESIAN_POINT('Ctrl Pts',(7.33209850268048,-10.6790420193395,3.40417582021604));
#95470=CARTESIAN_POINT('Ctrl Pts',(7.3020952552254,-10.4128131726403,4.16177655833391));
#95471=CARTESIAN_POINT('Ctrl Pts',(7.27208700464185,-10.0666499299777,4.8812170112621));
#95472=CARTESIAN_POINT('Ctrl Pts',(7.27208662092667,-10.066645503592,4.88122621073938));
#95473=CARTESIAN_POINT('Ctrl Pts',(7.2720862372115,-10.0666410771933,4.88123541021042));
#95474=CARTESIAN_POINT('Ctrl Pts',(7.27208585349632,-10.0666366507816,4.88124460967523));
#95475=CARTESIAN_POINT('Ctrl Pts',(7.23228903670486,-9.6075536928767,5.83536224009391));
#95476=CARTESIAN_POINT('Ctrl Pts',(7.19248043715747,-9.00787535320312,6.7224152676858));
#95477=CARTESIAN_POINT('Ctrl Pts',(7.15265826104708,-8.29767799140454,7.51084519278056));
#95478=CARTESIAN_POINT('Ctrl Pts',(7.11184999850807,-7.5698945494739,8.31879841180325));
#95479=CARTESIAN_POINT('Ctrl Pts',(7.0710274788903,-6.72604943649446,9.0231857719293));
#95480=CARTESIAN_POINT('Ctrl Pts',(7.03018869589303,-5.79846489065266,9.59002045639908));
#95481=CARTESIAN_POINT('Ctrl Pts',(7.02173023308444,-5.60634507691215,9.70742234120858));
#95482=CARTESIAN_POINT('Ctrl Pts',(7.01327107234976,-5.41063290456088,9.81892334267702));
#95483=CARTESIAN_POINT('Ctrl Pts',(7.00481119545851,-5.21161542129423,9.92422123240472));
#95484=CARTESIAN_POINT('Ctrl Pts',(7.00481117113412,-5.21161484906612,9.92422153516411));
#95485=CARTESIAN_POINT('Ctrl Pts',(7.00481114680973,-5.21161427683798,9.92422183792345));
#95486=CARTESIAN_POINT('Ctrl Pts',(7.00481112248533,-5.21161370460982,9.92422214068274));
#95487=CARTESIAN_POINT('Ctrl Pts',(6.95949580048587,-4.14557665577187,10.4882499890114));
#95488=CARTESIAN_POINT('Ctrl Pts',(6.91413937966825,-2.98477603349806,10.8743265992955));
#95489=CARTESIAN_POINT('Ctrl Pts',(6.86875514637579,-1.79216017556988,11.0712521117833));
#95490=CARTESIAN_POINT('Ctrl Pts',(6.82484072307876,-0.638168275380296,
11.2618000110427));
#95491=CARTESIAN_POINT('Ctrl Pts',(6.78090026783952,0.54561229331462,11.275247854403));
#95492=CARTESIAN_POINT('Ctrl Pts',(6.73694742131768,1.70211153428016,11.1014270624495));
#95493=CARTESIAN_POINT('Ctrl Pts',(6.73694635133782,1.70213968788115,11.1014228309887));
#95494=CARTESIAN_POINT('Ctrl Pts',(6.73694528135794,1.70216784146597,11.1014185994169));
#95495=CARTESIAN_POINT('Ctrl Pts',(6.73694421137806,1.70219599503462,11.1014143677342));
#95496=CARTESIAN_POINT('Ctrl Pts',(6.69068820405194,2.91929521429124,10.9184756481802));
#95497=CARTESIAN_POINT('Ctrl Pts',(6.64441099772795,4.10619837218388,10.5281362965954));
#95498=CARTESIAN_POINT('Ctrl Pts',(6.59811266643679,5.20164540543921,9.96066846821707));
#95499=CARTESIAN_POINT('Ctrl Pts',(6.55495578108234,6.22276389303163,9.4317046086418));
#95500=CARTESIAN_POINT('Ctrl Pts',(6.51178053818585,7.1644145500614,8.74883553718005));
#95501=CARTESIAN_POINT('Ctrl Pts',(6.46858684323349,7.97700317709334,7.93661371656795));
#95502=CARTESIAN_POINT('Ctrl Pts',(6.46858241565496,7.97708647165656,7.93653045960431));
#95503=CARTESIAN_POINT('Ctrl Pts',(6.46857798807624,7.97716976486372,7.93644720128152));
#95504=CARTESIAN_POINT('Ctrl Pts',(6.46857356049733,7.97725305671478,7.93636394159967));
#95505=CARTESIAN_POINT('Ctrl Pts',(6.41597493735464,8.96674116546658,6.94725799566618));
#95506=CARTESIAN_POINT('Ctrl Pts',(6.36334786988935,9.76486922000591,5.76632989175888));
#95507=CARTESIAN_POINT('Ctrl Pts',(6.3106911995868,10.3278483444582,4.48170981970171));
#95508=CARTESIAN_POINT('Ctrl Pts',(6.27371870834979,10.7231399689729,3.57972334611484));
#95509=CARTESIAN_POINT('Ctrl Pts',(6.23673162266534,11.0025015723476,2.62661508981526));
#95510=CARTESIAN_POINT('Ctrl Pts',(6.19972953977931,11.1507603510177,1.65288782707181));
#95511=CARTESIAN_POINT('Ctrl Pts',(6.18620303910717,11.204957907288,1.29693158226929));
#95512=CARTESIAN_POINT('Ctrl Pts',(6.17267489270487,11.2416340018188,0.938229413935324));
#95513=CARTESIAN_POINT('Ctrl Pts',(6.15914510492325,11.2609492036324,0.578477224997408));
#95514=CARTESIAN_POINT('Ctrl Pts',(6.11285293765214,11.3270361643196,-0.652414846280726));
#95515=CARTESIAN_POINT('Ctrl Pts',(6.0665415518186,11.1898853054317,-1.89559503509316));
#95516=CARTESIAN_POINT('Ctrl Pts',(6.02021108604259,10.8559260765016,-3.08317147400487));
#95517=CARTESIAN_POINT('Ctrl Pts',(6.02020856522246,10.8559079059278,-3.08323608951306));
#95518=CARTESIAN_POINT('Ctrl Pts',(6.02020604440228,10.8558897347714,-3.08330070485664));
#95519=CARTESIAN_POINT('Ctrl Pts',(6.02020352358204,10.8558715630324,-3.08336532003562));
#95520=CARTESIAN_POINT('Ctrl Pts',(5.98978091762796,10.636565304282,-3.86317583451194));
#95521=CARTESIAN_POINT('Ctrl Pts',(5.95939936030158,10.332268746888,-4.61907445363975));
#95522=CARTESIAN_POINT('Ctrl Pts',(5.92902341902273,9.95150322999734,-5.33455706247603));
#95523=CARTESIAN_POINT('Ctrl Pts',(5.8996254815835,9.58299709081924,-6.02700352134749));
#95524=CARTESIAN_POINT('Ctrl Pts',(5.87023278073892,9.14286870013787,-6.68159552966999));
#95525=CARTESIAN_POINT('Ctrl Pts',(5.84081112680754,8.63883207786456,-7.28341797140726));
#95526=CARTESIAN_POINT('Ctrl Pts',(5.84080847416191,8.63878663410579,-7.28347223149999));
#95527=CARTESIAN_POINT('Ctrl Pts',(5.84080582151604,8.6387411898275,-7.2835264911638));
#95528=CARTESIAN_POINT('Ctrl Pts',(5.84080316886994,8.63869574502971,-7.28358075039867));
#95529=CARTESIAN_POINT('Ctrl Pts',(5.81466418682828,8.19088600845037,-7.81824730980955));
#95530=CARTESIAN_POINT('Ctrl Pts',(5.78845545804168,7.69275291643841,-8.31127372036197));
#95531=CARTESIAN_POINT('Ctrl Pts',(5.76221253802134,7.15365412876904,-8.75474726498968));
#95532=CARTESIAN_POINT('Ctrl Pts',(5.7356328223173,6.60763666952502,-9.20391224851042));
#95533=CARTESIAN_POINT('Ctrl Pts',(5.70901800908207,6.01959384493397,-9.60224326500889));
#95534=CARTESIAN_POINT('Ctrl Pts',(5.68240714568773,5.39927719035735,-9.94147517498252));
#95535=CARTESIAN_POINT('Ctrl Pts',(5.67516337950511,5.23042025631692,-10.0338177871375));
#95536=CARTESIAN_POINT('Ctrl Pts',(5.66791991878384,5.05917210024071,-10.1217810351109));
#95537=CARTESIAN_POINT('Ctrl Pts',(5.66067757974053,4.8857299708475,-10.2051978341173));
#95538=CARTESIAN_POINT('Ctrl Pts',(5.66067284953871,4.88561669028005,-10.2052523162801));
#95539=CARTESIAN_POINT('Ctrl Pts',(5.66066811933736,4.88550340877672,-10.2053067965034));
#95540=CARTESIAN_POINT('Ctrl Pts',(5.6606633891365,4.88539012633754,-10.2053612747873));
#95541=CARTESIAN_POINT('Ctrl Pts',(5.62118471048364,3.93992477681437,-10.6600418952297));
#95542=CARTESIAN_POINT('Ctrl Pts',(5.58172432895299,2.92921033768375,-10.9796773858916));
#95543=CARTESIAN_POINT('Ctrl Pts',(5.54226356021694,1.89377849318269,-11.1580953544777));
#95544=CARTESIAN_POINT('Ctrl Pts',(5.50157002294364,0.825999387306831,-11.3420871642534));
#95545=CARTESIAN_POINT('Ctrl Pts',(5.46087607647536,-0.26806365938397,-11.3759020335183));
#95546=CARTESIAN_POINT('Ctrl Pts',(5.42015933791027,-1.34399290354479,-11.2528125098426));
#95547=CARTESIAN_POINT('Ctrl Pts',(5.41017075462064,-1.6079386233591,-11.2226163300245));
#95548=CARTESIAN_POINT('Ctrl Pts',(5.40018079084945,-1.87079324599402,-11.1829775503671));
#95549=CARTESIAN_POINT('Ctrl Pts',(5.39018909898668,-2.13190145643179,-11.1337970135774));
#95550=CARTESIAN_POINT('Ctrl Pts',(5.39018544367648,-2.13199697894367,-11.1337790216176));
#95551=CARTESIAN_POINT('Ctrl Pts',(5.39018178836605,-2.13209250122182,-11.1337610283809));
#95552=CARTESIAN_POINT('Ctrl Pts',(5.39017813305539,-2.1321880232662,-11.1337430338671));
#95553=CARTESIAN_POINT('Ctrl Pts',(5.34005511352045,-3.44202287456579,-10.8869953703623));
#95554=CARTESIAN_POINT('Ctrl Pts',(5.28991456891932,-4.70786373365093,-10.4001007459573));
#95555=CARTESIAN_POINT('Ctrl Pts',(5.23975236461588,-5.85487486493485,-9.71395761238606));
#95556=CARTESIAN_POINT('Ctrl Pts',(5.19962465794871,-6.77243673964246,-9.16507123911028));
#95557=CARTESIAN_POINT('Ctrl Pts',(5.15948308710158,-7.61395644577873,-8.48867732473233));
#95558=CARTESIAN_POINT('Ctrl Pts',(5.11932545839374,-8.3411162598051,-7.70569001257604));
#95559=CARTESIAN_POINT('Ctrl Pts',(5.11932451336444,-8.34113337205387,-7.70567158653899));
#95560=CARTESIAN_POINT('Ctrl Pts',(5.11932356833513,-8.34115048423931,-7.70565316044291));
#95561=CARTESIAN_POINT('Ctrl Pts',(5.1193226233058,-8.34116759636142,-7.7056347342878));
#95562=CARTESIAN_POINT('Ctrl Pts',(5.06030728534759,-9.40978805765443,-6.55495533566297));
#95563=CARTESIAN_POINT('Ctrl Pts',(5.00125411221408,-10.2314223980218,-5.17406477254987));
#95564=CARTESIAN_POINT('Ctrl Pts',(4.94216997403342,-10.7485626406966,-3.68783542484532));
#95565=CARTESIAN_POINT('Ctrl Pts',(4.91079087924851,-11.0232115260263,-2.89851136918884));
#95566=CARTESIAN_POINT('Ctrl Pts',(4.87940305062228,-11.2119758229205,-2.0794765216812));
#95567=CARTESIAN_POINT('Ctrl Pts',(4.84800751790959,-11.3062457605422,-1.24943989390665));
#95568=CARTESIAN_POINT('Ctrl Pts',(4.84800722672529,-11.306246634868,-1.24943219556201));
#95569=CARTESIAN_POINT('Ctrl Pts',(4.84800693554099,-11.3062475091857,-1.24942449721643));
#95570=CARTESIAN_POINT('Ctrl Pts',(4.8480066443567,-11.3062483834953,-1.2494167988699));
#95571=CARTESIAN_POINT('Ctrl Pts',(4.75749576470224,-11.5780162292644,1.14351483703349));
#95572=CARTESIAN_POINT('Ctrl Pts',(4.66692016212201,-11.0644284693562,3.62790218399632));
#95573=CARTESIAN_POINT('Ctrl Pts',(4.57624214332606,-9.85962740447419,5.71840762354233));
#95574=CARTESIAN_POINT('Ctrl Pts',(4.57624210922295,-9.85962695136046,5.71840840976068));
#95575=CARTESIAN_POINT('Ctrl Pts',(4.57624207511985,-9.85962649824664,5.71840919597897));
#95576=CARTESIAN_POINT('Ctrl Pts',(4.57624204101675,-9.85962604513272,5.71840998219722));
#95577=CARTESIAN_POINT('Ctrl Pts',(4.48556405918101,-8.65482495242934,7.80891427160857));
#95578=CARTESIAN_POINT('Ctrl Pts',(4.39477592636952,-6.75882245833947,9.50552941330722));
#95579=CARTESIAN_POINT('Ctrl Pts',(4.30397532251536,-4.54410559013394,10.4724028831779));
#95580=CARTESIAN_POINT('Ctrl Pts',(4.30397525127883,-4.54410385260408,10.472403641727));
#95581=CARTESIAN_POINT('Ctrl Pts',(4.30397518004229,-4.54410211507402,10.4724044002757));
#95582=CARTESIAN_POINT('Ctrl Pts',(4.30397510880575,-4.54410037754377,10.4724051588239));
#95583=CARTESIAN_POINT('Ctrl Pts',(4.21317449695879,-2.32938281477614,11.4392775685767));
#95584=CARTESIAN_POINT('Ctrl Pts',(4.12236011008899,0.204050645536416,11.6764109304539));
#95585=CARTESIAN_POINT('Ctrl Pts',(4.03129677776446,2.56543232038823,11.1417036427205));
#95586=CARTESIAN_POINT('Ctrl Pts',(4.03129671431827,2.56543396562396,11.1417032701761));
#95587=CARTESIAN_POINT('Ctrl Pts',(4.03129665087209,2.56543561085961,11.1417028976313));
#95588=CARTESIAN_POINT('Ctrl Pts',(4.03129658742591,2.56543725609518,11.1417025250862));
#95589=CARTESIAN_POINT('Ctrl Pts',(3.96299908741186,4.33647334566173,10.7406712496474));
#95590=CARTESIAN_POINT('Ctrl Pts',(3.89456170172107,6.01072971361824,9.90548016627018));
#95591=CARTESIAN_POINT('Ctrl Pts',(3.82642688347337,7.40108554833901,8.73184202297608));
#95592=CARTESIAN_POINT('Ctrl Pts',(3.82642683651131,7.4010865066444,8.73184121404377));
#95593=CARTESIAN_POINT('Ctrl Pts',(3.82642678954926,7.40108746494964,8.73184040511131));
#95594=CARTESIAN_POINT('Ctrl Pts',(3.82642674258721,7.40108842325476,8.73183959617868));
#95595=CARTESIAN_POINT('Ctrl Pts',(3.75829190713916,8.79144422611794,7.55820068286923));
#95596=CARTESIAN_POINT('Ctrl Pts',(3.6904595686611,9.89789927334666,6.04611449400784));
#95597=CARTESIAN_POINT('Ctrl Pts',(3.6207940229697,10.5960088267933,4.36539634576722));
#95598=CARTESIAN_POINT('Ctrl Pts',(3.62079399296584,10.5960091274581,4.36539562190821));
#95599=CARTESIAN_POINT('Ctrl Pts',(3.62079396296198,10.5960094281229,4.36539489804917));
#95600=CARTESIAN_POINT('Ctrl Pts',(3.62079393295812,10.5960097287876,4.36539417419011));
#95601=CARTESIAN_POINT('Ctrl Pts',(3.55112837455883,11.2941190420186,2.68467561220641));
#95602=CARTESIAN_POINT('Ctrl Pts',(3.47962957405442,11.5838826054181,0.835325224206452));
#95603=CARTESIAN_POINT('Ctrl Pts',(3.42175958283319,11.4318218501684,-0.979655960985377));
#95604=CARTESIAN_POINT('Ctrl Pts',(3.42175956715402,11.4318218089694,-0.979656452732337));
#95605=CARTESIAN_POINT('Ctrl Pts',(3.42175955147486,11.4318217677704,-0.979656944479301));
#95606=CARTESIAN_POINT('Ctrl Pts',(3.42175953579569,11.4318217265713,-0.979657436226255));
#95607=CARTESIAN_POINT('Ctrl Pts',(3.3638895362804,11.2797606907088,-2.79463909454147));
#95608=CARTESIAN_POINT('Ctrl Pts',(3.31964848099095,10.6858751883979,-4.57525165075327));
#95609=CARTESIAN_POINT('Ctrl Pts',(3.26934389910569,9.71592393542433,-6.12115521092141));
#95610=CARTESIAN_POINT('Ctrl Pts',(3.21903931722043,8.74597268245079,-7.66705877108943));
#95611=CARTESIAN_POINT('Ctrl Pts',(3.16267108324328,7.39995562580389,-8.97825315031857));
#95612=CARTESIAN_POINT('Ctrl Pts',(3.1092085985088,5.8273121468005,-9.90727266988443));
#95613=CARTESIAN_POINT('Ctrl Pts',(3.05574611377432,4.25466866779709,-10.8362921894503));
#95614=CARTESIAN_POINT('Ctrl Pts',(3.00518947058605,2.45539879241857,-11.3831369591947));
#95615=CARTESIAN_POINT('Ctrl Pts',(2.95317599819347,0.630199733268789,-11.4865686023698));
#95616=CARTESIAN_POINT('Ctrl Pts',(2.90116252580088,-1.19499932588101,-11.5900002455448));
#95617=CARTESIAN_POINT('Ctrl Pts',(2.84769218566752,-3.04612758015582,-11.2500187197434));
#95618=CARTESIAN_POINT('Ctrl Pts',(2.79488159658331,-4.71660844897229,-10.5035064391955));
#95619=CARTESIAN_POINT('Ctrl Pts',(2.7420710074991,-6.38708931778873,-9.75699415864752));
#95620=CARTESIAN_POINT('Ctrl Pts',(2.68992015353981,-7.87692275998864,-8.60395112887428));
#95621=CARTESIAN_POINT('Ctrl Pts',(2.63743468235449,-9.01931348046436,-7.17271637140658));
#95622=CARTESIAN_POINT('Ctrl Pts',(2.63743467004437,-9.0193137484046,-7.17271603571986));
#95623=CARTESIAN_POINT('Ctrl Pts',(2.63743465773425,-9.01931401634483,-7.17271570003313));
#95624=CARTESIAN_POINT('Ctrl Pts',(2.63743464542413,-9.01931428428504,-7.17271536434638));
#95625=CARTESIAN_POINT('Ctrl Pts',(2.58494918639199,-10.1617045738397,-5.74148081206935));
#95626=CARTESIAN_POINT('Ctrl Pts',(2.53212914832179,-10.9566523403097,-4.03205471200254));
#95627=CARTESIAN_POINT('Ctrl Pts',(2.47942578441284,-11.3149095833295,-2.2345112037788));
#95628=CARTESIAN_POINT('Ctrl Pts',(2.47942576112028,-11.3149097416634,-2.23451040934395));
#95629=CARTESIAN_POINT('Ctrl Pts',(2.47942573782772,-11.3149098999972,-2.23450961490907));
#95630=CARTESIAN_POINT('Ctrl Pts',(2.47942571453516,-11.3149100583309,-2.23450882047418));
#95631=CARTESIAN_POINT('Ctrl Pts',(2.42672236166057,-11.673166841048,-0.436965607195262));
#95632=CARTESIAN_POINT('Ctrl Pts',(2.37413557642947,-11.594733173071,1.44869484258399));
#95633=CARTESIAN_POINT('Ctrl Pts',(2.32146716899691,-11.0874541804838,3.21132484352732));
#95634=CARTESIAN_POINT('Ctrl Pts',(2.32146714047697,-11.0874539057922,3.21132579799139));
#95635=CARTESIAN_POINT('Ctrl Pts',(2.32146711195703,-11.0874536311005,3.21132675245542));
#95636=CARTESIAN_POINT('Ctrl Pts',(2.32146708343709,-11.0874533564087,3.21132770691942));
#95637=CARTESIAN_POINT('Ctrl Pts',(2.26879868115906,-10.5801739498787,4.97395739916155));
#95638=CARTESIAN_POINT('Ctrl Pts',(2.21604875089909,-9.64404943021566,6.61355667467342));
#95639=CARTESIAN_POINT('Ctrl Pts',(2.16330110871024,-8.38328705927666,7.94836318859917));
#95640=CARTESIAN_POINT('Ctrl Pts',(2.1633010790123,-8.38328634944304,7.94836394012108));
#95641=CARTESIAN_POINT('Ctrl Pts',(2.16330104931436,-8.38328563960932,7.94836469164289));
#95642=CARTESIAN_POINT('Ctrl Pts',(2.16330101961641,-8.38328492977549,7.9483654431646));
#95643=CARTESIAN_POINT('Ctrl Pts',(2.1105533785651,-7.12252222041275,9.28317158515742));
#95644=CARTESIAN_POINT('Ctrl Pts',(2.05780789908406,-5.53712179696833,10.3131846727588));
#95645=CARTESIAN_POINT('Ctrl Pts',(2.00503741874543,-3.8029092346673,10.9196062470078));
#95646=CARTESIAN_POINT('Ctrl Pts',(1.9522669689543,-2.06869767625853,11.5260274702144));
#95647=CARTESIAN_POINT('Ctrl Pts',(1.89947155499029,-0.185674043531211,
11.7088577069818));
#95648=CARTESIAN_POINT('Ctrl Pts',(1.84664003082162,1.63475428012898,11.4539068979886));
#95649=CARTESIAN_POINT('Ctrl Pts',(1.84663997049356,1.634756358867,11.4539066068616));
#95650=CARTESIAN_POINT('Ctrl Pts',(1.84663991016551,1.63475843760494,11.4539063157339));
#95651=CARTESIAN_POINT('Ctrl Pts',(1.84663984983746,1.6347605163428,11.4539060246057));
#95652=CARTESIAN_POINT('Ctrl Pts',(1.79380839845376,3.45518618623734,11.1989545674529));
#95653=CARTESIAN_POINT('Ctrl Pts',(1.74094090272129,5.21301617918042,10.5062232930386));
#95654=CARTESIAN_POINT('Ctrl Pts',(1.68809114646529,6.71448492712146,9.43804832595781));
#95655=CARTESIAN_POINT('Ctrl Pts',(1.68809101322363,6.71448871253515,9.43804563293862));
#95656=CARTESIAN_POINT('Ctrl Pts',(1.68809087998197,6.71449249794722,9.43804293991704));
#95657=CARTESIAN_POINT('Ctrl Pts',(1.68809074674031,6.71449628335766,9.43804024689308));
#95658=CARTESIAN_POINT('Ctrl Pts',(1.63524099091071,8.21596372907952,8.36986339353148));
#95659=CARTESIAN_POINT('Ctrl Pts',(1.58240874757455,9.46106908054857,6.92624306034315));
#95660=CARTESIAN_POINT('Ctrl Pts',(1.52945999603721,10.3045992775066,5.30076081748356));
#95661=CARTESIAN_POINT('Ctrl Pts',(1.52945986220838,10.3046014095429,5.30075670905086));
#95662=CARTESIAN_POINT('Ctrl Pts',(1.52945972837956,10.3046035415765,5.30075260061701));
#95663=CARTESIAN_POINT('Ctrl Pts',(1.52945959455073,10.3046056736076,5.30074849218199));
#95664=CARTESIAN_POINT('Ctrl Pts',(1.47651070859563,11.1481359726256,3.67526122157152));
#95665=CARTESIAN_POINT('Ctrl Pts',(1.42344639163322,11.5900913133187,1.86791206070984));
#95666=CARTESIAN_POINT('Ctrl Pts',(1.37078399030106,11.5968559808931,-0.0151246218382906));
#95667=CARTESIAN_POINT('Ctrl Pts',(20.6563591733144,-11.5926712737699,-0.0152754849923014));
#95668=CARTESIAN_POINT('Ctrl Pts',(20.6037145486049,-11.585908889594,1.86712555758729));
#95669=CARTESIAN_POINT('Ctrl Pts',(20.5506704336544,-11.1441131812359,3.67379159074529));
#95670=CARTESIAN_POINT('Ctrl Pts',(20.4977411586544,-10.3008921028426,5.29867567785781));
#95671=CARTESIAN_POINT('Ctrl Pts',(20.4977410246894,-10.3008899686352,5.29867979046809));
#95672=CARTESIAN_POINT('Ctrl Pts',(20.4977408907245,-10.3008878344252,5.29868390307719));
#95673=CARTESIAN_POINT('Ctrl Pts',(20.4977407567596,-10.3008857002126,5.29868801568514));
#95674=CARTESIAN_POINT('Ctrl Pts',(20.4448116163112,-9.4576647239953,6.92356707000062));
#95675=CARTESIAN_POINT('Ctrl Pts',(20.3919983869448,-8.21301820129604,8.36666416537622));
#95676=CARTESIAN_POINT('Ctrl Pts',(20.3391682146961,-6.71210990886197,9.43444527360875));
#95677=CARTESIAN_POINT('Ctrl Pts',(20.33916808131,-6.71210611935304,9.43444796955364));
#95678=CARTESIAN_POINT('Ctrl Pts',(20.3391679479238,-6.7121023298424,9.4344506654962));
#95679=CARTESIAN_POINT('Ctrl Pts',(20.3391678145376,-6.7120985403302,9.4344533614363));
#95680=CARTESIAN_POINT('Ctrl Pts',(20.286337641874,-5.21118894454904,10.5022325811003));
#95681=CARTESIAN_POINT('Ctrl Pts',(20.2334903071855,-3.45401843924274,11.1946955874164));
#95682=CARTESIAN_POINT('Ctrl Pts',(20.1806788768804,-1.63428162441622,11.4495487431153));
#95683=CARTESIAN_POINT('Ctrl Pts',(20.1806788168593,-1.63427955625594,11.44954903276));
#95684=CARTESIAN_POINT('Ctrl Pts',(20.1806787568383,-1.63427748809554,11.4495493224042));
#95685=CARTESIAN_POINT('Ctrl Pts',(20.1806786968172,-1.6342754199351,11.4495496120478));
#95686=CARTESIAN_POINT('Ctrl Pts',(20.127867193276,0.185464063436388,11.7044021268553));
#95687=CARTESIAN_POINT('Ctrl Pts',(20.0750916629277,2.06776954364581,11.5216435485773));
#95688=CARTESIAN_POINT('Ctrl Pts',(20.0223414858343,3.80131493537512,10.9154560212435));
#95689=CARTESIAN_POINT('Ctrl Pts',(19.9695912794199,5.53486129069071,10.309268156962));
#95690=CARTESIAN_POINT('Ctrl Pts',(19.9168664069274,7.1196474471959,9.27965093289917));
#95691=CARTESIAN_POINT('Ctrl Pts',(19.8641392593043,8.37991863116215,7.94536453312017));
#95692=CARTESIAN_POINT('Ctrl Pts',(19.8641392286874,8.37991936295992,7.94536375834421));
#95693=CARTESIAN_POINT('Ctrl Pts',(19.8641391980705,8.37992009475757,7.94536298356816));
#95694=CARTESIAN_POINT('Ctrl Pts',(19.8641391674536,8.37992082655512,7.945362208792));
#95695=CARTESIAN_POINT('Ctrl Pts',(19.8114120255027,9.64019149801263,6.61107559879492));
#95696=CARTESIAN_POINT('Ctrl Pts',(19.7586826779208,10.5759470416542,4.9721199710173));
#95697=CARTESIAN_POINT('Ctrl Pts',(19.7060352623099,11.0830256424956,3.21018842377476));
#95698=CARTESIAN_POINT('Ctrl Pts',(19.7060352260731,11.0830259915146,3.2101872110484));
#95699=CARTESIAN_POINT('Ctrl Pts',(19.7060351898362,11.0830263405333,3.210185998322));
#95700=CARTESIAN_POINT('Ctrl Pts',(19.7060351535993,11.0830266895519,3.21018478559552));
#95701=CARTESIAN_POINT('Ctrl Pts',(19.6533877226761,11.5901048488513,1.44825255283667));
#95702=CARTESIAN_POINT('Ctrl Pts',(19.6008218004355,11.6685061651627,-0.436655556151005));
#95703=CARTESIAN_POINT('Ctrl Pts',(19.5481397518776,11.3103928857645,-2.2334789716602));
#95704=CARTESIAN_POINT('Ctrl Pts',(19.5481397310522,11.3103927442013,-2.23347968194976));
#95705=CARTESIAN_POINT('Ctrl Pts',(19.5481397102268,11.310392602638,-2.23348039223931));
#95706=CARTESIAN_POINT('Ctrl Pts',(19.5481396894015,11.3103924610746,-2.23348110252884));
#95707=CARTESIAN_POINT('Ctrl Pts',(19.4954576505601,10.9522789032391,-4.03030411386188));
#95708=CARTESIAN_POINT('Ctrl Pts',(19.4426589642928,10.1576489530311,-5.73904072781481));
#95709=CARTESIAN_POINT('Ctrl Pts',(19.3901948846326,9.01572496391351,-7.16969094962721));
#95710=CARTESIAN_POINT('Ctrl Pts',(19.3901948541255,9.01572429990197,-7.16969178152869));
#95711=CARTESIAN_POINT('Ctrl Pts',(19.3901948236184,9.01572363589031,-7.16969261343008));
#95712=CARTESIAN_POINT('Ctrl Pts',(19.3901947931114,9.01572297187853,-7.16969344533137));
#95713=CARTESIAN_POINT('Ctrl Pts',(19.3377306833332,7.87379791485763,-8.60034417564005));
#95714=CARTESIAN_POINT('Ctrl Pts',(19.2855977093484,6.3845758633306,-9.75290960514574));
#95715=CARTESIAN_POINT('Ctrl Pts',(19.2328105722069,4.71478199691756,-10.4991167385146));
#95716=CARTESIAN_POINT('Ctrl Pts',(19.2328105576676,4.71478153700262,-10.4991169440441));
#95717=CARTESIAN_POINT('Ctrl Pts',(19.2328105431283,4.71478107708768,-10.4991171495735));
#95718=CARTESIAN_POINT('Ctrl Pts',(19.232810528589,4.71478061717272,-10.4991173551029));
#95719=CARTESIAN_POINT('Ctrl Pts',(19.1800234056227,3.0449871112073,-11.2453240590873));
#95720=CARTESIAN_POINT('Ctrl Pts',(19.126575436485,1.19462796304064,-11.5851614135244));
#95721=CARTESIAN_POINT('Ctrl Pts',(19.0745838253278,-0.629806639099064,
-11.4817745800324));
#95722=CARTESIAN_POINT('Ctrl Pts',(19.0745837795721,-0.629808244709866,
-11.4817744890458));
#95723=CARTESIAN_POINT('Ctrl Pts',(19.0745837338164,-0.62980985032067,-11.4817743980589));
#95724=CARTESIAN_POINT('Ctrl Pts',(19.0745836880607,-0.629811455931433,
-11.4817743070717));
#95725=CARTESIAN_POINT('Ctrl Pts',(19.0353427236988,-2.00681388582104,-11.4037419135721));
#95726=CARTESIAN_POINT('Ctrl Pts',(18.9969205011456,-3.36905776993691,-11.0732077906153));
#95727=CARTESIAN_POINT('Ctrl Pts',(18.9574625391331,-4.63027157441452,-10.5165193993473));
#95728=CARTESIAN_POINT('Ctrl Pts',(18.9446414170003,-5.04007926335718,-10.3356339838239));
#95729=CARTESIAN_POINT('Ctrl Pts',(18.9317109342901,-5.43922050625814,-10.1308713769124));
#95730=CARTESIAN_POINT('Ctrl Pts',(18.9186074542421,-5.82473675705504,-9.9031359251377));
#95731=CARTESIAN_POINT('Ctrl Pts',(18.8866679432054,-6.76442609927844,-9.34803461245184));
#95732=CARTESIAN_POINT('Ctrl Pts',(18.8536879756499,-7.62314728010116,-8.65644218333828));
#95733=CARTESIAN_POINT('Ctrl Pts',(18.8215823250737,-8.36902821121461,-7.85982151710422));
#95734=CARTESIAN_POINT('Ctrl Pts',(18.7999795800723,-8.87090483626633,-7.32380393743614));
#95735=CARTESIAN_POINT('Ctrl Pts',(18.7787726604597,-9.32169308761486,-6.7402340793714));
#95736=CARTESIAN_POINT('Ctrl Pts',(18.7585450056109,-9.71167301288714,-6.11868848475595));
#95737=CARTESIAN_POINT('Ctrl Pts',(18.7585444020376,-9.71168464950343,-6.11866993844851));
#95738=CARTESIAN_POINT('Ctrl Pts',(18.7585437984652,-9.71169628606556,-6.11865139210728));
#95739=CARTESIAN_POINT('Ctrl Pts',(18.7585431948937,-9.71170792257357,-6.1186328457322));
#95740=CARTESIAN_POINT('Ctrl Pts',(18.7348347109139,-10.1687937088616,-5.39012525343856));
#95741=CARTESIAN_POINT('Ctrl Pts',(18.7124730873212,-10.5423427757897,-4.60943846859312));
#95742=CARTESIAN_POINT('Ctrl Pts',(18.689397148694,-10.8254413080832,-3.79760667526428));
#95743=CARTESIAN_POINT('Ctrl Pts',(18.6666931274324,-11.1039771111179,-2.99885926159179));
#95744=CARTESIAN_POINT('Ctrl Pts',(18.6432974588946,-11.2949540425782,-2.16996449215795));
#95745=CARTESIAN_POINT('Ctrl Pts',(18.6172478588867,-11.3918346917951,-1.33096655160278));
#95746=CARTESIAN_POINT('Ctrl Pts',(18.6136145412749,-11.4053473049997,-1.21394571470871));
#95747=CARTESIAN_POINT('Ctrl Pts',(18.6099295983133,-11.4170294700437,-1.0967283249332));
#95748=CARTESIAN_POINT('Ctrl Pts',(18.6061877098378,-11.4268635310544,-0.979368755714328));
#95749=CARTESIAN_POINT('Ctrl Pts',(18.6061870500506,-11.4268652650419,-0.979348062328425));
#95750=CARTESIAN_POINT('Ctrl Pts',(18.6061863902616,-11.4268669989719,-0.979327368938115));
#95751=CARTESIAN_POINT('Ctrl Pts',(18.6061857304709,-11.4268687328444,-0.979306675543372));
#95752=CARTESIAN_POINT('Ctrl Pts',(18.5834005247388,-11.4867462659404,-0.264681229497011));
#95753=CARTESIAN_POINT('Ctrl Pts',(18.5584830336108,-11.478078130921,0.455221826164347));
#95754=CARTESIAN_POINT('Ctrl Pts',(18.5323945625552,-11.4029360819467,1.16806210182922));
#95755=CARTESIAN_POINT('Ctrl Pts',(18.5066208390778,-11.3287005934944,1.87230222802751));
#95756=CARTESIAN_POINT('Ctrl Pts',(18.4797041152464,-11.1895856521491,2.56965049513616));
#95757=CARTESIAN_POINT('Ctrl Pts',(18.452570095882,-10.9875404649071,3.24821661673467));
#95758=CARTESIAN_POINT('Ctrl Pts',(18.4374500639232,-10.8749537652667,3.62633757651284));
#95759=CARTESIAN_POINT('Ctrl Pts',(18.4222625456683,-10.7428256417688,3.99862650688148));
#95760=CARTESIAN_POINT('Ctrl Pts',(18.4071677397897,-10.591486415767,4.36302445712109));
#95761=CARTESIAN_POINT('Ctrl Pts',(18.4071644116394,-10.5914530480183,4.3631048007276));
#95762=CARTESIAN_POINT('Ctrl Pts',(18.4071610834933,-10.5914196793356,4.36318514394952));
#95763=CARTESIAN_POINT('Ctrl Pts',(18.4071577553514,-10.5913863097188,4.36326548678688));
#95764=CARTESIAN_POINT('Ctrl Pts',(18.3820082452178,-10.3392247339024,4.97038592893616));
#95765=CARTESIAN_POINT('Ctrl Pts',(18.3570973782381,-10.0337233596071,5.55554420614552));
#95766=CARTESIAN_POINT('Ctrl Pts',(18.3323202199419,-9.68078489052606,6.11065375339466));
#95767=CARTESIAN_POINT('Ctrl Pts',(18.3079231460669,-9.3332605376296,6.65724785716777));
#95768=CARTESIAN_POINT('Ctrl Pts',(18.2836556957903,-8.93974412258217,7.17470688012032));
#95769=CARTESIAN_POINT('Ctrl Pts',(18.2594178245586,-8.50591348580286,7.65533477953397));
#95770=CARTESIAN_POINT('Ctrl Pts',(18.2401528907354,-8.16109283599554,8.03735119456104));
#95771=CARTESIAN_POINT('Ctrl Pts',(18.2209066430271,-7.79080458210409,8.39609973384926));
#95772=CARTESIAN_POINT('Ctrl Pts',(18.2016290017132,-7.39791434534383,8.72773455289831));
#95773=CARTESIAN_POINT('Ctrl Pts',(18.2016255775624,-7.39784455903638,8.72779345884017));
#95774=CARTESIAN_POINT('Ctrl Pts',(18.2016221534106,-7.39777477201591,8.72785236392661));
#95775=CARTESIAN_POINT('Ctrl Pts',(18.2016187292579,-7.39770498428236,8.72791126815769));
#95776=CARTESIAN_POINT('Ctrl Pts',(18.1823945443621,-7.00589644234068,9.05861667612544));
#95777=CARTESIAN_POINT('Ctrl Pts',(18.163049995771,-6.59146899869525,9.36233212467602));
#95778=CARTESIAN_POINT('Ctrl Pts',(18.1436704590147,-6.15866743141592,9.63698434701735));
#95779=CARTESIAN_POINT('Ctrl Pts',(18.1243556225998,-5.72731081142756,9.91071961800122));
#95780=CARTESIAN_POINT('Ctrl Pts',(18.105006048155,-5.27770302579153,10.1555864360692));
#95781=CARTESIAN_POINT('Ctrl Pts',(18.0857040287375,-4.8139995903071,10.3695537217475));
#95782=CARTESIAN_POINT('Ctrl Pts',(18.0666496124358,-4.35624446587525,10.5807762704389));
#95783=CARTESIAN_POINT('Ctrl Pts',(18.0476414992938,-3.88475311646732,10.7618881686774));
#95784=CARTESIAN_POINT('Ctrl Pts',(18.028756860855,-3.40347319721907,10.9109396938641));
#95785=CARTESIAN_POINT('Ctrl Pts',(18.017902919585,-3.12685768271607,10.9966070210848));
#95786=CARTESIAN_POINT('Ctrl Pts',(18.0070897307925,-2.84700769423683,11.0716836019147));
#95787=CARTESIAN_POINT('Ctrl Pts',(17.9963317599933,-2.56466511419696,11.135797362719));
#95788=CARTESIAN_POINT('Ctrl Pts',(17.9963311846464,-2.56465001423521,11.1358007915867));
#95789=CARTESIAN_POINT('Ctrl Pts',(17.9963306092995,-2.56463491426632,11.135804220423));
#95790=CARTESIAN_POINT('Ctrl Pts',(17.9963300339529,-2.56461981429031,11.1358076492279));
#95791=CARTESIAN_POINT('Ctrl Pts',(17.9768958491772,-2.05456952995011,11.2516265701319));
#95792=CARTESIAN_POINT('Ctrl Pts',(17.9574004091647,-1.53644606554202,11.331299040876));
#95793=CARTESIAN_POINT('Ctrl Pts',(17.9378512061723,-1.0153381659182,11.3752735917127));
#95794=CARTESIAN_POINT('Ctrl Pts',(17.9234700491171,-0.631990847352272,
11.4076229883742));
#95795=CARTESIAN_POINT('Ctrl Pts',(17.9090597997092,-0.247028601760643,
11.4206550469504));
#95796=CARTESIAN_POINT('Ctrl Pts',(17.8946234605342,0.137526945126385,11.414565855171));
#95797=CARTESIAN_POINT('Ctrl Pts',(17.8794344836361,0.542131273611075,11.408159203724));
#95798=CARTESIAN_POINT('Ctrl Pts',(17.8642540867261,0.946288682112462,11.3806441565564));
#95799=CARTESIAN_POINT('Ctrl Pts',(17.8490764860305,1.34782593038233,11.3322244716497));
#95800=CARTESIAN_POINT('Ctrl Pts',(17.8339924594865,1.74688758925703,11.2841033076374));
#95801=CARTESIAN_POINT('Ctrl Pts',(17.8189111952324,2.14336221523588,11.2153343458876));
#95802=CARTESIAN_POINT('Ctrl Pts',(17.8038270235645,2.53510906264001,11.1260671287608));
#95803=CARTESIAN_POINT('Ctrl Pts',(17.8000535704286,2.63310836962008,11.103736060949));
#95804=CARTESIAN_POINT('Ctrl Pts',(17.7962799353667,2.73081173799778,11.0801219712589));
#95805=CARTESIAN_POINT('Ctrl Pts',(17.7925060296454,2.82818547696053,11.055226717161));
#95806=CARTESIAN_POINT('Ctrl Pts',(17.7828056836779,3.07847232190678,10.9912366242605));
#95807=CARTESIAN_POINT('Ctrl Pts',(17.7728937466464,3.32652271866186,10.9184862906763));
#95808=CARTESIAN_POINT('Ctrl Pts',(17.7629110876035,3.57174719113817,10.8372136533684));
#95809=CARTESIAN_POINT('Ctrl Pts',(17.7553786878304,3.75678093344116,10.775889511956));
#95810=CARTESIAN_POINT('Ctrl Pts',(17.7478060134944,3.94020683028634,10.7097132161103));
#95811=CARTESIAN_POINT('Ctrl Pts',(17.7402525390214,4.12179077946943,10.6387825823858));
#95812=CARTESIAN_POINT('Ctrl Pts',(17.7343980689171,4.26253101837736,10.5838063888335));
#95813=CARTESIAN_POINT('Ctrl Pts',(17.7285938577166,4.40218261181708,10.5260274920075));
#95814=CARTESIAN_POINT('Ctrl Pts',(17.7228420832576,4.54061669736803,10.465461273219));
#95815=CARTESIAN_POINT('Ctrl Pts',(17.7156518837169,4.71367089228399,10.389748429884));
#95816=CARTESIAN_POINT('Ctrl Pts',(17.7085436164182,4.88482235323807,10.3096796974154));
#95817=CARTESIAN_POINT('Ctrl Pts',(17.7015219415102,5.05388155833274,10.2254292304244));
#95818=CARTESIAN_POINT('Ctrl Pts',(17.6871005257297,5.40110257327522,10.0523920234788));
#95819=CARTESIAN_POINT('Ctrl Pts',(17.6727915987991,5.73922499208294,9.86143185706003));
#95820=CARTESIAN_POINT('Ctrl Pts',(17.6584917271518,6.06671669227161,9.65383289905655));
#95821=CARTESIAN_POINT('Ctrl Pts',(17.6441416360901,6.39535850357742,9.44550487870013));
#95822=CARTESIAN_POINT('Ctrl Pts',(17.6298006652466,6.71329440145111,9.22041996616636));
#95823=CARTESIAN_POINT('Ctrl Pts',(17.6153658278202,7.0189267110527,8.97989280350298));
#95824=CARTESIAN_POINT('Ctrl Pts',(17.6063665968301,7.20946960882593,8.82993895004162));
#95825=CARTESIAN_POINT('Ctrl Pts',(17.597330904034,7.39522944235641,8.67398348006849));
#95826=CARTESIAN_POINT('Ctrl Pts',(17.5882342232595,7.57581058956664,8.5123507333688));
#95827=CARTESIAN_POINT('Ctrl Pts',(17.570801635833,7.92187051124135,8.20260291900894));
#95828=CARTESIAN_POINT('Ctrl Pts',(17.5532521221025,8.24925679949015,7.87193935681038));
#95829=CARTESIAN_POINT('Ctrl Pts',(17.5356012364988,8.55538584983627,7.52267230287006));
#95830=CARTESIAN_POINT('Ctrl Pts',(17.5188462385182,8.84597702670678,7.19113263313973));
#95831=CARTESIAN_POINT('Ctrl Pts',(17.5019999135686,9.11741460146095,6.8428292824108));
#95832=CARTESIAN_POINT('Ctrl Pts',(17.4850755148002,9.36745291600106,6.47971529953186));
#95833=CARTESIAN_POINT('Ctrl Pts',(17.4734938848635,9.53855803285768,6.23123073992728));
#95834=CARTESIAN_POINT('Ctrl Pts',(17.4620681140206,9.69985748204413,5.97600618604054));
#95835=CARTESIAN_POINT('Ctrl Pts',(17.4508315775933,9.85063309773795,5.71477009049237));
#95836=CARTESIAN_POINT('Ctrl Pts',(17.445209014683,9.92607853326528,5.58405219613394));
#95837=CARTESIAN_POINT('Ctrl Pts',(17.4396338452531,9.99888949830509,5.45182917745403));
#95838=CARTESIAN_POINT('Ctrl Pts',(17.4341103385296,10.0690450450509,5.31822958070305));
#95839=CARTESIAN_POINT('Ctrl Pts',(17.4253224355891,10.1806625674672,5.10567253173293));
#95840=CARTESIAN_POINT('Ctrl Pts',(17.4166052134124,10.2854698674235,4.88959849063566));
#95841=CARTESIAN_POINT('Ctrl Pts',(17.407821599972,10.3831861088303,4.67040458670955));
#95842=CARTESIAN_POINT('Ctrl Pts',(17.4000512154975,10.4696303461929,4.47649567672039));
#95843=CARTESIAN_POINT('Ctrl Pts',(17.3922288216349,10.5505245652096,4.28014573517023));
#95844=CARTESIAN_POINT('Ctrl Pts',(17.3842603515511,10.6256619800217,4.08166139633652));
#95845=CARTESIAN_POINT('Ctrl Pts',(17.3694478756162,10.7653338539217,3.7127016761487));
#95846=CARTESIAN_POINT('Ctrl Pts',(17.3546425838804,10.8858945263555,3.33657659901067));
#95847=CARTESIAN_POINT('Ctrl Pts',(17.3398311092709,10.9869532301011,2.95529661764224));
#95848=CARTESIAN_POINT('Ctrl Pts',(17.3250017259557,11.0881341249612,2.57355562674091));
#95849=CARTESIAN_POINT('Ctrl Pts',(17.3101661438342,11.1697659678492,2.18664632400007));
#95850=CARTESIAN_POINT('Ctrl Pts',(17.2953111696126,11.2314054174755,1.7965788629401));
#95851=CARTESIAN_POINT('Ctrl Pts',(17.2909948894645,11.2493154541267,1.6832403667923));
#95852=CARTESIAN_POINT('Ctrl Pts',(17.2866769736132,11.2655372811745,1.56963524128526));
#95853=CARTESIAN_POINT('Ctrl Pts',(17.2823571021727,11.2800591949974,1.45581285081457));
#95854=CARTESIAN_POINT('Ctrl Pts',(17.269239278253,11.3241567824215,1.1101770843575));
#95855=CARTESIAN_POINT('Ctrl Pts',(17.2560129092754,11.3524343047511,0.762525396881152));
#95856=CARTESIAN_POINT('Ctrl Pts',(17.2427740669595,11.3647067757544,0.414395378551398));
#95857=CARTESIAN_POINT('Ctrl Pts',(17.2295616876319,11.3769547154392,0.0669612338036552));
#95858=CARTESIAN_POINT('Ctrl Pts',(17.2163368990233,11.3732623098732,-0.280949084064888));
#95859=CARTESIAN_POINT('Ctrl Pts',(17.2031927160801,11.3534609095458,-0.627856637969633));
#95860=CARTESIAN_POINT('Ctrl Pts',(17.195334121398,11.3416221227621,-0.835264422088129));
#95861=CARTESIAN_POINT('Ctrl Pts',(17.1875042852075,11.3240253214374,-1.04231473548696));
#95862=CARTESIAN_POINT('Ctrl Pts',(17.179722732406,11.3006352045343,-1.2487003895174));
#95863=CARTESIAN_POINT('Ctrl Pts',(17.1797220690039,11.3006332104526,-1.24871798454966));
#95864=CARTESIAN_POINT('Ctrl Pts',(17.1797214056021,11.3006312163286,-1.24873557957695));
#95865=CARTESIAN_POINT('Ctrl Pts',(17.1797207422005,11.3006292221623,-1.24875317459922));
#95866=CARTESIAN_POINT('Ctrl Pts',(17.1664171336884,11.2606389538955,-1.60159720896684));
#95867=CARTESIAN_POINT('Ctrl Pts',(17.1532153799316,11.2036540450757,-1.95243587269292));
#95868=CARTESIAN_POINT('Ctrl Pts',(17.1400310196288,11.1302347366909,-2.29979918441093));
#95869=CARTESIAN_POINT('Ctrl Pts',(17.1268509988193,11.0568395934985,-2.64704816515195));
#95870=CARTESIAN_POINT('Ctrl Pts',(17.1136883759637,10.9670201751712,-2.99082366113072));
#95871=CARTESIAN_POINT('Ctrl Pts',(17.1004602987123,10.8613632646006,-3.32961276547741));
#95872=CARTESIAN_POINT('Ctrl Pts',(17.093264264523,10.8038862234286,-3.51391301800193));
#95873=CARTESIAN_POINT('Ctrl Pts',(17.0860488828582,10.7417228848526,-3.69673689788994));
#95874=CARTESIAN_POINT('Ctrl Pts',(17.0788010422857,10.6749721170883,-3.87783609052177));
#95875=CARTESIAN_POINT('Ctrl Pts',(17.0618512862622,10.5188691762622,-4.30135356452081));
#95876=CARTESIAN_POINT('Ctrl Pts',(17.0449116121264,10.3379612816245,-4.71558713436491));
#95877=CARTESIAN_POINT('Ctrl Pts',(17.0279776992362,10.1336467949107,-5.11775193322988));
#95878=CARTESIAN_POINT('Ctrl Pts',(17.0147660258491,9.97424262859502,-5.43151698002458));
#95879=CARTESIAN_POINT('Ctrl Pts',(17.0015577606713,9.80059010964242,-5.73793916776007));
#95880=CARTESIAN_POINT('Ctrl Pts',(16.9883050898332,9.61323203514672,-6.03569643286859));
#95881=CARTESIAN_POINT('Ctrl Pts',(16.9845712997621,9.56044601738282,-6.11958617355713));
#95882=CARTESIAN_POINT('Ctrl Pts',(16.9808339915489,9.50657195391244,-6.20278783938413));
#95883=CARTESIAN_POINT('Ctrl Pts',(16.9770921125338,9.45162167652532,-6.28527117954114));
#95884=CARTESIAN_POINT('Ctrl Pts',(16.9608377334333,9.21292271359193,-6.6435712408139));
#95885=CARTESIAN_POINT('Ctrl Pts',(16.9446245873696,8.95405231378699,-6.98850040250276));
#95886=CARTESIAN_POINT('Ctrl Pts',(16.9284389646338,8.67621779025595,-7.31739009469023));
#95887=CARTESIAN_POINT('Ctrl Pts',(16.9220180229297,8.56599902956192,-7.44786277251745));
#95888=CARTESIAN_POINT('Ctrl Pts',(16.9156014195238,8.45279634404502,-7.57581128912845));
#95889=CARTESIAN_POINT('Ctrl Pts',(16.9091883236421,8.33668733010234,-7.70106952046181));
#95890=CARTESIAN_POINT('Ctrl Pts',(16.8931331960915,8.0460094635932,-8.01465236997828));
#95891=CARTESIAN_POINT('Ctrl Pts',(16.8771000186673,7.73711305391114,-8.31137203881411));
#95892=CARTESIAN_POINT('Ctrl Pts',(16.8610758846774,7.4124119890984,-8.58963890716383));
#95893=CARTESIAN_POINT('Ctrl Pts',(16.845044908476,7.08757227883031,-8.86802459383862));
#95894=CARTESIAN_POINT('Ctrl Pts',(16.8290229844305,6.74691507681148,-9.12794100812106));
#95895=CARTESIAN_POINT('Ctrl Pts',(16.8129976534456,6.39289795770402,-9.36782843649133));
#95896=CARTESIAN_POINT('Ctrl Pts',(16.8000012737082,6.10579369022996,-9.56237469055983));
#95897=CARTESIAN_POINT('Ctrl Pts',(16.7870026607976,5.8099034735611,-9.74374822440784));
#95898=CARTESIAN_POINT('Ctrl Pts',(16.7739953989264,5.50655304996275,-9.91113745714248));
#95899=CARTESIAN_POINT('Ctrl Pts',(16.7589630605645,5.15597456120005,-10.1045872092515));
#95900=CARTESIAN_POINT('Ctrl Pts',(16.7439297861409,4.79518685920721,-10.2795409072731));
#95901=CARTESIAN_POINT('Ctrl Pts',(16.7288930927054,4.42613322613574,-10.4347396739405));
#95902=CARTESIAN_POINT('Ctrl Pts',(16.7059890749003,3.86398763081691,-10.6711397395757));
#95903=CARTESIAN_POINT('Ctrl Pts',(16.6830771012879,3.28266179623832,-10.8617032120053));
#95904=CARTESIAN_POINT('Ctrl Pts',(16.660149213089,2.68995422151479,-11.0047568660834));
#95905=CARTESIAN_POINT('Ctrl Pts',(16.6366666976463,2.08290900846487,-11.1512709982133));
#95906=CARTESIAN_POINT('Ctrl Pts',(16.613167482723,1.46392562965263,-11.2479482536141));
#95907=CARTESIAN_POINT('Ctrl Pts',(16.5896435621228,0.841421641600292,-11.29302792262));
#95908=CARTESIAN_POINT('Ctrl Pts',(16.583381022206,0.675698582941044,-11.3050290355034));
#95909=CARTESIAN_POINT('Ctrl Pts',(16.5771167345246,0.509726175893628,-11.3133734986216));
#95910=CARTESIAN_POINT('Ctrl Pts',(16.5708505551953,0.343663562097396,-11.3180286219251));
#95911=CARTESIAN_POINT('Ctrl Pts',(16.563309919019,0.143826039527265,-11.3236305348842));
#95912=CARTESIAN_POINT('Ctrl Pts',(16.555780015154,-0.0561365062592693,
-11.3239139818911));
#95913=CARTESIAN_POINT('Ctrl Pts',(16.5482589551089,-0.255950842440518,
-11.3188205116742));
#95914=CARTESIAN_POINT('Ctrl Pts',(16.5254989223572,-0.860623695532547,
-11.3034067869783));
#95915=CARTESIAN_POINT('Ctrl Pts',(16.5028197022815,-1.46394306304044,-11.2387517590465));
#95916=CARTESIAN_POINT('Ctrl Pts',(16.4801704660534,-2.05826210501978,-11.1267611656254));
#95917=CARTESIAN_POINT('Ctrl Pts',(16.4577078735389,-2.64768359054951,-11.0156934439522));
#95918=CARTESIAN_POINT('Ctrl Pts',(16.4352747935128,-3.22825166601579,-10.8580657122636));
#95919=CARTESIAN_POINT('Ctrl Pts',(16.4128237642916,-3.79246292298964,-10.6557613845628));
#95920=CARTESIAN_POINT('Ctrl Pts',(16.3980607989102,-4.16346735100046,-10.522733550653));
#95921=CARTESIAN_POINT('Ctrl Pts',(16.3832901110842,-4.52739834561009,-10.3703885974072));
#95922=CARTESIAN_POINT('Ctrl Pts',(16.3684987026711,-4.88211519408174,-10.1992720087013));
#95923=CARTESIAN_POINT('Ctrl Pts',(16.3684981996459,-4.88212725726756,-10.1992661893803));
#95924=CARTESIAN_POINT('Ctrl Pts',(16.3684976966207,-4.8821393204427,-10.1992603700376));
#95925=CARTESIAN_POINT('Ctrl Pts',(16.3684971935955,-4.88215138360721,-10.1992545506731));
#95926=CARTESIAN_POINT('Ctrl Pts',(16.3510590516397,-5.30033950116647,-9.99751734883505));
#95927=CARTESIAN_POINT('Ctrl Pts',(16.3334957030325,-5.70581057641984,-9.76945707877262));
#95928=CARTESIAN_POINT('Ctrl Pts',(16.3158833545317,-6.09580305607242,-9.51735400966098));
#95929=CARTESIAN_POINT('Ctrl Pts',(16.298271006031,-6.485795535725,-9.26525094054935));
#95930=CARTESIAN_POINT('Ctrl Pts',(16.2806097240013,-6.86031024912703,-8.98910619483964));
#95931=CARTESIAN_POINT('Ctrl Pts',(16.2629726827512,-7.21663392926645,-8.69116642701088));
#95932=CARTESIAN_POINT('Ctrl Pts',(16.2483995158922,-7.51105771457272,-8.44498420807137));
#95933=CARTESIAN_POINT('Ctrl Pts',(16.2339252337094,-7.79315311500984,-8.18404924571618));
#95934=CARTESIAN_POINT('Ctrl Pts',(16.2195735026631,-8.06130761505714,-7.90967958982998));
#95935=CARTESIAN_POINT('Ctrl Pts',(16.2089571825821,-8.25966793789824,-7.70672176697118));
#95936=CARTESIAN_POINT('Ctrl Pts',(16.1984079167211,-8.45040074228537,-7.49641327831099));
#95937=CARTESIAN_POINT('Ctrl Pts',(16.1879354848093,-8.63287033435264,-7.27929465333164));
#95938=CARTESIAN_POINT('Ctrl Pts',(16.1855091838064,-8.67514572539506,-7.22899161560571));
#95939=CARTESIAN_POINT('Ctrl Pts',(16.1830870082473,-8.71697763175051,-7.17832304343388));
#95940=CARTESIAN_POINT('Ctrl Pts',(16.1806690820714,-8.75836150028961,-7.12729848826442));
#95941=CARTESIAN_POINT('Ctrl Pts',(16.1682911799108,-8.97021473258396,-6.86609243574614));
#95942=CARTESIAN_POINT('Ctrl Pts',(16.1558057071422,-9.1699270812072,-6.59534961160817));
#95943=CARTESIAN_POINT('Ctrl Pts',(16.1432642674463,-9.35701879829506,-6.31633651487297));
#95944=CARTESIAN_POINT('Ctrl Pts',(16.1306238735717,-9.54558670214291,-6.03512195542379));
#95945=CARTESIAN_POINT('Ctrl Pts',(16.1179266926506,-9.72133466453958,-5.74550612004991));
#95946=CARTESIAN_POINT('Ctrl Pts',(16.1052247240192,-9.88377661046624,-5.44873326416131));
#95947=CARTESIAN_POINT('Ctrl Pts',(16.1030773577283,-9.91123868103423,-5.39856151163407));
#95948=CARTESIAN_POINT('Ctrl Pts',(16.1009298515565,-9.93832045718344,-5.34818508711592));
#95949=CARTESIAN_POINT('Ctrl Pts',(16.0987824528555,-9.96501958366583,-5.29760985599476));
#95950=CARTESIAN_POINT('Ctrl Pts',(16.0810524102623,-10.1854614836817,-4.88003439526046));
#95951=CARTESIAN_POINT('Ctrl Pts',(16.0632530007794,-10.3798600347158,-4.44855263773922));
#95952=CARTESIAN_POINT('Ctrl Pts',(16.0453685199868,-10.5463722689621,-4.00643121409874));
#95953=CARTESIAN_POINT('Ctrl Pts',(16.033077414964,-10.6608077609632,-3.70258337452398));
#95954=CARTESIAN_POINT('Ctrl Pts',(16.0207461488524,-10.7620713071895,-3.39371069163026));
#95955=CARTESIAN_POINT('Ctrl Pts',(16.0083699646992,-10.8495527626949,-3.08088155401435));
#95956=CARTESIAN_POINT('Ctrl Pts',(16.0035940901124,-10.8833111857265,-2.9601631880107));
#95957=CARTESIAN_POINT('Ctrl Pts',(15.9988115299569,-10.9150171691888,-2.83885573418935));
#95958=CARTESIAN_POINT('Ctrl Pts',(15.9940220242916,-10.9446640919374,-2.71702798364124));
#95959=CARTESIAN_POINT('Ctrl Pts',(15.9807342044901,-11.0269153710227,-2.37903377103331));
#95960=CARTESIAN_POINT('Ctrl Pts',(15.9676012984832,-11.0937025818476,-2.037245337332));
#95961=CARTESIAN_POINT('Ctrl Pts',(15.9545647436297,-11.1448107093041,-1.69315726102379));
#95962=CARTESIAN_POINT('Ctrl Pts',(15.9415160036568,-11.1959666069453,-1.34874756950933));
#95963=CARTESIAN_POINT('Ctrl Pts',(15.9285639096431,-11.2314133261888,-1.00203424509647));
#95964=CARTESIAN_POINT('Ctrl Pts',(15.9156522578572,-11.2509545749342,-0.654564312121401));
#95965=CARTESIAN_POINT('Ctrl Pts',(15.9142425832482,-11.2530880589098,-0.616628070499019));
#95966=CARTESIAN_POINT('Ctrl Pts',(15.9128333923135,-11.2550319762816,-0.57868285440704));
#95967=CARTESIAN_POINT('Ctrl Pts',(15.9114246129926,-11.2567860916136,-0.540730709036398));
#95968=CARTESIAN_POINT('Ctrl Pts',(15.896297122496,-11.2756218046469,-0.133200083115572));
#95969=CARTESIAN_POINT('Ctrl Pts',(15.8811812274722,-11.2724972532996,0.275133806617833));
#95970=CARTESIAN_POINT('Ctrl Pts',(15.866009903517,-11.2471854056454,0.681880736138495));
#95971=CARTESIAN_POINT('Ctrl Pts',(15.8538996454936,-11.2269806425646,1.00655973457034));
#95972=CARTESIAN_POINT('Ctrl Pts',(15.8417540721048,-11.1926381024088,1.33022661539188));
#95973=CARTESIAN_POINT('Ctrl Pts',(15.8295400541171,-11.1440408971964,1.65164183924907));
#95974=CARTESIAN_POINT('Ctrl Pts',(15.8295391702672,-11.1440373805293,1.6516650980013));
#95975=CARTESIAN_POINT('Ctrl Pts',(15.8295382864169,-11.1440338637875,1.65168835674174));
#95976=CARTESIAN_POINT('Ctrl Pts',(15.8295374025663,-11.1440303469711,1.65171161547037));
#95977=CARTESIAN_POINT('Ctrl Pts',(15.816784962099,-11.093288750435,1.98729496184131));
#95978=CARTESIAN_POINT('Ctrl Pts',(15.8039130298149,-11.0269101699919,2.32045746517097));
#95979=CARTESIAN_POINT('Ctrl Pts',(15.7909874558207,-10.9455312672853,2.64991634597987));
#95980=CARTESIAN_POINT('Ctrl Pts',(15.7780454877898,-10.8640491483724,2.97979309302464));
#95981=CARTESIAN_POINT('Ctrl Pts',(15.7650498239764,-10.7675292664881,3.30595720866079));
#95982=CARTESIAN_POINT('Ctrl Pts',(15.75206424864,-10.6565846729906,3.62716614328774));
#95983=CARTESIAN_POINT('Ctrl Pts',(15.7426825785663,-10.5764306909228,3.85922950369542));
#95984=CARTESIAN_POINT('Ctrl Pts',(15.7333061132432,-10.488747063491,4.08870743526162));
#95985=CARTESIAN_POINT('Ctrl Pts',(15.7239579733421,-10.3937536873271,4.31514398655314));
#95986=CARTESIAN_POINT('Ctrl Pts',(15.7107915749463,-10.2599601574097,4.63406880766187));
#95987=CARTESIAN_POINT('Ctrl Pts',(15.6976909195897,-10.1116875116354,4.9469541132507));
#95988=CARTESIAN_POINT('Ctrl Pts',(15.6847177269443,-9.94958308666377,5.2524241885062));
#95989=CARTESIAN_POINT('Ctrl Pts',(15.6727187110484,-9.79965132929213,5.53495605162788));
#95990=CARTESIAN_POINT('Ctrl Pts',(15.6608285954209,-9.63788771127589,5.811145088744));
#95991=CARTESIAN_POINT('Ctrl Pts',(15.6490961272982,-9.46479960650109,6.07994229205141));
#95992=CARTESIAN_POINT('Ctrl Pts',(15.6467196831804,-9.42974012846632,6.13438791474411));
#95993=CARTESIAN_POINT('Ctrl Pts',(15.6443497106583,-9.39421600074739,6.18853039061903));
#95994=CARTESIAN_POINT('Ctrl Pts',(15.6419866226875,-9.35823486758082,6.24236374822694));
#95995=CARTESIAN_POINT('Ctrl Pts',(15.6269862132743,-9.12983383667652,6.58408712635861));
#95996=CARTESIAN_POINT('Ctrl Pts',(15.611834850162,-8.8822881668317,6.91267923813996));
#95997=CARTESIAN_POINT('Ctrl Pts',(15.5965715424223,-8.61750993968684,7.22650596940827));
#95998=CARTESIAN_POINT('Ctrl Pts',(15.584724568317,-8.41199611174719,7.47008994362021));
#95999=CARTESIAN_POINT('Ctrl Pts',(15.5728102156546,-8.19609987425416,7.7047794729152));
#96000=CARTESIAN_POINT('Ctrl Pts',(15.5608469949931,-7.97069767366566,7.92982292259678));
#96001=CARTESIAN_POINT('Ctrl Pts',(15.546547793163,-7.70128263482498,8.1988091595479));
#96002=CARTESIAN_POINT('Ctrl Pts',(15.5322500538376,-7.41833237647199,8.45421872950808));
#96003=CARTESIAN_POINT('Ctrl Pts',(15.5179489803913,-7.12315253349482,8.69476756943813));
#96004=CARTESIAN_POINT('Ctrl Pts',(15.5154829894361,-7.07225349953903,8.73624636232635));
#96005=CARTESIAN_POINT('Ctrl Pts',(15.5130168993599,-7.02099076553669,8.77728319147544));
#96006=CARTESIAN_POINT('Ctrl Pts',(15.5105506855879,-6.96937094029732,8.81787134061039));
#96007=CARTESIAN_POINT('Ctrl Pts',(15.4974931629857,-6.69606655670022,9.03276782716831));
#96008=CARTESIAN_POINT('Ctrl Pts',(15.4844339968103,-6.41278921190233,9.23505585109763));
#96009=CARTESIAN_POINT('Ctrl Pts',(15.4713723156188,-6.12063727973133,9.42366104347754));
#96010=CARTESIAN_POINT('Ctrl Pts',(15.4537235811276,-5.72588626671685,9.67850135960518));
#96011=CARTESIAN_POINT('Ctrl Pts',(15.436070244661,-5.31493186286818,9.90835908134703));
#96012=CARTESIAN_POINT('Ctrl Pts',(15.4184103849752,-4.89133265966661,10.1117089124309));
#96013=CARTESIAN_POINT('Ctrl Pts',(15.4007051415832,-4.46664485768154,10.3155813280171));
#96014=CARTESIAN_POINT('Ctrl Pts',(15.3829933396985,-4.02924810549658,10.4928088688309));
#96015=CARTESIAN_POINT('Ctrl Pts',(15.3652733218964,-3.58275659444785,10.6418978456182));
#96016=CARTESIAN_POINT('Ctrl Pts',(15.3633532580213,-3.53437672088036,10.6580524771595));
#96017=CARTESIAN_POINT('Ctrl Pts',(15.3614330979687,-3.48589008528935,10.6738767821366));
#96018=CARTESIAN_POINT('Ctrl Pts',(15.3595128398411,-3.43730129811629,10.6893688951891));
#96019=CARTESIAN_POINT('Ctrl Pts',(15.3503867735382,-3.20638208630126,10.7629954815599));
#96020=CARTESIAN_POINT('Ctrl Pts',(15.3411706767005,-2.97305390698645,10.8289328157232));
#96021=CARTESIAN_POINT('Ctrl Pts',(15.3319491449979,-2.73785862511626,10.8871720241923));
#96022=CARTESIAN_POINT('Ctrl Pts',(15.3241947349801,-2.54008230023958,10.9361455262249));
#96023=CARTESIAN_POINT('Ctrl Pts',(15.3164364503988,-2.34098490422853,10.9796760416066));
#96024=CARTESIAN_POINT('Ctrl Pts',(15.3087231597288,-2.14086073602318,11.0177641579777));
#96025=CARTESIAN_POINT('Ctrl Pts',(15.3030975434798,-1.99490204982233,11.045543368631));
#96026=CARTESIAN_POINT('Ctrl Pts',(15.2975031964061,-1.84840170014174,11.0704447887901));
#96027=CARTESIAN_POINT('Ctrl Pts',(15.2919401866255,-1.70147371298188,11.0924211245245));
#96028=CARTESIAN_POINT('Ctrl Pts',(15.2849796942184,-1.51763597417496,11.1199181313697));
#96029=CARTESIAN_POINT('Ctrl Pts',(15.2780682522276,-1.33312876471508,11.1428357490647));
#96030=CARTESIAN_POINT('Ctrl Pts',(15.2712062606979,-1.14818779157993,11.1612111263306));
#96031=CARTESIAN_POINT('Ctrl Pts',(15.2565513847108,-0.753216883420893,
11.2004546715735));
#96032=CARTESIAN_POINT('Ctrl Pts',(15.2417880158008,-0.356230914403019,
11.2181470297901));
#96033=CARTESIAN_POINT('Ctrl Pts',(15.2269407912071,0.0403976675311114,
11.2147424095226));
#96034=CARTESIAN_POINT('Ctrl Pts',(15.223025529029,0.144989934983414,11.2138445999098));
#96035=CARTESIAN_POINT('Ctrl Pts',(15.2191044397254,0.249557517966656,11.2114799435831));
#96036=CARTESIAN_POINT('Ctrl Pts',(15.2151779818984,0.354057296599062,11.2076572361261));
#96037=CARTESIAN_POINT('Ctrl Pts',(15.2022992179719,0.696816098215689,11.1951187729444));
#96038=CARTESIAN_POINT('Ctrl Pts',(15.1894285714027,1.03885434801065,11.167063534534));
#96039=CARTESIAN_POINT('Ctrl Pts',(15.176560634575,1.37888273726765,11.1237375046297));
#96040=CARTESIAN_POINT('Ctrl Pts',(15.1706282521209,1.53564278958491,11.1037633173881));
#96041=CARTESIAN_POINT('Ctrl Pts',(15.1646964456791,1.69197568407878,11.0805427435218));
#96042=CARTESIAN_POINT('Ctrl Pts',(15.1587646858145,1.84775483686978,11.0540961733022));
#96043=CARTESIAN_POINT('Ctrl Pts',(15.1453128659511,2.20102488651213,10.9941216452156));
#96044=CARTESIAN_POINT('Ctrl Pts',(15.1318527589919,2.55155730831782,10.9175263915371));
#96045=CARTESIAN_POINT('Ctrl Pts',(15.1183411040416,2.89768337032284,10.824420911768));
#96046=CARTESIAN_POINT('Ctrl Pts',(15.1048923411799,3.24219833501767,10.7317488058603));
#96047=CARTESIAN_POINT('Ctrl Pts',(15.0913924504108,3.58234777223796,10.6227191870421));
#96048=CARTESIAN_POINT('Ctrl Pts',(15.0778008782604,3.91643536896289,10.4974497033195));
#96049=CARTESIAN_POINT('Ctrl Pts',(15.0711231977693,4.08057607338532,10.4359035055486));
#96050=CARTESIAN_POINT('Ctrl Pts',(15.0644234239915,4.2432527662515,10.3704374251837));
#96051=CARTESIAN_POINT('Ctrl Pts',(15.0576970245877,4.40425989922078,10.3010668804539));
#96052=CARTESIAN_POINT('Ctrl Pts',(15.0463063079057,4.67691492984938,10.183592408055));
#96053=CARTESIAN_POINT('Ctrl Pts',(15.0350395082811,4.94494615285118,10.0554153771109));
#96054=CARTESIAN_POINT('Ctrl Pts',(15.0239216225122,5.20738442942893,9.91676673804391));
#96055=CARTESIAN_POINT('Ctrl Pts',(15.0183628066874,5.33860056846611,9.84744400304363));
#96056=CARTESIAN_POINT('Ctrl Pts',(15.0128412401794,5.46841903543546,9.7755038407282));
#96057=CARTESIAN_POINT('Ctrl Pts',(15.0073602513422,5.59675654054199,9.70104559446499));
#96058=CARTESIAN_POINT('Ctrl Pts',(14.9991386428056,5.78926573165558,9.58935652315283));
#96059=CARTESIAN_POINT('Ctrl Pts',(14.990982342604,5.97840148681949,9.47194440885129));
#96060=CARTESIAN_POINT('Ctrl Pts',(14.982793878564,6.16375328342834,9.34889430887797));
#96061=CARTESIAN_POINT('Ctrl Pts',(14.9746054145239,6.34910508003718,9.22584420890465));
#96062=CARTESIAN_POINT('Ctrl Pts',(14.9663846757789,6.53067257440623,9.09715565980792));
#96063=CARTESIAN_POINT('Ctrl Pts',(14.958035400268,6.70799664566802,8.96294977261773));
#96064=CARTESIAN_POINT('Ctrl Pts',(14.9438663009938,7.00892363821142,8.73519629433143));
#96065=CARTESIAN_POINT('Ctrl Pts',(14.9297048407444,7.29829892641942,8.49233128970611));
#96066=CARTESIAN_POINT('Ctrl Pts',(14.9155444032486,7.5748854850347,8.23573319682833));
#96067=CARTESIAN_POINT('Ctrl Pts',(14.9012834997017,7.85343438127926,7.97731458130559));
#96068=CARTESIAN_POINT('Ctrl Pts',(14.8870236331363,8.11901308083736,7.7049666699828));
#96069=CARTESIAN_POINT('Ctrl Pts',(14.8727581311784,8.37032354391681,7.42005806068027));
#96070=CARTESIAN_POINT('Ctrl Pts',(14.8678011884713,8.45764830618842,7.32105869443179));
#96071=CARTESIAN_POINT('Ctrl Pts',(14.8628435661219,8.54324996292118,7.22054243972945));
#96072=CARTESIAN_POINT('Ctrl Pts',(14.857884986722,8.6270728691673,7.11856583587876));
#96073=CARTESIAN_POINT('Ctrl Pts',(14.8456785387162,8.83341824840889,6.86753181740228));
#96074=CARTESIAN_POINT('Ctrl Pts',(14.8333979230135,9.02883460105979,6.60753129588973));
#96075=CARTESIAN_POINT('Ctrl Pts',(14.8211015218869,9.21253500466722,6.33960528723982));
#96076=CARTESIAN_POINT('Ctrl Pts',(14.8088177332149,9.39604698623265,6.07195409108165));
#96077=CARTESIAN_POINT('Ctrl Pts',(14.7965182230185,9.56786759034857,5.79639418886013));
#96078=CARTESIAN_POINT('Ctrl Pts',(14.784258731834,9.72724843380699,5.513926181261));
#96079=CARTESIAN_POINT('Ctrl Pts',(14.7752122552789,9.84485813244661,5.30548847615037));
#96080=CARTESIAN_POINT('Ctrl Pts',(14.7661874995261,9.95569494145445,5.09328842147978));
#96081=CARTESIAN_POINT('Ctrl Pts',(14.757206081749,10.0594678533509,4.8777126536179));
#96082=CARTESIAN_POINT('Ctrl Pts',(14.7571975315397,10.0595666440024,4.87750742789788));
#96083=CARTESIAN_POINT('Ctrl Pts',(14.7571889813498,10.0596654281814,4.87730219912515));
#96084=CARTESIAN_POINT('Ctrl Pts',(14.7571804311792,10.0597642058877,4.8770969673));
#96085=CARTESIAN_POINT('Ctrl Pts',(14.7417401730578,10.2381411483223,4.50648069317787));
#96086=CARTESIAN_POINT('Ctrl Pts',(14.7263628645334,10.3954128046633,4.1259070187093));
#96087=CARTESIAN_POINT('Ctrl Pts',(14.7110044208977,10.5311860218655,3.73780135474113));
#96088=CARTESIAN_POINT('Ctrl Pts',(14.6956232644371,10.6671600272069,3.34912174094907));
#96089=CARTESIAN_POINT('Ctrl Pts',(14.6802610526129,10.7815710421429,2.95288732267195));
#96090=CARTESIAN_POINT('Ctrl Pts',(14.6648752094907,10.8739972606444,2.55157887666387));
#96091=CARTESIAN_POINT('Ctrl Pts',(14.6514061812039,10.9549087415138,2.20026664969692));
#96092=CARTESIAN_POINT('Ctrl Pts',(14.6379190447941,11.018971273041,1.84506648378009));
#96093=CARTESIAN_POINT('Ctrl Pts',(14.624386376264,11.0658933994358,1.4876744121179));
#96094=CARTESIAN_POINT('Ctrl Pts',(14.6080772663412,11.122442343606,1.05695769358589));
#96095=CARTESIAN_POINT('Ctrl Pts',(14.591766379385,11.1543157325057,0.622938756550116));
#96096=CARTESIAN_POINT('Ctrl Pts',(14.5754370498476,11.161049334572,0.188663963741718));
#96097=CARTESIAN_POINT('Ctrl Pts',(14.5592396394342,11.1677285381474,-0.242102470069903));
#96098=CARTESIAN_POINT('Ctrl Pts',(14.5430240690424,11.1496719435507,-0.67311983496954));
#96099=CARTESIAN_POINT('Ctrl Pts',(14.5267752198866,11.1064667572452,-1.1013843654405));
#96100=CARTESIAN_POINT('Ctrl Pts',(14.5147782440051,11.0745671701981,-1.41758394324903));
#96101=CARTESIAN_POINT('Ctrl Pts',(14.5027631463582,11.0289591688627,-1.73228216587942));
#96102=CARTESIAN_POINT('Ctrl Pts',(14.4907243493819,10.9694936230759,-2.04426332029249));
#96103=CARTESIAN_POINT('Ctrl Pts',(14.4907194949762,10.969469644776,-2.04438912049456));
#96104=CARTESIAN_POINT('Ctrl Pts',(14.4907146405667,10.9694456642232,-2.04451492025482));
#96105=CARTESIAN_POINT('Ctrl Pts',(14.4907097861533,10.9694216814175,-2.04464071957316));
#96106=CARTESIAN_POINT('Ctrl Pts',(14.4730988720036,10.8824164968376,-2.50101738523806));
#96107=CARTESIAN_POINT('Ctrl Pts',(14.4554966900047,10.7659459820233,-2.95158140987517));
#96108=CARTESIAN_POINT('Ctrl Pts',(14.4379151671712,10.6218907828759,-3.39316742440224));
#96109=CARTESIAN_POINT('Ctrl Pts',(14.419954168372,10.4747263259973,-3.84428454046353));
#96110=CARTESIAN_POINT('Ctrl Pts',(14.4020147262933,10.298773834897,-4.28603272975413));
#96111=CARTESIAN_POINT('Ctrl Pts',(14.384108374905,10.0959871954966,-4.71505652523921));
#96112=CARTESIAN_POINT('Ctrl Pts',(14.3662964980548,9.89427046552061,-5.14181677612684));
#96113=CARTESIAN_POINT('Ctrl Pts',(14.3485173441753,9.66600198051707,-5.55598757991483));
#96114=CARTESIAN_POINT('Ctrl Pts',(14.3307812918777,9.41305321993345,-5.95427108959876));
#96115=CARTESIAN_POINT('Ctrl Pts',(14.3129041310352,9.15809199169641,-6.35572335440244));
#96116=CARTESIAN_POINT('Ctrl Pts',(14.29507073134,8.87805625267711,-6.7410357153329));
#96117=CARTESIAN_POINT('Ctrl Pts',(14.2772910900074,8.5748095345901,-7.10681912034434));
#96118=CARTESIAN_POINT('Ctrl Pts',(14.2605178060459,8.28872708682073,-7.45189857419375));
#96119=CARTESIAN_POINT('Ctrl Pts',(14.2437923326192,7.98198635718675,-7.77959808581969));
#96120=CARTESIAN_POINT('Ctrl Pts',(14.227122973847,7.65610933899355,-8.08704727484651));
#96121=CARTESIAN_POINT('Ctrl Pts',(14.2261228517416,7.63655748855957,-8.10549349910998));
#96122=CARTESIAN_POINT('Ctrl Pts',(14.2251229316967,7.61693674075024,-8.12386681794129));
#96123=CARTESIAN_POINT('Ctrl Pts',(14.2241232155377,7.59724741963854,-8.14216660735697));
#96124=CARTESIAN_POINT('Ctrl Pts',(14.2241072450444,7.5969328821891,-8.14245894699912));
#96125=CARTESIAN_POINT('Ctrl Pts',(14.224091274633,7.59661832736125,-8.1427512678872));
#96126=CARTESIAN_POINT('Ctrl Pts',(14.2240753043035,7.59630375515616,-8.14304357001812));
#96127=CARTESIAN_POINT('Ctrl Pts',(14.2131549621309,7.38120261376546,-8.3429166706131));
#96128=CARTESIAN_POINT('Ctrl Pts',(14.2022727831546,7.15797252043843,-8.53402145897874));
#96129=CARTESIAN_POINT('Ctrl Pts',(14.1913844675769,6.9273861129154,-8.71584559113722));
#96130=CARTESIAN_POINT('Ctrl Pts',(14.1804968209202,6.69681387141111,-8.89765855297526));
#96131=CARTESIAN_POINT('Ctrl Pts',(14.1696030234366,6.45888600183346,-9.07019140447614));
#96132=CARTESIAN_POINT('Ctrl Pts',(14.1586596895839,6.21442397422352,-9.23291415592088));
#96133=CARTESIAN_POINT('Ctrl Pts',(14.1512643133734,6.04921941337559,-9.34288027603868));
#96134=CARTESIAN_POINT('Ctrl Pts',(14.1438463206219,5.88103179822744,-9.44836586224379));
#96135=CARTESIAN_POINT('Ctrl Pts',(14.1363927682876,5.71012790879231,-9.54920486720541));
#96136=CARTESIAN_POINT('Ctrl Pts',(14.1216281677088,5.37158763273423,-9.74895494129653));
#96137=CARTESIAN_POINT('Ctrl Pts',(14.1068694552858,5.02262805541314,-9.93091603163188));
#96138=CARTESIAN_POINT('Ctrl Pts',(14.0921174001175,4.66529778493237,-10.0942603848338));
#96139=CARTESIAN_POINT('Ctrl Pts',(14.0773653449492,4.30796751445161,-10.2576047380358));
#96140=CARTESIAN_POINT('Ctrl Pts',(14.0626199458783,3.94226743200403,-10.402335429853));
#96141=CARTESIAN_POINT('Ctrl Pts',(14.0478772200694,3.57014454984236,-10.5276384934889));
#96142=CARTESIAN_POINT('Ctrl Pts',(14.0305614199039,3.13307439415546,-10.6748109253835));
#96143=CARTESIAN_POINT('Ctrl Pts',(14.0132282417536,2.68696134846804,-10.7951794302555));
#96144=CARTESIAN_POINT('Ctrl Pts',(13.9958926142567,2.23521888289641,-10.8873008395147));
#96145=CARTESIAN_POINT('Ctrl Pts',(13.9837106207932,1.91777298924478,-10.9520358717853));
#96146=CARTESIAN_POINT('Ctrl Pts',(13.971527403441,1.59754753804668,-11.0028233533345));
#96147=CARTESIAN_POINT('Ctrl Pts',(13.9593479247777,1.27572652031624,-11.0391779100375));
#96148=CARTESIAN_POINT('Ctrl Pts',(13.9420765290348,0.819360668440139,-11.0907313429248));
#96149=CARTESIAN_POINT('Ctrl Pts',(13.9248126805284,0.359787528436995,-11.113259270819));
#96150=CARTESIAN_POINT('Ctrl Pts',(13.9075699047137,-0.0993101696415865,
-11.1072933181119));
#96151=CARTESIAN_POINT('Ctrl Pts',(13.8953468761735,-0.424754536992514,
-11.1030641840679));
#96152=CARTESIAN_POINT('Ctrl Pts',(13.8831344205217,-0.749960265695552,
-11.084517719827));
#96153=CARTESIAN_POINT('Ctrl Pts',(13.8709371529732,-1.07362401428721,-11.0518567173184));
#96154=CARTESIAN_POINT('Ctrl Pts',(13.8562299511789,-1.46389077240429,-11.0124747858498));
#96155=CARTESIAN_POINT('Ctrl Pts',(13.8415141838714,-1.8521538137257,-10.9524664405571));
#96156=CARTESIAN_POINT('Ctrl Pts',(13.8267936423669,-2.23612309892015,-10.8721120054768));
#96157=CARTESIAN_POINT('Ctrl Pts',(13.8074272722069,-2.7412737623547,-10.7663975700887));
#96158=CARTESIAN_POINT('Ctrl Pts',(13.7880526528729,-3.23899168788081,-10.6254662692622));
#96159=CARTESIAN_POINT('Ctrl Pts',(13.7686781120946,-3.72446110312998,-10.4509094002611));
#96160=CARTESIAN_POINT('Ctrl Pts',(13.7492251037983,-4.21189668524437,-10.2756455702834));
#96161=CARTESIAN_POINT('Ctrl Pts',(13.7297721758329,-4.68698327940954,-10.0664838182762));
#96162=CARTESIAN_POINT('Ctrl Pts',(13.7103273747444,-5.14486845773911,-9.82508158909665));
#96163=CARTESIAN_POINT('Ctrl Pts',(13.7050057894525,-5.27018087514552,-9.75901546960325));
#96164=CARTESIAN_POINT('Ctrl Pts',(13.6996848106097,-5.39420510479515,-9.69053481749199));
#96165=CARTESIAN_POINT('Ctrl Pts',(13.6943645980911,-5.51684212818613,-9.61967412727097));
#96166=CARTESIAN_POINT('Ctrl Pts',(13.6943603323047,-5.51694045947439,-9.61961731063629));
#96167=CARTESIAN_POINT('Ctrl Pts',(13.6943560665187,-5.51703878987083,-9.61956049247151));
#96168=CARTESIAN_POINT('Ctrl Pts',(13.6943518007333,-5.51713711937541,-9.61950367277666));
#96169=CARTESIAN_POINT('Ctrl Pts',(13.672318355336,-6.02502430590092,-9.32602111045481));
#96170=CARTESIAN_POINT('Ctrl Pts',(13.650294336554,-6.50906190953783,-8.99172904315948));
#96171=CARTESIAN_POINT('Ctrl Pts',(13.6282771905346,-6.96384305218222,-8.62166957247464));
#96172=CARTESIAN_POINT('Ctrl Pts',(13.6058802342115,-7.42646946976525,-8.24522633162227));
#96173=CARTESIAN_POINT('Ctrl Pts',(13.5834903898995,-7.85882243931573,-7.83177022822399));
#96174=CARTESIAN_POINT('Ctrl Pts',(13.5611049469218,-8.25518594461479,-7.38656161626531));
#96175=CARTESIAN_POINT('Ctrl Pts',(13.5467276107356,-8.50975545986931,-7.10062070844145));
#96176=CARTESIAN_POINT('Ctrl Pts',(13.5323520896496,-8.74947872840078,-6.80158092168345));
#96177=CARTESIAN_POINT('Ctrl Pts',(13.5179776605464,-8.97283292601846,-6.49082829953906));
#96178=CARTESIAN_POINT('Ctrl Pts',(13.5179763595475,-8.97285314133025,-6.49080017398237));
#96179=CARTESIAN_POINT('Ctrl Pts',(13.5179750585485,-8.9728733565079,-6.49077204832963));
#96180=CARTESIAN_POINT('Ctrl Pts',(13.5179737575496,-8.97289357155134,-6.49074392258092));
#96181=CARTESIAN_POINT('Ctrl Pts',(13.4921480292973,-9.37417615952936,-5.93242836588278));
#96182=CARTESIAN_POINT('Ctrl Pts',(13.4663166539886,-9.7225828106941,-5.33627768736209));
#96183=CARTESIAN_POINT('Ctrl Pts',(13.440491435221,-10.0132972689579,-4.71338935698886));
#96184=CARTESIAN_POINT('Ctrl Pts',(13.4143413439915,-10.3076688161562,-4.08266530343198));
#96185=CARTESIAN_POINT('Ctrl Pts',(13.3881975686009,-10.5428877259154,-3.42452840408841));
#96186=CARTESIAN_POINT('Ctrl Pts',(13.3620711711185,-10.7140055390992,-2.75049821329857));
#96187=CARTESIAN_POINT('Ctrl Pts',(13.3553005411707,-10.7583505503597,-2.57582395908512));
#96188=CARTESIAN_POINT('Ctrl Pts',(13.3485310720448,-10.7983909050603,-2.40008225456296));
#96189=CARTESIAN_POINT('Ctrl Pts',(13.34176294332,-10.8340410075211,-2.22347335356751));
#96190=CARTESIAN_POINT('Ctrl Pts',(13.3417607609311,-10.8340525029272,-2.22341640587578));
#96191=CARTESIAN_POINT('Ctrl Pts',(13.3417585785423,-10.8340639978769,-2.22335945809389));
#96192=CARTESIAN_POINT('Ctrl Pts',(13.3417563961537,-10.8340754923701,-2.22330251022183));
#96193=CARTESIAN_POINT('Ctrl Pts',(13.3105788808085,-10.9982853547507,-1.40974752574804));
#96194=CARTESIAN_POINT('Ctrl Pts',(13.2794222220121,-11.069299590073,-0.577797912359255));
#96195=CARTESIAN_POINT('Ctrl Pts',(13.2482776981295,-11.0476511917255,0.251461408095067));
#96196=CARTESIAN_POINT('Ctrl Pts',(13.2208054288712,-11.0285553586777,0.982942660542084));
#96197=CARTESIAN_POINT('Ctrl Pts',(13.1933426162945,-10.937358983901,1.71233147641963));
#96198=CARTESIAN_POINT('Ctrl Pts',(13.1658839303791,-10.7743974792278,2.42514198951792));
#96199=CARTESIAN_POINT('Ctrl Pts',(13.1658821827909,-10.7743871076607,2.42518735582724));
#96200=CARTESIAN_POINT('Ctrl Pts',(13.1658804352027,-10.774376735803,2.42523272206939));
#96201=CARTESIAN_POINT('Ctrl Pts',(13.1658786876146,-10.7743663636545,2.42527808824439));
#96202=CARTESIAN_POINT('Ctrl Pts',(13.1280368516429,-10.5497704613986,3.40762586902646));
#96203=CARTESIAN_POINT('Ctrl Pts',(13.0902086077735,-10.1888936274173,4.35849696440613));
#96204=CARTESIAN_POINT('Ctrl Pts',(13.0523973489158,-9.70795439135571,5.24321458223078));
#96205=CARTESIAN_POINT('Ctrl Pts',(13.0316692936244,-9.4443044791854,5.72821498299888));
#96206=CARTESIAN_POINT('Ctrl Pts',(13.0109463370872,-9.14457426237966,6.19333505790884));
#96207=CARTESIAN_POINT('Ctrl Pts',(12.9902289974229,-8.81144133675073,6.63286537247014));
#96208=CARTESIAN_POINT('Ctrl Pts',(12.9902260976388,-8.81139470848843,6.63292689306214));
#96209=CARTESIAN_POINT('Ctrl Pts',(12.9902231978549,-8.81134807957172,6.63298841315281));
#96210=CARTESIAN_POINT('Ctrl Pts',(12.990220298071,-8.81130145000063,6.63304993274213));
#96211=CARTESIAN_POINT('Ctrl Pts',(12.9380037558956,-7.9716405999951,7.74083603199739));
#96212=CARTESIAN_POINT('Ctrl Pts',(12.8858195375993,-6.91977593055457,8.68604892505739));
#96213=CARTESIAN_POINT('Ctrl Pts',(12.8336661371426,-5.73205062687898,9.40563273683172));
#96214=CARTESIAN_POINT('Ctrl Pts',(12.8273800139828,-5.58889241526566,9.49236519195473));
#96215=CARTESIAN_POINT('Ctrl Pts',(12.8210943397431,-5.44376046343101,9.57581980868288));
#96216=CARTESIAN_POINT('Ctrl Pts',(12.8148091127809,-5.29678846581114,9.65588622909681));
#96217=CARTESIAN_POINT('Ctrl Pts',(12.8148074440706,-5.2967494451542,9.65590748650893));
#96218=CARTESIAN_POINT('Ctrl Pts',(12.8148057753604,-5.29671042436758,9.65592874368221));
#96219=CARTESIAN_POINT('Ctrl Pts',(12.8148041066501,-5.29667140345124,9.65595000061667));
#96220=CARTESIAN_POINT('Ctrl Pts',(12.7795911172689,-4.47325515726357,10.104512126223));
#96221=CARTESIAN_POINT('Ctrl Pts',(12.7443897733396,-3.59207956867088,10.4467162251273));
#96222=CARTESIAN_POINT('Ctrl Pts',(12.7092021403706,-2.68282119992599,10.6728297518592));
#96223=CARTESIAN_POINT('Ctrl Pts',(12.6859989915403,-2.08324528432376,10.8219317337387));
#96224=CARTESIAN_POINT('Ctrl Pts',(12.6628017875576,-1.47145724776612,10.9205542219341));
#96225=CARTESIAN_POINT('Ctrl Pts',(12.6396109205276,-0.855959330699359,
10.9658962051474));
#96226=CARTESIAN_POINT('Ctrl Pts',(12.639608461027,-0.855894054248407,10.9659010138781));
#96227=CARTESIAN_POINT('Ctrl Pts',(12.6396060015265,-0.855828777755838,
10.9659058220097));
#96228=CARTESIAN_POINT('Ctrl Pts',(12.6396035420261,-0.855763501221594,
10.9659106295421));
#96229=CARTESIAN_POINT('Ctrl Pts',(12.600852474588,0.172711781201659,11.0416565048728));
#96230=CARTESIAN_POINT('Ctrl Pts',(12.5621242554643,1.21152764921655,10.9686607859318));
#96231=CARTESIAN_POINT('Ctrl Pts',(12.523415689347,2.22066350476061,10.7565359105041));
#96232=CARTESIAN_POINT('Ctrl Pts',(12.4839776371738,3.24881712843266,10.5404134150604));
#96233=CARTESIAN_POINT('Ctrl Pts',(12.4445599840427,4.24615952376666,10.1798673325154));
#96234=CARTESIAN_POINT('Ctrl Pts',(12.4051604950114,5.17033547788135,9.68510657471025));
#96235=CARTESIAN_POINT('Ctrl Pts',(12.3958748650144,5.38814429147203,9.56850188142757));
#96236=CARTESIAN_POINT('Ctrl Pts',(12.3865902489369,5.60188906417856,9.44444251544705));
#96237=CARTESIAN_POINT('Ctrl Pts',(12.3773066267887,5.81101532521251,9.3130625511924));
#96238=CARTESIAN_POINT('Ctrl Pts',(12.3773065522333,5.81101700467344,9.31306149610005));
#96239=CARTESIAN_POINT('Ctrl Pts',(12.377306477678,5.81101868413409,9.31306044100723));
#96240=CARTESIAN_POINT('Ctrl Pts',(12.3773064031226,5.81102036359442,9.31305938591394));
#96241=CARTESIAN_POINT('Ctrl Pts',(12.3241086670831,7.00937155969095,8.56021498805325));
#96242=CARTESIAN_POINT('Ctrl Pts',(12.2709407504699,8.05609808609067,7.56696251764249));
#96243=CARTESIAN_POINT('Ctrl Pts',(12.2178065051586,8.8827252865088,6.41753671029591));
#96244=CARTESIAN_POINT('Ctrl Pts',(12.1837058825503,9.4132400615682,5.67985547584888));
#96245=CARTESIAN_POINT('Ctrl Pts',(12.1496190936948,9.85310033145007,4.87784795278562));
#96246=CARTESIAN_POINT('Ctrl Pts',(12.1155467762475,10.1842082928,4.03376973742849));
#96247=CARTESIAN_POINT('Ctrl Pts',(12.1155465571978,10.1842104214813,4.03376431087971));
#96248=CARTESIAN_POINT('Ctrl Pts',(12.1155463381481,10.1842125501581,4.03375888432918));
#96249=CARTESIAN_POINT('Ctrl Pts',(12.1155461190984,10.1842146788304,4.03375345777692));
#96250=CARTESIAN_POINT('Ctrl Pts',(12.0549794961925,10.7727865153168,2.53332719255639));
#96251=CARTESIAN_POINT('Ctrl Pts',(11.9944605437619,11.0177216674262,0.899991790145014));
#96252=CARTESIAN_POINT('Ctrl Pts',(11.9339855927979,10.9113240835915,-0.707007078692226));
#96253=CARTESIAN_POINT('Ctrl Pts',(11.9074297722812,10.8646026709291,-1.41267401766815));
#96254=CARTESIAN_POINT('Ctrl Pts',(11.8808824625675,10.7501342130751,-2.11326202676983));
#96255=CARTESIAN_POINT('Ctrl Pts',(11.8543434757932,10.5672658927243,-2.79528406953566));
#96256=CARTESIAN_POINT('Ctrl Pts',(11.8543434226523,10.5672655265544,-2.79528543519573));
#96257=CARTESIAN_POINT('Ctrl Pts',(11.8543433695114,10.5672651603842,-2.79528680085578));
#96258=CARTESIAN_POINT('Ctrl Pts',(11.8543433163706,10.5672647942137,-2.7952881665157));
#96259=CARTESIAN_POINT('Ctrl Pts',(11.7800575547027,10.0553939777664,-4.70434829349969));
#96260=CARTESIAN_POINT('Ctrl Pts',(11.7058378548569,9.00761473780677,-6.46795760223549));
#96261=CARTESIAN_POINT('Ctrl Pts',(11.6316861718067,7.58770537091745,-7.83892251958424));
#96262=CARTESIAN_POINT('Ctrl Pts',(11.6190193009064,7.34515108353452,-8.07311593101516));
#96263=CARTESIAN_POINT('Ctrl Pts',(11.606354412188,7.09173782638425,-8.29585177971521));
#96264=CARTESIAN_POINT('Ctrl Pts',(11.5936915121807,6.82828205311893,-8.5058980015901));
#96265=CARTESIAN_POINT('Ctrl Pts',(11.5936913931372,6.82827957638059,-8.50589997622716));
#96266=CARTESIAN_POINT('Ctrl Pts',(11.5936912740938,6.82827709964131,-8.50590195086313));
#96267=CARTESIAN_POINT('Ctrl Pts',(11.5936911550503,6.82827462290119,-8.50590392549794));
#96268=CARTESIAN_POINT('Ctrl Pts',(11.5068997264266,5.0225492848719,-9.94555763904382));
#96269=CARTESIAN_POINT('Ctrl Pts',(11.4202013141422,2.74505378677467,-10.7890813085325));
#96270=CARTESIAN_POINT('Ctrl Pts',(11.3335954869663,0.442386430243757,-10.8750546437055));
#96271=CARTESIAN_POINT('Ctrl Pts',(11.3335954593555,0.442385696129285,-10.8750546711147));
#96272=CARTESIAN_POINT('Ctrl Pts',(11.3335954317446,0.442384962014812,-10.8750546985239));
#96273=CARTESIAN_POINT('Ctrl Pts',(11.3335954041338,0.442384227900335,-10.8750547259329));
#96274=CARTESIAN_POINT('Ctrl Pts',(11.2469895821273,-1.86028300880753,-10.9610275730008));
#96275=CARTESIAN_POINT('Ctrl Pts',(11.1604765226659,-4.18812205175047,-10.2894500642299));
#96276=CARTESIAN_POINT('Ctrl Pts',(11.0740563207977,-6.0881731640799,-8.99381874970801));
#96277=CARTESIAN_POINT('Ctrl Pts',(11.0740562881466,-6.08817388195301,-8.99381826019546));
#96278=CARTESIAN_POINT('Ctrl Pts',(11.0740562554955,-6.08817459982607,-8.9938177706828));
#96279=CARTESIAN_POINT('Ctrl Pts',(11.0740562228444,-6.08817531769906,-8.99381728117006));
#96280=CARTESIAN_POINT('Ctrl Pts',(10.9876360070261,-7.98822641502771,-7.69818528489756));
#96281=CARTESIAN_POINT('Ctrl Pts',(10.9013086316892,-9.46049010855842,-5.77850039221671));
#96282=CARTESIAN_POINT('Ctrl Pts',(10.8150741171685,-10.2174550760751,-3.6130677051965));
#96283=CARTESIAN_POINT('Ctrl Pts',(10.8150740985777,-10.217455239265,-3.61306723836286));
#96284=CARTESIAN_POINT('Ctrl Pts',(10.8150740799868,-10.2174554024549,-3.61306677152912));
#96285=CARTESIAN_POINT('Ctrl Pts',(10.815074061396,-10.2174555656447,-3.61306630469546));
#96286=CARTESIAN_POINT('Ctrl Pts',(10.7288395283245,-10.9744203879367,-1.44763304488258));
#96287=CARTESIAN_POINT('Ctrl Pts',(10.64269786965,-11.0160857164996,0.963547943719072));
#96288=CARTESIAN_POINT('Ctrl Pts',(10.5566490107872,-10.3432575454559,3.15272781414372));
#96289=CARTESIAN_POINT('Ctrl Pts',(10.4992831048788,-9.89470543142672,4.61218106109354));
#96290=CARTESIAN_POINT('Ctrl Pts',(10.4419584574757,-9.12860066636951,5.97296717125667));
#96291=CARTESIAN_POINT('Ctrl Pts',(10.3846748536244,-8.11866041143882,7.11645359126049));
#96292=CARTESIAN_POINT('Ctrl Pts',(10.3273912859189,-7.10872079377668,8.25993928972863));
#96293=CARTESIAN_POINT('Ctrl Pts',(10.270148710313,-5.85494574612279,9.18612541739735));
#96294=CARTESIAN_POINT('Ctrl Pts',(10.212947625229,-4.46736999604014,9.81217383299535));
#96295=CARTESIAN_POINT('Ctrl Pts',(10.2129475891353,-4.4673691204844,9.81217422802984));
#96296=CARTESIAN_POINT('Ctrl Pts',(10.2129475530416,-4.46736824492864,9.8121746230642));
#96297=CARTESIAN_POINT('Ctrl Pts',(10.2129475169479,-4.46736736937278,9.81217501809846));
#96298=CARTESIAN_POINT('Ctrl Pts',(10.1557463958226,-3.07979057487988,10.4382234499593));
#96299=CARTESIAN_POINT('Ctrl Pts',(10.0985865820643,-1.55841352331276,10.764137510334));
#96300=CARTESIAN_POINT('Ctrl Pts',(10.0414676010471,-0.0371553896940832,
10.7643933921731));
#96301=CARTESIAN_POINT('Ctrl Pts',(10.0414675736428,-0.0371546598294985,
10.7643933922959));
#96302=CARTESIAN_POINT('Ctrl Pts',(10.0414675462384,-0.0371539299649098,
10.7643933924186));
#96303=CARTESIAN_POINT('Ctrl Pts',(10.041467518834,-0.0371532001003252,
10.7643933925412));
#96304=CARTESIAN_POINT('Ctrl Pts',(9.9843485652607,1.48410420353549,10.7646489617688));
#96305=CARTESIAN_POINT('Ctrl Pts',(9.92727075752572,3.00523791058294,10.4392434588977));
#96306=CARTESIAN_POINT('Ctrl Pts',(9.87023419783678,4.38858771822708,9.81420125308147));
#96307=CARTESIAN_POINT('Ctrl Pts',(9.87023410346677,4.38859000705254,9.81420021891607));
#96308=CARTESIAN_POINT('Ctrl Pts',(9.87023400909677,4.3885922958776,9.81419918474985));
#96309=CARTESIAN_POINT('Ctrl Pts',(9.87023391472676,4.3885945847023,9.81419815058281));
#96310=CARTESIAN_POINT('Ctrl Pts',(9.81492195756586,5.73011589466252,9.20805425213235));
#96311=CARTESIAN_POINT('Ctrl Pts',(9.75965008730089,6.94206068657357,8.32010181699716));
#96312=CARTESIAN_POINT('Ctrl Pts',(9.70441539209234,7.9310140168344,7.23174142669155));
#96313=CARTESIAN_POINT('Ctrl Pts',(9.68370762696688,8.30177759588128,6.82370964070612));
#96314=CARTESIAN_POINT('Ctrl Pts',(9.66300506861179,8.64119941133731,6.38750964268081));
#96315=CARTESIAN_POINT('Ctrl Pts',(9.6423074979077,8.94435870693281,5.92742985065327));
#96316=CARTESIAN_POINT('Ctrl Pts',(9.64230720657879,8.94436297405523,5.92742337479446));
#96317=CARTESIAN_POINT('Ctrl Pts',(9.64230691524988,8.94436724117044,5.92741689893095));
#96318=CARTESIAN_POINT('Ctrl Pts',(9.64230662392097,8.94437150827848,5.92741042306268));
#96319=CARTESIAN_POINT('Ctrl Pts',(9.60435433150811,9.50026049356103,5.08377960741856));
#96320=CARTESIAN_POINT('Ctrl Pts',(9.56642190939225,9.9342040024153,4.159855444481));
#96321=CARTESIAN_POINT('Ctrl Pts',(9.5285088642955,10.2309211646493,3.19456526247108));
#96322=CARTESIAN_POINT('Ctrl Pts',(9.52850829697134,10.2309256046729,3.19455081803803));
#96323=CARTESIAN_POINT('Ctrl Pts',(9.52850772964719,10.2309300446658,3.1945363735957));
#96324=CARTESIAN_POINT('Ctrl Pts',(9.52850716232304,10.2309344846279,3.19452192914411));
#96325=CARTESIAN_POINT('Ctrl Pts',(9.49751616091674,10.4734746138266,2.4054703449874));
#96326=CARTESIAN_POINT('Ctrl Pts',(9.46653980188838,10.6243054333359,1.58876224559805));
#96327=CARTESIAN_POINT('Ctrl Pts',(9.43557487104774,10.6810137934708,0.766165713708518));
#96328=CARTESIAN_POINT('Ctrl Pts',(9.40971907541639,10.7283654177255,0.0792955273978293));
#96329=CARTESIAN_POINT('Ctrl Pts',(9.38387122529526,10.7100934152529,-0.611679955836055));
#96330=CARTESIAN_POINT('Ctrl Pts',(9.3580287865665,10.6248148432736,-1.29410491435847));
#96331=CARTESIAN_POINT('Ctrl Pts',(9.35802791788757,10.6248119766827,-1.29412785368672));
#96332=CARTESIAN_POINT('Ctrl Pts',(9.35802704920864,10.6248091100161,-1.29415079300532));
#96333=CARTESIAN_POINT('Ctrl Pts',(9.35802618052972,10.6248062432738,-1.29417373231425));
#96334=CARTESIAN_POINT('Ctrl Pts',(9.33136117227495,10.5368085895391,-1.99831981820764));
#96335=CARTESIAN_POINT('Ctrl Pts',(9.30470642071757,10.3774519767225,-2.69334920017192));
#96336=CARTESIAN_POINT('Ctrl Pts',(9.27806101664121,10.1517039759143,-3.3660344562145));
#96337=CARTESIAN_POINT('Ctrl Pts',(9.25166522032462,9.92807072827676,-4.0324181579887));
#96338=CARTESIAN_POINT('Ctrl Pts',(9.22527859740385,9.63928326821499,-4.67687583326026));
#96339=CARTESIAN_POINT('Ctrl Pts',(9.1989005456505,9.29012867331838,-5.28652206468518));
#96340=CARTESIAN_POINT('Ctrl Pts',(9.19519318643189,9.24105600039261,-5.37220608704211));
#96341=CARTESIAN_POINT('Ctrl Pts',(9.19148599698024,9.19079080927959,-5.45720239902285));
#96342=CARTESIAN_POINT('Ctrl Pts',(9.18777897607309,9.13934633775977,-5.54147516031589));
#96343=CARTESIAN_POINT('Ctrl Pts',(9.18777862752297,9.13934150072836,-5.54148308400489));
#96344=CARTESIAN_POINT('Ctrl Pts',(9.18777827897285,9.13933666368652,-5.54149100768753));
#96345=CARTESIAN_POINT('Ctrl Pts',(9.18777793042273,9.13933182663427,-5.54149893136375));
#96346=CARTESIAN_POINT('Ctrl Pts',(9.16595156155315,8.83643338769895,-6.03768318532182));
#96347=CARTESIAN_POINT('Ctrl Pts',(9.14412404033658,8.49268493443823,-6.5088028215877));
#96348=CARTESIAN_POINT('Ctrl Pts',(9.12230283605917,8.11333699133592,-6.94895344648578));
#96349=CARTESIAN_POINT('Ctrl Pts',(9.1007799800376,7.73917564544167,-7.38308615552656));
#96350=CARTESIAN_POINT('Ctrl Pts',(9.07926327119728,7.33038224266112,-7.78708966817594));
#96351=CARTESIAN_POINT('Ctrl Pts',(9.05776052154422,6.8920401299936,-8.15531820550438));
#96352=CARTESIAN_POINT('Ctrl Pts',(9.04442758288083,6.62024286703547,-8.38364102846997));
#96353=CARTESIAN_POINT('Ctrl Pts',(9.03110002353198,6.33708584074756,-8.59820985818628));
#96354=CARTESIAN_POINT('Ctrl Pts',(9.01777983194417,6.04378813771145,-8.79768591775239));
#96355=CARTESIAN_POINT('Ctrl Pts',(9.01777534574994,6.04368935606449,-8.79775310059593));
#96356=CARTESIAN_POINT('Ctrl Pts',(9.01777085955654,6.04359057326732,-8.79782028172752));
#96357=CARTESIAN_POINT('Ctrl Pts',(9.01776637336399,6.04349178931997,-8.79788746114716));
#96358=CARTESIAN_POINT('Ctrl Pts',(8.99835752642122,5.61611768741423,-9.08852925980856));
#96359=CARTESIAN_POINT('Ctrl Pts',(8.97897750190263,5.16711889953788,-9.34709581950139));
#96360=CARTESIAN_POINT('Ctrl Pts',(8.95961099581836,4.70183043817049,-9.57208606414997));
#96361=CARTESIAN_POINT('Ctrl Pts',(8.94010759386849,4.23325299600327,-9.79866669552901));
#96362=CARTESIAN_POINT('Ctrl Pts',(8.92061791695976,3.74815476838732,-9.99119583465263));
#96363=CARTESIAN_POINT('Ctrl Pts',(8.90112442847188,3.25193223126937,-10.1481415373154));
#96364=CARTESIAN_POINT('Ctrl Pts',(8.88176502595483,2.75912296113442,-10.3040076888798));
#96365=CARTESIAN_POINT('Ctrl Pts',(8.86240184781724,2.25534145763491,-10.4247794736471));
#96366=CARTESIAN_POINT('Ctrl Pts',(8.84301586321307,1.74582552457155,-10.5089394452822));
#96367=CARTESIAN_POINT('Ctrl Pts',(8.82424818602389,1.25256037710942,-10.5904151718006));
#96368=CARTESIAN_POINT('Ctrl Pts',(8.80545909132578,0.75391995921181,-10.6375782823634));
#96369=CARTESIAN_POINT('Ctrl Pts',(8.78663001960709,0.254620932449703,-10.6490198881749));
#96370=CARTESIAN_POINT('Ctrl Pts',(8.77889317541281,0.0494595291618394,
-10.6537212310143));
#96371=CARTESIAN_POINT('Ctrl Pts',(8.77114956980311,-0.155813432184366,
-10.6523909638077));
#96372=CARTESIAN_POINT('Ctrl Pts',(8.76339787861685,-0.360872045124682,
-10.6449290957503));
#96373=CARTESIAN_POINT('Ctrl Pts',(8.76339639289417,-0.360911347546018,
-10.6449276655764));
#96374=CARTESIAN_POINT('Ctrl Pts',(8.76339490717174,-0.360950649958548,
-10.6449262351748));
#96375=CARTESIAN_POINT('Ctrl Pts',(8.76339342144957,-0.360989952362255,
-10.6449248045455));
#96376=CARTESIAN_POINT('Ctrl Pts',(8.7472112451467,-0.789063545175176,-10.6293426885334));
#96377=CARTESIAN_POINT('Ctrl Pts',(8.73105993269548,-1.21608690026484,-10.5867478851266));
#96378=CARTESIAN_POINT('Ctrl Pts',(8.71493237946594,-1.6389963910984,-10.5183805109206));
#96379=CARTESIAN_POINT('Ctrl Pts',(8.69877732719559,-2.06262698358809,-10.4498965637177));
#96380=CARTESIAN_POINT('Ctrl Pts',(8.68264613405947,-2.48212897303565,-10.3555528793687));
#96381=CARTESIAN_POINT('Ctrl Pts',(8.66653095761318,-2.89445997262348,-10.2366322226155));
#96382=CARTESIAN_POINT('Ctrl Pts',(8.65637934997417,-3.1542041050669,-10.1617192453015));
#96383=CARTESIAN_POINT('Ctrl Pts',(8.64623408231994,-3.41110338803429,-10.0770541792883));
#96384=CARTESIAN_POINT('Ctrl Pts',(8.63609301378944,-3.66440656040103,-9.98296294023557));
#96385=CARTESIAN_POINT('Ctrl Pts',(8.61999121628629,-4.06659656395806,-9.83356664402763));
#96386=CARTESIAN_POINT('Ctrl Pts',(8.60389650957975,-4.45980978303877,-9.66037870828455));
#96387=CARTESIAN_POINT('Ctrl Pts',(8.58781889640342,-4.8411520976406,-9.46449648788158));
#96388=CARTESIAN_POINT('Ctrl Pts',(8.57193722196419,-5.21784697293012,-9.27100149464125));
#96389=CARTESIAN_POINT('Ctrl Pts',(8.55607221493741,-5.58295902660875,-9.05536112634003));
#96390=CARTESIAN_POINT('Ctrl Pts',(8.54023467305762,-5.93365513709574,-8.81860803880677));
#96391=CARTESIAN_POINT('Ctrl Pts',(8.52997407019511,-6.16085917812977,-8.66522379356907));
#96392=CARTESIAN_POINT('Ctrl Pts',(8.51972501786341,-6.38201150082015,-8.50297743261047));
#96393=CARTESIAN_POINT('Ctrl Pts',(8.50949077051101,-6.596330404719,-8.33214655552495));
#96394=CARTESIAN_POINT('Ctrl Pts',(8.50947347554573,-6.59669258455251,-8.33185786657827));
#96395=CARTESIAN_POINT('Ctrl Pts',(8.50945618061979,-6.59705474487907,-8.33156915312288));
#96396=CARTESIAN_POINT('Ctrl Pts',(8.50943888573315,-6.59741688569491,-8.3312804151605));
#96397=CARTESIAN_POINT('Ctrl Pts',(8.49562499333087,-6.88666852213946,-8.10065761742697));
#96398=CARTESIAN_POINT('Ctrl Pts',(8.4818363825045,-7.16346871481822,-7.854401200835));
#96399=CARTESIAN_POINT('Ctrl Pts',(8.46804513914204,-7.42663655013192,-7.59427885300374));
#96400=CARTESIAN_POINT('Ctrl Pts',(8.45397426302108,-7.69514040525225,-7.32888223600308));
#96401=CARTESIAN_POINT('Ctrl Pts',(8.43990064456776,-7.94945379603481,-7.04905274715913));
#96402=CARTESIAN_POINT('Ctrl Pts',(8.42579182381223,-8.18837355310747,-6.75664594045687));
#96403=CARTESIAN_POINT('Ctrl Pts',(8.41168300305669,-8.42729331018012,-6.46423913375461));
#96404=CARTESIAN_POINT('Ctrl Pts',(8.39753889189418,-8.65082004612712,-6.15925583448179));
#96405=CARTESIAN_POINT('Ctrl Pts',(8.3833249342102,-8.85779381202089,-5.84351584079338));
#96406=CARTESIAN_POINT('Ctrl Pts',(8.38332138896566,-8.85784543540609,-5.84343708894168));
#96407=CARTESIAN_POINT('Ctrl Pts',(8.38331784371677,-8.85789705776173,-5.84335833642056));
#96408=CARTESIAN_POINT('Ctrl Pts',(8.38331429846353,-8.85794867908778,-5.84327958323009));
#96409=CARTESIAN_POINT('Ctrl Pts',(8.37051523834771,-9.04431179920568,-5.55896510664368));
#96410=CARTESIAN_POINT('Ctrl Pts',(8.35766296116299,-9.21721824714137,-5.26597631159482));
#96411=CARTESIAN_POINT('Ctrl Pts',(8.34479347421291,-9.37579863677535,-4.96559013941187));
#96412=CARTESIAN_POINT('Ctrl Pts',(8.33191202528665,-9.53452642426984,-4.66492476322892));
#96413=CARTESIAN_POINT('Ctrl Pts',(8.31901338599653,-9.67890075224488,-4.35684781344631));
#96414=CARTESIAN_POINT('Ctrl Pts',(8.30613513665175,-9.80802233333987,-4.04268415445901));
#96415=CARTESIAN_POINT('Ctrl Pts',(8.29328204869782,-9.93689163802027,-3.72913430519128));
#96416=CARTESIAN_POINT('Ctrl Pts',(8.28044923194413,-10.0505668707882,-3.40952124130343));
#96417=CARTESIAN_POINT('Ctrl Pts',(8.26767542199453,-10.1481388416316,-3.08521150397574));
#96418=CARTESIAN_POINT('Ctrl Pts',(8.26369649813215,-10.1785316096953,-2.98419201505693));
#96419=CARTESIAN_POINT('Ctrl Pts',(8.25972331273786,-10.2073618763737,-2.88271720020414));
#96420=CARTESIAN_POINT('Ctrl Pts',(8.25575708057026,-10.2346020753326,-2.78082939218218));
#96421=CARTESIAN_POINT('Ctrl Pts',(8.25575524159449,-10.2346147054722,-2.78078215107212));
#96422=CARTESIAN_POINT('Ctrl Pts',(8.25575340262021,-10.23462733527,-2.78073490987328));
#96423=CARTESIAN_POINT('Ctrl Pts',(8.25575156364743,-10.2346399647259,-2.78068766858567));
#96424=CARTESIAN_POINT('Ctrl Pts',(8.23893975591997,-10.3500978914959,-2.3488099092274));
#96425=CARTESIAN_POINT('Ctrl Pts',(8.22213948265902,-10.4374195792317,-1.90951906036571));
#96426=CARTESIAN_POINT('Ctrl Pts',(8.20536583923801,-10.4967246634927,-1.4663631741822));
#96427=CARTESIAN_POINT('Ctrl Pts',(8.18866213713668,-10.5557824624291,-1.02505512193209));
#96428=CARTESIAN_POINT('Ctrl Pts',(8.17198481832912,-10.587056050329,-0.579913295276316));
#96429=CARTESIAN_POINT('Ctrl Pts',(8.15535026019998,-10.5906237611432,-0.134473438999874));
#96430=CARTESIAN_POINT('Ctrl Pts',(8.14675394429533,-10.5924674632107,0.0957185319170201));
#96431=CARTESIAN_POINT('Ctrl Pts',(8.13816907393653,-10.5869115670197,0.325989486190348));
#96432=CARTESIAN_POINT('Ctrl Pts',(8.12959810751433,-10.5739637046953,0.555846992221927));
#96433=CARTESIAN_POINT('Ctrl Pts',(8.11399970135177,-10.5503997323819,0.974167466480529));
#96434=CARTESIAN_POINT('Ctrl Pts',(8.09840440902365,-10.502506383742,1.39112198332939));
#96435=CARTESIAN_POINT('Ctrl Pts',(8.08278120579911,-10.4305106422116,1.80368115067515));
#96436=CARTESIAN_POINT('Ctrl Pts',(8.06723453277086,-10.3588675715229,2.21421939864826));
#96437=CARTESIAN_POINT('Ctrl Pts',(8.0516601675866,-10.2633587199306,2.62040500791612));
#96438=CARTESIAN_POINT('Ctrl Pts',(8.03602523301925,-10.1442192815926,3.01930278573934));
#96439=CARTESIAN_POINT('Ctrl Pts',(8.02525642685694,-10.0621601266776,3.29404988042343));
#96440=CARTESIAN_POINT('Ctrl Pts',(8.01445883116972,-9.96889090332492,3.56534070631904));
#96441=CARTESIAN_POINT('Ctrl Pts',(8.00362135560029,-9.86448776295425,3.83223060469584));
#96442=CARTESIAN_POINT('Ctrl Pts',(8.00361847717217,-9.86446003353207,3.83230149052017));
#96443=CARTESIAN_POINT('Ctrl Pts',(8.00361559874135,-9.86443230332504,3.83237237603219));
#96444=CARTESIAN_POINT('Ctrl Pts',(8.00361272030785,-9.86440457233314,3.8324432612319));
#96445=CARTESIAN_POINT('Ctrl Pts',(7.99175489825204,-9.75016564112609,4.12445767902653));
#96446=CARTESIAN_POINT('Ctrl Pts',(7.97985127327469,-9.6226052671416,4.41117579171117));
#96447=CARTESIAN_POINT('Ctrl Pts',(7.96794656006958,-9.48241448953288,4.69158072901337));
#96448=CARTESIAN_POINT('Ctrl Pts',(7.9560368093057,-9.34216438926174,4.97210432153467));
#96449=CARTESIAN_POINT('Ctrl Pts',(7.94412597831665,-9.18927254031056,5.24630895141322));
#96450=CARTESIAN_POINT('Ctrl Pts',(7.93226013853909,-9.02445980303907,5.51313322716271));
#96451=CARTESIAN_POINT('Ctrl Pts',(7.92772634728073,-8.96148688569672,5.61508349714716));
#96452=CARTESIAN_POINT('Ctrl Pts',(7.9231991379743,-8.89677397751238,5.71595588881535));
#96453=CARTESIAN_POINT('Ctrl Pts',(7.91868114386462,-8.83036269920675,5.81568976264978));
#96454=CARTESIAN_POINT('Ctrl Pts',(7.90363802990147,-8.6092396955607,6.14776368608839));
#96455=CARTESIAN_POINT('Ctrl Pts',(7.88863551605419,-8.36946664710543,6.467329519687));
#96456=CARTESIAN_POINT('Ctrl Pts',(7.87366135061745,-8.1127219252988,6.77251705231258));
#96457=CARTESIAN_POINT('Ctrl Pts',(7.86059975399369,-7.8887698121954,7.03872463914581));
#96458=CARTESIAN_POINT('Ctrl Pts',(7.84755972805931,-7.65190353345911,7.29399255982887));
#96459=CARTESIAN_POINT('Ctrl Pts',(7.83453293268559,-7.40320723697946,7.53706684196062));
#96460=CARTESIAN_POINT('Ctrl Pts',(7.82055549866077,-7.13636217059618,7.79787962393472));
#96461=CARTESIAN_POINT('Ctrl Pts',(7.80655344619261,-6.85586588937608,8.0448321766411));
#96462=CARTESIAN_POINT('Ctrl Pts',(7.79253868315848,-6.56314195267823,8.27617014315061));
#96463=CARTESIAN_POINT('Ctrl Pts',(7.77852392012436,-6.27041801598037,8.50750810966013));
#96464=CARTESIAN_POINT('Ctrl Pts',(7.76449645060328,-5.96546692684914,8.72323061436176));
#96465=CARTESIAN_POINT('Ctrl Pts',(7.75046860256975,-5.64975683954333,8.92161329300628));
#96466=CARTESIAN_POINT('Ctrl Pts',(7.73643453651719,-5.33390680979414,9.12008390725339));
#96467=CARTESIAN_POINT('Ctrl Pts',(7.72240009304984,-5.00728898979586,9.30119876896146));
#96468=CARTESIAN_POINT('Ctrl Pts',(7.7083779972811,-4.67208326333854,9.46439566421491));
#96469=CARTESIAN_POINT('Ctrl Pts',(7.69435590151235,-4.33687753688123,9.62759255946835));
#96470=CARTESIAN_POINT('Ctrl Pts',(7.6803461522571,-3.99308478902251,9.77287109063093));
#96471=CARTESIAN_POINT('Ctrl Pts',(7.66636185182228,-3.64290807812789,9.89971719420171));
#96472=CARTESIAN_POINT('Ctrl Pts',(7.65445708985596,-3.34480447196023,10.0077006200731));
#96473=CARTESIAN_POINT('Ctrl Pts',(7.64255734761132,-3.04196792755086,10.1024013789332));
#96474=CARTESIAN_POINT('Ctrl Pts',(7.63065709966863,-2.7355264387069,10.1835564166123));
#96475=CARTESIAN_POINT('Ctrl Pts',(7.62858144652543,-2.68207660786407,10.1977115594174));
#96476=CARTESIAN_POINT('Ctrl Pts',(7.62650577801372,-2.6285170677211,10.2114544823994));
#96477=CARTESIAN_POINT('Ctrl Pts',(7.62443006483418,-2.57485376276606,10.2247836327651));
#96478=CARTESIAN_POINT('Ctrl Pts',(7.61136764785412,-2.23715177544045,10.3086636802508));
#96479=CARTESIAN_POINT('Ctrl Pts',(7.59830284456884,-1.89532432840384,10.3761631879042));
#96480=CARTESIAN_POINT('Ctrl Pts',(7.58526635791234,-1.55097828880704,10.4267423524011));
#96481=CARTESIAN_POINT('Ctrl Pts',(7.57738000331749,-1.34266794851768,10.457339954105));
#96482=CARTESIAN_POINT('Ctrl Pts',(7.56950403796996,-1.13343670299237,10.4817448062152));
#96483=CARTESIAN_POINT('Ctrl Pts',(7.56164556698497,-0.923648317160969,
10.4998327504193));
#96484=CARTESIAN_POINT('Ctrl Pts',(7.55198659798043,-0.665794146785195,
10.5220649241789));
#96485=CARTESIAN_POINT('Ctrl Pts',(7.54235885760643,-0.407101643435756,
10.5347386581196));
#96486=CARTESIAN_POINT('Ctrl Pts',(7.53270344148809,-0.148322417901669,
10.5378431069723));
#96487=CARTESIAN_POINT('Ctrl Pts',(7.52305485201656,0.110273843547451,10.5409453608936));
#96488=CARTESIAN_POINT('Ctrl Pts',(7.51337856162289,0.368956567182821,10.5344924572168));
#96489=CARTESIAN_POINT('Ctrl Pts',(7.50361357471649,0.627026431465063,10.5184847695713));
#96490=CARTESIAN_POINT('Ctrl Pts',(7.50205789272213,0.668140121119621,10.5159345489023));
#96491=CARTESIAN_POINT('Ctrl Pts',(7.50049995672176,0.709238362916833,10.5131418363632));
#96492=CARTESIAN_POINT('Ctrl Pts',(7.49893951778007,0.750318451084926,10.5101066441853));
#96493=CARTESIAN_POINT('Ctrl Pts',(7.49893946511535,0.750319837535474,10.5101065417478));
#96494=CARTESIAN_POINT('Ctrl Pts',(7.49893941245062,0.750321223986051,10.5101064393099));
#96495=CARTESIAN_POINT('Ctrl Pts',(7.49893935978589,0.750322610436558,10.5101063368718));
#96496=CARTESIAN_POINT('Ctrl Pts',(7.48198998805347,1.19653141131127,10.4771381309561));
#96497=CARTESIAN_POINT('Ctrl Pts',(7.46508225238495,1.64030606335611,10.4146175450127));
#96498=CARTESIAN_POINT('Ctrl Pts',(7.44821688158249,2.07814433184817,10.3240954784714));
#96499=CARTESIAN_POINT('Ctrl Pts',(7.43170948506089,2.50668930693269,10.2354947792129));
#96500=CARTESIAN_POINT('Ctrl Pts',(7.41524267753539,2.92954651537385,10.1200692709601));
#96501=CARTESIAN_POINT('Ctrl Pts',(7.39881712372831,3.34346707870409,9.97930837620721));
#96502=CARTESIAN_POINT('Ctrl Pts',(7.39478374456776,3.4451074004778,9.94474381502492));
#96503=CARTESIAN_POINT('Ctrl Pts',(7.39075285267287,3.54620906299803,9.90865174356461));
#96504=CARTESIAN_POINT('Ctrl Pts',(7.38672445736098,3.64672436865318,9.87105448655237));
#96505=CARTESIAN_POINT('Ctrl Pts',(7.37411964003414,3.96123597147262,9.75341296432386));
#96506=CARTESIAN_POINT('Ctrl Pts',(7.3615169623578,4.27020880049875,9.62100692760719));
#96507=CARTESIAN_POINT('Ctrl Pts',(7.34895020829766,4.5722323797965,9.47431349544438));
#96508=CARTESIAN_POINT('Ctrl Pts',(7.33647642255021,4.87202160148474,9.32870529506109));
#96509=CARTESIAN_POINT('Ctrl Pts',(7.32403798719921,5.16496412382945,9.16901956140302));
#96510=CARTESIAN_POINT('Ctrl Pts',(7.31166977747338,5.44962988328277,8.99571647636085));
#96511=CARTESIAN_POINT('Ctrl Pts',(7.30318261108378,5.64496984916783,8.87679448593627));
#96512=CARTESIAN_POINT('Ctrl Pts',(7.29472854479695,5.83641137531478,8.75146020726419));
#96513=CARTESIAN_POINT('Ctrl Pts',(7.28631958659107,6.02347818357612,8.61986325984403));
#96514=CARTESIAN_POINT('Ctrl Pts',(7.27463137819316,6.28349562994193,8.4369473137403));
#96515=CARTESIAN_POINT('Ctrl Pts',(7.26280946049035,6.53535117459058,8.24246766819848));
#96516=CARTESIAN_POINT('Ctrl Pts',(7.25082513989488,6.77780730593302,8.03703899672175));
#96517=CARTESIAN_POINT('Ctrl Pts',(7.24996567306476,6.79519527557118,8.02230648621493));
#96518=CARTESIAN_POINT('Ctrl Pts',(7.24910537184593,6.81253492333505,8.00751767055478));
#96519=CARTESIAN_POINT('Ctrl Pts',(7.24824422611732,6.8298258026593,7.99267277976961));
#96520=CARTESIAN_POINT('Ctrl Pts',(7.24064310929476,6.98244804688657,7.86164066136463));
#96521=CARTESIAN_POINT('Ctrl Pts',(7.23297614520133,7.13126997787669,7.72623952432876));
#96522=CARTESIAN_POINT('Ctrl Pts',(7.22523669377821,7.27612659363062,7.58678420492436));
#96523=CARTESIAN_POINT('Ctrl Pts',(7.20794988167096,7.59967783287577,7.27529728264758));
#96524=CARTESIAN_POINT('Ctrl Pts',(7.19085345038819,7.90238058333808,6.94257127578086));
#96525=CARTESIAN_POINT('Ctrl Pts',(7.17393416520806,8.18237619965603,6.59192414856784));
#96526=CARTESIAN_POINT('Ctrl Pts',(7.17045404182884,8.23996842533526,6.51979963194222));
#96527=CARTESIAN_POINT('Ctrl Pts',(7.16698142602644,8.29659997351081,6.44691672877537));
#96528=CARTESIAN_POINT('Ctrl Pts',(7.16351622164847,8.35225469332804,6.37330404858248));
#96529=CARTESIAN_POINT('Ctrl Pts',(7.1511588668378,8.55072642678239,6.11079196892269));
#96530=CARTESIAN_POINT('Ctrl Pts',(7.13880542955081,8.73699807123786,5.8391004948121));
#96531=CARTESIAN_POINT('Ctrl Pts',(7.12645060901618,8.91038567592227,5.55937107268271));
#96532=CARTESIAN_POINT('Ctrl Pts',(7.1248820524924,8.93239880494414,5.5238568854272));
#96533=CARTESIAN_POINT('Ctrl Pts',(7.12331347368119,8.95420420288556,5.48821310102129));
#96534=CARTESIAN_POINT('Ctrl Pts',(7.1217448617425,8.97580041811654,5.45244202516763));
#96535=CARTESIAN_POINT('Ctrl Pts',(7.11016696045319,9.13520176015734,5.18841624859845));
#96536=CARTESIAN_POINT('Ctrl Pts',(7.09869336515209,9.28299403518174,4.91725496648527));
#96537=CARTESIAN_POINT('Ctrl Pts',(7.08726976744149,9.41861036362551,4.64013730851957));
#96538=CARTESIAN_POINT('Ctrl Pts',(7.07582835505919,9.55443818064142,4.36258749597136));
#96539=CARTESIAN_POINT('Ctrl Pts',(7.06443718727363,9.67805264090616,4.07906329225098));
#96540=CARTESIAN_POINT('Ctrl Pts',(7.0530392780045,9.78892239703109,3.79071360024181));
#96541=CARTESIAN_POINT('Ctrl Pts',(7.04163873223882,9.89981779888827,3.50229720889771));
#96542=CARTESIAN_POINT('Ctrl Pts',(7.03023142720831,9.9979632434126,3.20905351964547));
#96543=CARTESIAN_POINT('Ctrl Pts',(7.01875734339556,10.0828558637816,2.91208901810758));
#96544=CARTESIAN_POINT('Ctrl Pts',(7.01184760207909,10.1339785552311,2.73325575182819));
#96545=CARTESIAN_POINT('Ctrl Pts',(7.00491358093342,10.1802956248337,2.5530722654501));
#96546=CARTESIAN_POINT('Ctrl Pts',(6.99794178234568,10.2217007833587,2.3717717922649));
#96547=CARTESIAN_POINT('Ctrl Pts',(6.99792744780864,10.2217859154478,2.37139902499172));
#96548=CARTESIAN_POINT('Ctrl Pts',(6.99791311311183,10.2218710267728,2.37102625299427));
#96549=CARTESIAN_POINT('Ctrl Pts',(6.99789877825514,10.2219561173342,2.37065347627479));
#96550=CARTESIAN_POINT('Ctrl Pts',(6.98620503756456,10.2913692256778,2.06655875193916));
#96551=CARTESIAN_POINT('Ctrl Pts',(6.97438164383785,10.3470087783027,1.75942986008445));
#96552=CARTESIAN_POINT('Ctrl Pts',(6.96249146361515,10.3888788479672,1.45047588388174));
#96553=CARTESIAN_POINT('Ctrl Pts',(6.95054014680674,10.4309642039481,1.13993333703588));
#96554=CARTESIAN_POINT('Ctrl Pts',(6.93852148280035,10.4591373233995,0.827546860502543));
#96555=CARTESIAN_POINT('Ctrl Pts',(6.92650127112355,10.4733989646626,0.514596639856709));
#96556=CARTESIAN_POINT('Ctrl Pts',(6.92205360172844,10.4786759986347,0.398800083524568));
#96557=CARTESIAN_POINT('Ctrl Pts',(6.91760573093899,10.4820484148576,0.282926858573439));
#96558=CARTESIAN_POINT('Ctrl Pts',(6.91316102314921,10.4835164749871,0.167043612462112));
#96559=CARTESIAN_POINT('Ctrl Pts',(6.90321253510248,10.4868024004835,-0.0923352136112138));
#96560=CARTESIAN_POINT('Ctrl Pts',(6.8933906550617,10.480273521832,-0.351782186675668));
#96561=CARTESIAN_POINT('Ctrl Pts',(6.883627223104,10.4641867797313,-0.610563600947552));
#96562=CARTESIAN_POINT('Ctrl Pts',(6.87945102918872,10.4573058638025,-0.721254326540172));
#96563=CARTESIAN_POINT('Ctrl Pts',(6.87528552576304,10.4486761771571,-0.831823931034166));
#96564=CARTESIAN_POINT('Ctrl Pts',(6.87112532674824,10.4383173506522,-0.942217865737286));
#96565=CARTESIAN_POINT('Ctrl Pts',(6.85983053833117,10.4101935149399,-1.24193336746276));
#96566=CARTESIAN_POINT('Ctrl Pts',(6.84853943064584,10.3694127824273,-1.54036539315888));
#96567=CARTESIAN_POINT('Ctrl Pts',(6.83728918438053,10.3159772580025,-1.83647285089519));
#96568=CARTESIAN_POINT('Ctrl Pts',(6.83470795559292,10.3037171429194,-1.90441101652365));
#96569=CARTESIAN_POINT('Ctrl Pts',(6.83212888371649,10.2907907219817,-1.97222664598265));
#96570=CARTESIAN_POINT('Ctrl Pts',(6.82955242909833,10.2771977868899,-2.03990685551943));
#96571=CARTESIAN_POINT('Ctrl Pts',(6.81574446378667,10.2043493171716,-2.40262466897609));
#96572=CARTESIAN_POINT('Ctrl Pts',(6.80192036382046,10.1125117745603,-2.76168806542135));
#96573=CARTESIAN_POINT('Ctrl Pts',(6.78807745902409,10.0018741101773,-3.11483240124537));
#96574=CARTESIAN_POINT('Ctrl Pts',(6.77423455422773,9.89123644579426,-3.46797673706938));
#96575=CARTESIAN_POINT('Ctrl Pts',(6.76037284161516,9.76179888759734,-3.81520099936977));
#96576=CARTESIAN_POINT('Ctrl Pts',(6.74648934354437,9.61380470446798,-4.15425276629866));
#96577=CARTESIAN_POINT('Ctrl Pts',(6.73261001329415,9.46585494913316,-4.49320275002283));
#96578=CARTESIAN_POINT('Ctrl Pts',(6.71870890610072,9.29936006367006,-4.82398422208848));
#96579=CARTESIAN_POINT('Ctrl Pts',(6.70478279576421,9.11581742043377,-5.14496074671712));
#96580=CARTESIAN_POINT('Ctrl Pts',(6.69085668542771,8.93227477719748,-5.46593727134576));
#96581=CARTESIAN_POINT('Ctrl Pts',(6.67690556584498,8.73168518099751,-5.77710817676585));
#96582=CARTESIAN_POINT('Ctrl Pts',(6.6629260401176,8.51558669495431,-6.07687546169718));
#96583=CARTESIAN_POINT('Ctrl Pts',(6.64807074331246,8.28595035307013,-6.39542217615415));
#96584=CARTESIAN_POINT('Ctrl Pts',(6.63327942254754,8.03853954349429,-6.70106938587962));
#96585=CARTESIAN_POINT('Ctrl Pts',(6.61851871389973,7.77508392304408,-6.99208883334353));
#96586=CARTESIAN_POINT('Ctrl Pts',(6.6054942236311,7.54261709190193,-7.24887731497497));
#96587=CARTESIAN_POINT('Ctrl Pts',(6.59249356624743,7.29765716313496,-7.49427743212588));
#96588=CARTESIAN_POINT('Ctrl Pts',(6.57949316050575,7.04135873008535,-7.72710075685483));
#96589=CARTESIAN_POINT('Ctrl Pts',(6.56562633850373,6.76797920477563,-7.97544066763027));
#96590=CARTESIAN_POINT('Ctrl Pts',(6.55175959586778,6.48169310717675,-8.20947273883599));
#96591=CARTESIAN_POINT('Ctrl Pts',(6.53794775738398,6.18385922718087,-8.42753754943576));
#96592=CARTESIAN_POINT('Ctrl Pts',(6.52413591890019,5.886025347185,-8.64560236003553));
#96593=CARTESIAN_POINT('Ctrl Pts',(6.51037891881835,5.57664330890136,-8.84769897987254));
#96594=CARTESIAN_POINT('Ctrl Pts',(6.49673405207432,5.25712342423703,-9.03214895234355));
#96595=CARTESIAN_POINT('Ctrl Pts',(6.49673387958854,5.2571193851622,-9.03215128398949));
#96596=CARTESIAN_POINT('Ctrl Pts',(6.49673370710277,5.25711534608575,-9.0321536156326));
#96597=CARTESIAN_POINT('Ctrl Pts',(6.49673353461703,5.25711130700768,-9.0321559472729));
#96598=CARTESIAN_POINT('Ctrl Pts',(6.47784823489588,4.81487650934325,-9.28744501520444));
#96599=CARTESIAN_POINT('Ctrl Pts',(6.45884300813255,4.35359187063555,-9.50957315768382));
#96600=CARTESIAN_POINT('Ctrl Pts',(6.43975306559737,3.87857966579415,-9.69706314280026));
#96601=CARTESIAN_POINT('Ctrl Pts',(6.42033130758202,3.39531094564121,-9.88781202088218));
#96602=CARTESIAN_POINT('Ctrl Pts',(6.40082193578461,2.89783297111858,-10.0427069401333));
#96603=CARTESIAN_POINT('Ctrl Pts',(6.38126510777301,2.3918007507519,-10.1601748393213));
#96604=CARTESIAN_POINT('Ctrl Pts',(6.3783858841865,2.31730094415984,-10.1774688680769));
#96605=CARTESIAN_POINT('Ctrl Pts',(6.37550563631349,2.24261581791397,-10.1939516648252));
#96606=CARTESIAN_POINT('Ctrl Pts',(6.37262449652578,2.16776351169906,-10.2096182042152));
#96607=CARTESIAN_POINT('Ctrl Pts',(6.35286828018625,1.65449499158147,-10.3170449742732));
#96608=CARTESIAN_POINT('Ctrl Pts',(6.33306997362655,1.13336162687368,-10.3860905466361));
#96609=CARTESIAN_POINT('Ctrl Pts',(6.3132733717463,0.610349461919558,-10.4158264066385));
#96610=CARTESIAN_POINT('Ctrl Pts',(6.29373395326672,0.0941318997962036,
-10.4451759594532));
#96611=CARTESIAN_POINT('Ctrl Pts',(6.27419620422037,-0.423915227717483,
-10.4362291878969));
#96612=CARTESIAN_POINT('Ctrl Pts',(6.25470391212629,-0.937992906419497,
-10.3881184713038));
#96613=CARTESIAN_POINT('Ctrl Pts',(6.25226070791324,-1.00242846609496,-10.3820881745636));
#96614=CARTESIAN_POINT('Ctrl Pts',(6.24981822003481,-1.06680161607427,-10.3754426356291));
#96615=CARTESIAN_POINT('Ctrl Pts',(6.24737653663699,-1.13110089858024,-10.3681801908432));
#96616=CARTESIAN_POINT('Ctrl Pts',(6.24737506176842,-1.13113973776426,-10.3681758040536));
#96617=CARTESIAN_POINT('Ctrl Pts',(6.24737358690014,-1.1311785769213,-10.3681714170388));
#96618=CARTESIAN_POINT('Ctrl Pts',(6.24737211203216,-1.13121741605142,-10.3681670297989));
#96619=CARTESIAN_POINT('Ctrl Pts',(6.22417898983719,-1.74198441449639,-10.2991752343847));
#96620=CARTESIAN_POINT('Ctrl Pts',(6.20101181766919,-2.34646124507136,-10.1745430361542));
#96621=CARTESIAN_POINT('Ctrl Pts',(6.17786738316811,-2.93569442720166,-9.99822295766118));
#96622=CARTESIAN_POINT('Ctrl Pts',(6.15379904898534,-3.54844913237382,-9.81486438080322));
#96623=CARTESIAN_POINT('Ctrl Pts',(6.12975530887175,-4.14471762789403,-9.57560943680304));
#96624=CARTESIAN_POINT('Ctrl Pts',(6.10573222227401,-4.71443073759851,-9.28496134416452));
#96625=CARTESIAN_POINT('Ctrl Pts',(6.08121404253301,-5.29588509683334,-8.98832326863274));
#96626=CARTESIAN_POINT('Ctrl Pts',(6.05671737982178,-5.8496768475326,-8.63815268934198));
#96627=CARTESIAN_POINT('Ctrl Pts',(6.03223764683064,-6.36512167495428,-8.23928595966293));
#96628=CARTESIAN_POINT('Ctrl Pts',(6.0209303082614,-6.60320879704551,-8.0550469747802));
#96629=CARTESIAN_POINT('Ctrl Pts',(6.00962657594759,-6.83311473533747,-7.86041891267326));
#96630=CARTESIAN_POINT('Ctrl Pts',(5.998325967254,-7.0537891945181,-7.65588108533446));
#96631=CARTESIAN_POINT('Ctrl Pts',(5.99831956952164,-7.05391412726871,-7.65576528818481));
#96632=CARTESIAN_POINT('Ctrl Pts',(5.99831317179029,-7.05403905706055,-7.65564948785897));
#96633=CARTESIAN_POINT('Ctrl Pts',(5.99830677405993,-7.05416398389352,-7.65553368435712));
#96634=CARTESIAN_POINT('Ctrl Pts',(5.97508168029947,-7.50767440834225,-7.2351428521476));
#96635=CARTESIAN_POINT('Ctrl Pts',(5.95185196548336,-7.92212415910938,-6.7730276653975));
#96636=CARTESIAN_POINT('Ctrl Pts',(5.92862314188893,-8.2928164442724,-6.27799373205562));
#96637=CARTESIAN_POINT('Ctrl Pts',(5.90462840496468,-8.6757313958704,-5.76663727223179));
#96638=CARTESIAN_POINT('Ctrl Pts',(5.8806346180938,-9.0119563867889,-5.22015401889032));
#96639=CARTESIAN_POINT('Ctrl Pts',(5.85664836077958,-9.29627330714031,-4.64821044104104));
#96640=CARTESIAN_POINT('Ctrl Pts',(5.83271966389727,-9.57990794494461,-4.07763937074639));
#96641=CARTESIAN_POINT('Ctrl Pts',(5.80879846099807,-9.81188372396935,-3.48172845089952));
#96642=CARTESIAN_POINT('Ctrl Pts',(5.7848917759895,-9.98697203229548,-2.87005949959171));
#96643=CARTESIAN_POINT('Ctrl Pts',(5.77325976611036,-10.0721628034728,-2.57244653979286));
#96644=CARTESIAN_POINT('Ctrl Pts',(5.76163120054524,-10.1438853013618,-2.27110294951748));
#96645=CARTESIAN_POINT('Ctrl Pts',(5.75000693068917,-10.2015327465523,-1.96713277598939));
#96646=CARTESIAN_POINT('Ctrl Pts',(5.75000229790167,-10.201555721618,-1.96701163038288));
#96647=CARTESIAN_POINT('Ctrl Pts',(5.74999766511417,-10.2015786944493,-1.96689048435908));
#96648=CARTESIAN_POINT('Ctrl Pts',(5.74999303232669,-10.2016016650461,-1.96676933791808));
#96649=CARTESIAN_POINT('Ctrl Pts',(5.72266451037347,-10.3371037708125,-1.2521341023623));
#96650=CARTESIAN_POINT('Ctrl Pts',(5.69533641472616,-10.394848005795,-0.522978506931299));
#96651=CARTESIAN_POINT('Ctrl Pts',(5.66801289675197,-10.3769973889688,0.204494087600538));
#96652=CARTESIAN_POINT('Ctrl Pts',(5.63977329699423,-10.3585482904641,0.956356820785527));
#96653=CARTESIAN_POINT('Ctrl Pts',(5.61153858643246,-10.2593502213994,1.70642010905303));
#96654=CARTESIAN_POINT('Ctrl Pts',(5.58331348970829,-10.0818433849781,2.43677691238762));
#96655=CARTESIAN_POINT('Ctrl Pts',(5.5562635484521,-9.91172706811686,3.13672521794417));
#96656=CARTESIAN_POINT('Ctrl Pts',(5.5292224381274,-9.66968745763753,3.81857221540741));
#96657=CARTESIAN_POINT('Ctrl Pts',(5.50219443957856,-9.35791672220047,4.46656365982966));
#96658=CARTESIAN_POINT('Ctrl Pts',(5.50219405281362,-9.3579122608272,4.46657293245014));
#96659=CARTESIAN_POINT('Ctrl Pts',(5.50219366604868,-9.35790779943968,4.46658220506364));
#96660=CARTESIAN_POINT('Ctrl Pts',(5.50219327928375,-9.35790333803786,4.46659147767025));
#96661=CARTESIAN_POINT('Ctrl Pts',(5.46506916479616,-8.92967012276696,5.35663418252138));
#96662=CARTESIAN_POINT('Ctrl Pts',(5.42796768099261,-8.36987247228588,6.18285085526827));
#96663=CARTESIAN_POINT('Ctrl Pts',(5.39088688229172,-7.70723164974139,6.91584755034263));
#96664=CARTESIAN_POINT('Ctrl Pts',(5.3528736784168,-7.02792857198343,7.66727561515523));
#96665=CARTESIAN_POINT('Ctrl Pts',(5.31488221310929,-6.24054371848018,8.32073862513858));
#96666=CARTESIAN_POINT('Ctrl Pts',(5.27691036332006,-5.37597656080281,8.84454225364133));
#96667=CARTESIAN_POINT('Ctrl Pts',(5.26958608558794,-5.20921276035468,8.94557718540107));
#96668=CARTESIAN_POINT('Ctrl Pts',(5.26226253757739,-5.03957727573607,9.04178795673227));
#96669=CARTESIAN_POINT('Ctrl Pts',(5.25493970393503,-4.86729175390944,9.13294690721646));
#96670=CARTESIAN_POINT('Ctrl Pts',(5.25493968611562,-4.86729133466932,9.13294712904293));
#96671=CARTESIAN_POINT('Ctrl Pts',(5.25493966829622,-4.86729091542919,9.13294735086937));
#96672=CARTESIAN_POINT('Ctrl Pts',(5.25493965047681,-4.86729049618903,9.13294757269579));
#96673=CARTESIAN_POINT('Ctrl Pts',(5.21070364291279,-3.82654253050402,9.68362332642355));
#96674=CARTESIAN_POINT('Ctrl Pts',(5.16646436531577,-2.68916245918068,10.0499722137216));
#96675=CARTESIAN_POINT('Ctrl Pts',(5.12224167595592,-1.52387103549523,10.2206421596411));
#96676=CARTESIAN_POINT('Ctrl Pts',(5.08416977506241,-0.520656164649018,
10.3675741839165));
#96677=CARTESIAN_POINT('Ctrl Pts',(5.04611019969174,0.503245735025882,10.369472651501));
#96678=CARTESIAN_POINT('Ctrl Pts',(5.00807667263332,1.50395692832491,10.2190800401682));
#96679=CARTESIAN_POINT('Ctrl Pts',(5.00807571336979,1.50398216778658,10.2190762470373));
#96680=CARTESIAN_POINT('Ctrl Pts',(5.00807475410628,1.50400740723351,10.2190724538095));
#96681=CARTESIAN_POINT('Ctrl Pts',(5.00807379484279,1.50403264666567,10.2190686604848));
#96682=CARTESIAN_POINT('Ctrl Pts',(4.96444129015806,2.65205886646503,10.0465276883694));
#96683=CARTESIAN_POINT('Ctrl Pts',(4.92083357238826,3.76958415940242,9.67356309954827));
#96684=CARTESIAN_POINT('Ctrl Pts',(4.87724979701675,4.79633951199453,9.1308780752111));
#96685=CARTESIAN_POINT('Ctrl Pts',(4.83871681435949,5.7041072732183,8.6510831870242));
#96686=CARTESIAN_POINT('Ctrl Pts',(4.80020254377808,6.54092293690988,8.03862698318508));
#96687=CARTESIAN_POINT('Ctrl Pts',(4.76170628627147,7.26515529284603,7.31475570640799));
#96688=CARTESIAN_POINT('Ctrl Pts',(4.76170224698123,7.2652312842508,7.31467975289011));
#96689=CARTESIAN_POINT('Ctrl Pts',(4.76169820769119,7.26530727441612,7.31460379814559));
#96690=CARTESIAN_POINT('Ctrl Pts',(4.76169416840135,7.26538326334192,7.31452784217451));
#96691=CARTESIAN_POINT('Ctrl Pts',(4.71294834591452,8.18241146189463,6.39789733855326));
#96692=CARTESIAN_POINT('Ctrl Pts',(4.66423043686984,8.91894727366709,5.3026200862389));
#96693=CARTESIAN_POINT('Ctrl Pts',(4.61553898512807,9.43455879998508,4.11255713400774));
#96694=CARTESIAN_POINT('Ctrl Pts',(4.58228459333126,9.78670167307214,3.29978983583315));
#96695=CARTESIAN_POINT('Ctrl Pts',(4.54904254230922,10.0357967364297,2.44280989826008));
#96696=CARTESIAN_POINT('Ctrl Pts',(4.51581236975189,10.1689504712162,1.56832823132173));
#96697=CARTESIAN_POINT('Ctrl Pts',(4.50221482292277,10.2234360186839,1.21049664327063));
#96698=CARTESIAN_POINT('Ctrl Pts',(4.48861965687846,10.2585067326653,0.849744968950366));
#96699=CARTESIAN_POINT('Ctrl Pts',(4.4750268723026,10.2743826178923,0.488134898172381));
#96700=CARTESIAN_POINT('Ctrl Pts',(4.43404183365644,10.3222516741507,-0.602193771641681));
#96701=CARTESIAN_POINT('Ctrl Pts',(4.39307844339743,10.1956112695613,-1.70032308395014));
#96702=CARTESIAN_POINT('Ctrl Pts',(4.35213669516808,9.9004959265895,-2.74976740252401));
#96703=CARTESIAN_POINT('Ctrl Pts',(4.35213425480337,9.90047833601024,-2.74982995546783));
#96704=CARTESIAN_POINT('Ctrl Pts',(4.35213181443874,9.9004607448324,-2.74989250823873));
#96705=CARTESIAN_POINT('Ctrl Pts',(4.35212937407419,9.90044315305601,-2.74995506083663));
#96706=CARTESIAN_POINT('Ctrl Pts',(4.32158644227856,9.68026931644747,-3.53284617798636));
#96707=CARTESIAN_POINT('Ctrl Pts',(4.29112143584156,9.36621225935035,-4.28872013106504));
#96708=CARTESIAN_POINT('Ctrl Pts',(4.26068196180613,8.96886291644311,-4.99759054013052));
#96709=CARTESIAN_POINT('Ctrl Pts',(4.23679094882394,8.65699555964141,-5.55396126210704));
#96710=CARTESIAN_POINT('Ctrl Pts',(4.21291561406977,8.29381931908319,-6.0813783156756));
#96711=CARTESIAN_POINT('Ctrl Pts',(4.18902945460217,7.88444870906465,-6.57020010178684));
#96712=CARTESIAN_POINT('Ctrl Pts',(4.18902715704074,7.88440933253259,-6.57024712056703));
#96713=CARTESIAN_POINT('Ctrl Pts',(4.18902485947921,7.88436995557313,-6.57029413899016));
#96714=CARTESIAN_POINT('Ctrl Pts',(4.18902256191758,7.88433057818626,-6.5703411570562));
#96715=CARTESIAN_POINT('Ctrl Pts',(4.1632552257245,7.44271005679019,-7.09765250229566));
#96716=CARTESIAN_POINT('Ctrl Pts',(4.13741478222157,6.94744670774601,-7.58004695698877));
#96717=CARTESIAN_POINT('Ctrl Pts',(4.11155104549517,6.40953211685417,-8.00846912279131));
#96718=CARTESIAN_POINT('Ctrl Pts',(4.08529628275577,5.86348495795648,-8.44336847374108));
#96719=CARTESIAN_POINT('Ctrl Pts',(4.05901752914186,5.27348561834659,-8.82265002777255));
#96720=CARTESIAN_POINT('Ctrl Pts',(4.03276906429671,4.65106218177041,-9.13679878128589));
#96721=CARTESIAN_POINT('Ctrl Pts',(4.03036741752322,4.59411251835131,-9.16554234189878));
#96722=CARTESIAN_POINT('Ctrl Pts',(4.02796602575629,4.53689144154322,-9.19374061335957));
#96723=CARTESIAN_POINT('Ctrl Pts',(4.02556493144338,4.47940780021195,-9.22138629613659));
#96724=CARTESIAN_POINT('Ctrl Pts',(4.02556067586587,4.47930591912809,-9.22143529393945));
#96725=CARTESIAN_POINT('Ctrl Pts',(4.0255564202893,4.47920403721944,-9.22148429000651));
#96726=CARTESIAN_POINT('Ctrl Pts',(4.02555216471366,4.47910215448609,-9.22153328433775));
#96727=CARTESIAN_POINT('Ctrl Pts',(3.9873185556959,3.5637513479104,-9.66171582700827));
#96728=CARTESIAN_POINT('Ctrl Pts',(3.94914314148061,2.58176394555035,-9.9618342338202));
#96729=CARTESIAN_POINT('Ctrl Pts',(3.91100064892575,1.57790761846552,-10.1155811452561));
#96730=CARTESIAN_POINT('Ctrl Pts',(3.87146176774654,0.537300322533742,-10.2749566987596));
#96731=CARTESIAN_POINT('Ctrl Pts',(3.83195827482488,-0.52680434757945,-10.2770491449444));
#96732=CARTESIAN_POINT('Ctrl Pts',(3.7924602653118,-1.5645710703495,-10.1148748761191));
#96733=CARTESIAN_POINT('Ctrl Pts',(3.788594769662,-1.66613271362796,-10.0990035970754));
#96734=CARTESIAN_POINT('Ctrl Pts',(3.78472932511899,-1.76744213763999,-10.0815590438861));
#96735=CARTESIAN_POINT('Ctrl Pts',(3.78086390273701,-1.86845265557679,-10.0625346803859));
#96736=CARTESIAN_POINT('Ctrl Pts',(3.780860589853,-1.86853922726204,-10.0625183754382));
#96737=CARTESIAN_POINT('Ctrl Pts',(3.78085727696901,-1.86862579872775,-10.0625020693301));
#96738=CARTESIAN_POINT('Ctrl Pts',(3.78085396408503,-1.86871236997385,-10.0624857620616));
#96739=CARTESIAN_POINT('Ctrl Pts',(3.73455994817976,-3.07845308838546,-9.83460909809688));
#96740=CARTESIAN_POINT('Ctrl Pts',(3.68829656615448,-4.24527786346278,-9.38011420520289));
#96741=CARTESIAN_POINT('Ctrl Pts',(3.6420593453693,-5.29746547139911,-8.73927930300581));
#96742=CARTESIAN_POINT('Ctrl Pts',(3.60692904188819,-6.09690084744844,-8.25238315714807));
#96743=CARTESIAN_POINT('Ctrl Pts',(3.5718138394396,-6.83016017244939,-7.65791659589164));
#96744=CARTESIAN_POINT('Ctrl Pts',(3.53671175474974,-7.46577881040882,-6.97352719727064));
#96745=CARTESIAN_POINT('Ctrl Pts',(3.5367108904692,-7.46579446055678,-6.97351034629316));
#96746=CARTESIAN_POINT('Ctrl Pts',(3.53671002618867,-7.46581011064555,-6.97349349526117));
#96747=CARTESIAN_POINT('Ctrl Pts',(3.53670916190815,-7.46582576067513,-6.97347664417466));
#96748=CARTESIAN_POINT('Ctrl Pts',(3.4823015581945,-8.45101585130913,-5.9126784287268));
#96749=CARTESIAN_POINT('Ctrl Pts',(3.4279208344336,-9.20162723145157,-4.63584441625589));
#96750=CARTESIAN_POINT('Ctrl Pts',(3.37357498862076,-9.6634632420053,-3.2641321751324));
#96751=CARTESIAN_POINT('Ctrl Pts',(3.34671036430489,-9.89176129742237,-2.58605764199928));
#96752=CARTESIAN_POINT('Ctrl Pts',(3.31985426267946,-10.0494949150043,-1.8847995037906));
#96753=CARTESIAN_POINT('Ctrl Pts',(3.29300764938461,-10.1301213490435,-1.17499530757419));
#96754=CARTESIAN_POINT('Ctrl Pts',(3.29300737878892,-10.1301221617033,-1.17498815322841));
#96755=CARTESIAN_POINT('Ctrl Pts',(3.29300710819324,-10.1301229743554,-1.17498099888179));
#96756=CARTESIAN_POINT('Ctrl Pts',(3.29300683759755,-10.1301237869996,-1.17497384453428));
#96757=CARTESIAN_POINT('Ctrl Pts',(3.21185057929997,-10.3738496355576,0.970736917854522));
#96758=CARTESIAN_POINT('Ctrl Pts',(3.13078041734505,-9.91295623704456,3.19455927349203));
#96759=CARTESIAN_POINT('Ctrl Pts',(3.0497432811088,-8.83631410419166,5.0625402813841));
#96760=CARTESIAN_POINT('Ctrl Pts',(3.04974324576439,-8.83631363461336,5.06254109610547));
#96761=CARTESIAN_POINT('Ctrl Pts',(3.04974321041998,-8.83631316503494,5.06254191082676));
#96762=CARTESIAN_POINT('Ctrl Pts',(3.04974317507557,-8.83631269545641,5.06254272554799));
#96763=CARTESIAN_POINT('Ctrl Pts',(2.96870606622953,-7.75967038899954,6.93052279233136));
#96764=CARTESIAN_POINT('Ctrl Pts',(2.88769487591149,-6.06728729027483,8.44265309220118));
#96765=CARTESIAN_POINT('Ctrl Pts',(2.8068361779323,-4.09486592668815,9.30412583679137));
#96766=CARTESIAN_POINT('Ctrl Pts',(2.80683611536455,-4.09486440044578,9.30412650339143));
#96767=CARTESIAN_POINT('Ctrl Pts',(2.8068360527968,-4.09486287420324,9.3041271699911));
#96768=CARTESIAN_POINT('Ctrl Pts',(2.80683599022905,-4.09486134796053,9.30412783659038));
#96769=CARTESIAN_POINT('Ctrl Pts',(2.72597728129989,-2.12243927812803,10.1655996934111));
#96770=CARTESIAN_POINT('Ctrl Pts',(2.64526902547895,0.130022929717388,10.3764171800569));
#96771=CARTESIAN_POINT('Ctrl Pts',(2.56440160022704,2.22644944606699,9.9009745582931));
#96772=CARTESIAN_POINT('Ctrl Pts',(2.56440154883982,2.22645077824169,9.90097425617298));
#96773=CARTESIAN_POINT('Ctrl Pts',(2.56440149745259,2.22645211041634,9.90097395405258));
#96774=CARTESIAN_POINT('Ctrl Pts',(2.56440144606537,2.22645344259091,9.9009736519319));
#96775=CARTESIAN_POINT('Ctrl Pts',(2.50375088007378,3.79877310078287,9.54439104970355));
#96776=CARTESIAN_POINT('Ctrl Pts',(2.44301069353154,5.28332210046277,8.80178787523277));
#96777=CARTESIAN_POINT('Ctrl Pts',(2.38270289273039,6.51457988529196,7.76336126950861));
#96778=CARTESIAN_POINT('Ctrl Pts',(2.38270285132624,6.51458073060865,7.76336055657964));
#96779=CARTESIAN_POINT('Ctrl Pts',(2.38270280992208,6.51458157592522,7.76335984365053));
#96780=CARTESIAN_POINT('Ctrl Pts',(2.38270276851792,6.51458242124167,7.76335913072129));
#96781=CARTESIAN_POINT('Ctrl Pts',(2.32239495750723,7.7458400788396,6.72493193278451));
#96782=CARTESIAN_POINT('Ctrl Pts',(2.26251945886829,8.72380625407125,5.39068122422641));
#96783=CARTESIAN_POINT('Ctrl Pts',(2.20092967279735,9.34038183650534,3.904460088484));
#96784=CARTESIAN_POINT('Ctrl Pts',(2.20092964154596,9.34038214936309,3.90445933435779));
#96785=CARTESIAN_POINT('Ctrl Pts',(2.20092961029457,9.34038246222075,3.90445858023155));
#96786=CARTESIAN_POINT('Ctrl Pts',(2.20092957904319,9.34038277507832,3.90445782610527));
#96787=CARTESIAN_POINT('Ctrl Pts',(2.13933978131243,9.95695809007495,2.41823629675763));
#96788=CARTESIAN_POINT('Ctrl Pts',(2.07603570970493,10.2121426779904,0.780044366453755));
#96789=CARTESIAN_POINT('Ctrl Pts',(2.02490864864471,10.0782374348533,-0.8232068657955));
#96790=CARTESIAN_POINT('Ctrl Pts',(2.02490863093715,10.078237388476,-0.823207421072074));
#96791=CARTESIAN_POINT('Ctrl Pts',(2.0249086132296,10.0782373420987,-0.823207976348632));
#96792=CARTESIAN_POINT('Ctrl Pts',(2.02490859552205,10.0782372957213,-0.823208531625197));
#96793=CARTESIAN_POINT('Ctrl Pts',(1.97378152518914,9.94433173668894,-2.42646029494826));
#96794=CARTESIAN_POINT('Ctrl Pts',(1.93483149973001,9.42133607968513,-3.99477132083159));
#96795=CARTESIAN_POINT('Ctrl Pts',(1.89057925223621,8.56795357878977,-5.35484594214714));
#96796=CARTESIAN_POINT('Ctrl Pts',(1.84632700474241,7.71457107789448,-6.71492056346257));
#96797=CARTESIAN_POINT('Ctrl Pts',(1.79677221505219,6.53080200225584,-7.86675896507663));
#96798=CARTESIAN_POINT('Ctrl Pts',(1.74981056084319,5.14938720565873,-8.68267575370497));
#96799=CARTESIAN_POINT('Ctrl Pts',(1.70284890663419,3.7679724090616,-9.49859254233332));
#96800=CARTESIAN_POINT('Ctrl Pts',(1.65848047414983,2.18891191363664,-9.97858753801619));
#96801=CARTESIAN_POINT('Ctrl Pts',(1.61287087089241,0.588436780637463,-10.0693886900755));
#96802=CARTESIAN_POINT('Ctrl Pts',(1.56726126763499,-1.01203835236172,-10.1601898421347));
#96803=CARTESIAN_POINT('Ctrl Pts',(1.52041065882194,-2.63392819356923,-9.86179707393502));
#96804=CARTESIAN_POINT('Ctrl Pts',(1.47417904873224,-4.0963019978624,-9.20823383025107));
#96805=CARTESIAN_POINT('Ctrl Pts',(1.42794743864254,-5.55867580215555,-8.55467058656714));
#96806=CARTESIAN_POINT('Ctrl Pts',(1.38233482776403,-6.86153352960957,-7.54593681589203));
#96807=CARTESIAN_POINT('Ctrl Pts',(1.33646527388512,-7.85993138550466,-6.29513977391115));
#96808=CARTESIAN_POINT('Ctrl Pts',(1.33646525437671,-7.85993181012511,-6.29513924194485));
#96809=CARTESIAN_POINT('Ctrl Pts',(1.33646523486831,-7.85993223474552,-6.29513870997851));
#96810=CARTESIAN_POINT('Ctrl Pts',(1.3364652153599,-7.85993265936586,-6.29513817801212));
#96811=CARTESIAN_POINT('Ctrl Pts',(1.29059568077079,-8.85832983166594,-5.04434146209779));
#96812=CARTESIAN_POINT('Ctrl Pts',(1.2444691451342,-9.55226747109698,-3.55148181412588));
#96813=CARTESIAN_POINT('Ctrl Pts',(1.19848374839593,-9.86486406742352,-1.98300024121239));
#96814=CARTESIAN_POINT('Ctrl Pts',(1.19848371043099,-9.86486432549917,-1.98299894629458));
#96815=CARTESIAN_POINT('Ctrl Pts',(1.19848367246605,-9.86486458357456,-1.98299765137672));
#96816=CARTESIAN_POINT('Ctrl Pts',(1.19848363450111,-9.86486484164969,-1.98299635645881));
#96817=CARTESIAN_POINT('Ctrl Pts',(1.15249825640295,-10.1774606831884,-0.414515286520078));
#96818=CARTESIAN_POINT('Ctrl Pts',(1.10665389177668,-10.108715622417,1.22958744142003));
#96819=CARTESIAN_POINT('Ctrl Pts',(1.06077272615717,-9.6668224629688,2.76499530979388));
#96820=CARTESIAN_POINT('Ctrl Pts',(1.06077267392965,-9.66682195995227,2.76499705758183));
#96821=CARTESIAN_POINT('Ctrl Pts',(1.06077262170212,-9.66682145693525,2.76499880536965));
#96822=CARTESIAN_POINT('Ctrl Pts',(1.0607725694746,-9.66682095391775,2.76500055315732));
#96823=CARTESIAN_POINT('Ctrl Pts',(1.01489141812013,-9.22492708313986,4.30040769389711));
#96824=CARTESIAN_POINT('Ctrl Pts',(0.968973556976535,-8.40988552547852,
5.7271200694946));
#96825=CARTESIAN_POINT('Ctrl Pts',(0.923099914547117,-7.31332528013523,
6.88827573562447));
#96826=CARTESIAN_POINT('Ctrl Pts',(0.923099853871573,-7.31332382975139,
6.88827727144652));
#96827=CARTESIAN_POINT('Ctrl Pts',(0.923099793196029,-7.31332237936706,
6.88827880726812));
#96828=CARTESIAN_POINT('Ctrl Pts',(0.923099732520485,-7.31332092898224,
6.88828034308924));
#96829=CARTESIAN_POINT('Ctrl Pts',(0.877226098664229,-6.21676014107444,
8.04943509267856));
#96830=CARTESIAN_POINT('Ctrl Pts',(0.831396537222939,-4.83868108936204,
8.94503264313261));
#96831=CARTESIAN_POINT('Ctrl Pts',(0.785565047764798,-3.33266910390279,
9.47139320809289));
#96832=CARTESIAN_POINT('Ctrl Pts',(0.785565021561048,-3.33266824285372,
9.4713935090349));
#96833=CARTESIAN_POINT('Ctrl Pts',(0.785564995357298,-3.33266738180461,
9.47139380997679));
#96834=CARTESIAN_POINT('Ctrl Pts',(0.785564969153548,-3.33266652075545,
9.47139411091856));
#96835=CARTESIAN_POINT('Ctrl Pts',(0.739733508623329,-1.82665533964524,
9.99775392140918));
#96836=CARTESIAN_POINT('Ctrl Pts',(0.69390009258822,-0.192711114356479,
10.1548771844308));
#96837=CARTESIAN_POINT('Ctrl Pts',(0.648109453171715,1.38573190269856,9.93448485345363));
#96838=CARTESIAN_POINT('Ctrl Pts',(0.648109389881921,1.38573408435262,9.9344845488371));
#96839=CARTESIAN_POINT('Ctrl Pts',(0.648109326592126,1.38573626600657,9.93448424421986));
#96840=CARTESIAN_POINT('Ctrl Pts',(0.648109263302332,1.38573844766041,9.9344839396019));
#96841=CARTESIAN_POINT('Ctrl Pts',(0.602318710855294,2.96417831745571,9.71409098307494));
#96842=CARTESIAN_POINT('Ctrl Pts',(0.55657106409896,4.48711614855536,9.11618402724221));
#96843=CARTESIAN_POINT('Ctrl Pts',(0.510790325696514,5.78709048373477,8.19054629258984));
#96844=CARTESIAN_POINT('Ctrl Pts',(0.510790149412866,5.7870954894255,8.19054272832237));
#96845=CARTESIAN_POINT('Ctrl Pts',(0.510789973129217,5.78710049511293,8.19053916405004));
#96846=CARTESIAN_POINT('Ctrl Pts',(0.510789796845568,5.78710550079706,8.19053559977285));
#96847=CARTESIAN_POINT('Ctrl Pts',(0.465009082869899,7.08707741803496,7.26489584023529));
#96848=CARTESIAN_POINT('Ctrl Pts',(0.419194914517885,8.16408492797094,6.01152556991958));
#96849=CARTESIAN_POINT('Ctrl Pts',(0.373507579661479,8.89329891757632,4.60936110569497));
#96850=CARTESIAN_POINT('Ctrl Pts',(0.373507379106137,8.89330211863328,4.60935495056302));
#96851=CARTESIAN_POINT('Ctrl Pts',(0.373507178550797,8.89330531968354,4.60934879542821));
#96852=CARTESIAN_POINT('Ctrl Pts',(0.373506977995459,8.8933085207271,4.60934264029053));
#96853=CARTESIAN_POINT('Ctrl Pts',(0.327819443697221,9.6225226579455,3.20717071459683));
#96854=CARTESIAN_POINT('Ctrl Pts',(0.282261170678959,10.0039434919652,1.6562059829034));
#96855=CARTESIAN_POINT('Ctrl Pts',(0.236247419988345,10.0098541173715,0.0109034851016902));
#96856=CARTESIAN_POINT('Ctrl Pts',(20.3193161062581,-10.8205589424572,-0.0274550152749159));
#96857=CARTESIAN_POINT('Ctrl Pts',(20.3174123187361,-10.8253380330767,0.034723062884607));
#96858=CARTESIAN_POINT('Ctrl Pts',(20.3156419101068,-10.8304776395509,0.092329568131463));
#96859=CARTESIAN_POINT('Ctrl Pts',(20.3139884606019,-10.838945329927,0.146171788417064));
#96860=CARTESIAN_POINT('Ctrl Pts',(20.313582681329,-10.8417916635006,0.159397329278271));
#96861=CARTESIAN_POINT('Ctrl Pts',(20.3132737488013,-10.8459274194006,0.16951983910409));
#96862=CARTESIAN_POINT('Ctrl Pts',(20.3132119638891,-10.8470106149663,0.171551138051299));
#96863=CARTESIAN_POINT('Ctrl Pts',(20.3131578861053,-10.8486133792296,0.17334615859031));
#96864=CARTESIAN_POINT('Ctrl Pts',(20.3131442649206,-10.8491158658176,0.173800871954156));
#96865=CARTESIAN_POINT('Ctrl Pts',(20.313129658019,-10.8500405501164,0.174298436740182));
#96866=CARTESIAN_POINT('Ctrl Pts',(20.313125892081,-10.850423694506,0.174430447775073));
#96867=CARTESIAN_POINT('Ctrl Pts',(20.313124076547,-10.851186062719,0.174508900562405));
#96868=CARTESIAN_POINT('Ctrl Pts',(20.3131254455118,-10.8515368492789,0.174473476044135));
#96869=CARTESIAN_POINT('Ctrl Pts',(20.3131327610704,-10.8522949105386,0.174255487039109));
#96870=CARTESIAN_POINT('Ctrl Pts',(20.3131393815545,-10.8526798380712,0.174050470864689));
#96871=CARTESIAN_POINT('Ctrl Pts',(20.3131611608867,-10.8536464139303,0.173368233548088));
#96872=CARTESIAN_POINT('Ctrl Pts',(20.3131798412209,-10.8541953909257,0.172775776396129));
#96873=CARTESIAN_POINT('Ctrl Pts',(20.3132437615228,-10.8557810771898,0.17074055793655));
#96874=CARTESIAN_POINT('Ctrl Pts',(20.3133043635337,-10.8567788351687,0.168797239405895));
#96875=CARTESIAN_POINT('Ctrl Pts',(20.3144462591772,-10.872740236646,0.132090055974202));
#96876=CARTESIAN_POINT('Ctrl Pts',(20.3187259620078,-10.8834290614676,-0.00816301187489857));
#96877=CARTESIAN_POINT('Ctrl Pts',(20.3193037808912,-10.8848592494362,-0.0272277890842044));
#96878=CARTESIAN_POINT('Ctrl Pts',(1.71371885186958,10.8205931966853,-0.0274987012850931));
#96879=CARTESIAN_POINT('Ctrl Pts',(1.71468534383149,10.822944877955,0.0031147715923076));
#96880=CARTESIAN_POINT('Ctrl Pts',(1.71561699929121,10.8253939137338,0.0326182964624533));
#96881=CARTESIAN_POINT('Ctrl Pts',(1.71645436246431,10.8279623679907,0.0591357896026434));
#96882=CARTESIAN_POINT('Ctrl Pts',(1.71731777406016,10.8306107208919,0.0864781803428588));
#96883=CARTESIAN_POINT('Ctrl Pts',(1.71808091120447,10.83338814387,0.110645999870019));
#96884=CARTESIAN_POINT('Ctrl Pts',(1.71867722902095,10.8363614917576,0.129574074291803));
#96885=CARTESIAN_POINT('Ctrl Pts',(1.7191988450607,10.8389623631505,0.146130995697381));
#96886=CARTESIAN_POINT('Ctrl Pts',(1.71961433221267,10.8418050748521,0.159355934500197));
#96887=CARTESIAN_POINT('Ctrl Pts',(1.71985385804639,10.8449464085218,0.167054167370949));
#96888=CARTESIAN_POINT('Ctrl Pts',(1.71992928349054,10.8459355982203,0.169478301020406));
#96889=CARTESIAN_POINT('Ctrl Pts',(1.71999209380181,10.8470174704317,0.171509656335478));
#96890=CARTESIAN_POINT('Ctrl Pts',(1.72003208873138,10.848191838748,0.172826512697616));
#96891=CARTESIAN_POINT('Ctrl Pts',(1.72004661177751,10.8486182779345,0.17330469245437));
#96892=CARTESIAN_POINT('Ctrl Pts',(1.72006027466401,10.849120139148,0.173759399065278));
#96893=CARTESIAN_POINT('Ctrl Pts',(1.72006907171516,10.8496850261903,0.174063734720378));
#96894=CARTESIAN_POINT('Ctrl Pts',(1.72007465702634,10.8500436770448,0.17425695962123));
#96895=CARTESIAN_POINT('Ctrl Pts',(1.72007826406952,10.8504263471907,0.174388971008971));
#96896=CARTESIAN_POINT('Ctrl Pts',(1.72007897475741,10.850831577322,0.174430726563144));
#96897=CARTESIAN_POINT('Ctrl Pts',(1.72007959945218,10.8511877746751,0.174467429702221));
#96898=CARTESIAN_POINT('Ctrl Pts',(1.72007794588743,10.851538129416,0.17443201029948));
#96899=CARTESIAN_POINT('Ctrl Pts',(1.72007428397974,10.8518822489634,0.174332940383375));
#96900=CARTESIAN_POINT('Ctrl Pts',(1.72006988897607,10.8522952595587,0.174214037155319));
#96901=CARTESIAN_POINT('Ctrl Pts',(1.72006280779778,10.8526797158702,0.174009032859097));
#96902=CARTESIAN_POINT('Ctrl Pts',(1.72005441611114,10.8530306271272,0.173761060114384));
#96903=CARTESIAN_POINT('Ctrl Pts',(1.72003972135017,10.8536451111113,0.173326832721801));
#96904=CARTESIAN_POINT('Ctrl Pts',(1.72002011456704,10.854193422193,0.172734406146005));
#96905=CARTESIAN_POINT('Ctrl Pts',(1.72000063610676,10.85465461806,0.172141778503934));
#96906=CARTESIAN_POINT('Ctrl Pts',(1.71995322459096,10.8557771911396,0.170699294117637));
#96907=CARTESIAN_POINT('Ctrl Pts',(1.71989015281157,10.8567737612288,0.168756077607141));
#96908=CARTESIAN_POINT('Ctrl Pts',(1.71982793196062,10.8576097087584,0.166831443441117));
#96909=CARTESIAN_POINT('Ctrl Pts',(1.71954665823757,10.8613886682289,0.158130999632178));
#96910=CARTESIAN_POINT('Ctrl Pts',(1.71905811143705,10.8649667346043,0.142845235796171));
#96911=CARTESIAN_POINT('Ctrl Pts',(1.71847477844653,10.8681807676781,0.124502662428512));
#96912=CARTESIAN_POINT('Ctrl Pts',(1.71794817753767,10.8710822197908,0.107943997029649));
#96913=CARTESIAN_POINT('Ctrl Pts',(1.71734433393044,10.8736847458312,0.0888946809006036));
#96914=CARTESIAN_POINT('Ctrl Pts',(1.71674529327921,10.875903541945,0.0699625924862081));
#96915=CARTESIAN_POINT('Ctrl Pts',(1.71612325783427,10.8782075088378,0.0503037763168473));
#96916=CARTESIAN_POINT('Ctrl Pts',(1.71550633896194,10.8800975192133,0.0307717296376784));
#96917=CARTESIAN_POINT('Ctrl Pts',(1.71498600196939,10.8815377327113,0.0142938555230019));
#96918=CARTESIAN_POINT('Ctrl Pts',(1.71434319878671,10.8833169139602,-0.0060622407692471));
#96919=CARTESIAN_POINT('Ctrl Pts',(1.71384733713533,10.8844151671384,-0.0217562947441692));
#96920=CARTESIAN_POINT('Ctrl Pts',(1.71367396487917,10.884828376917,-0.0272688936357385));
#96921=CARTESIAN_POINT('Ctrl Pts',(0.236247419988345,10.0098541173715,0.0109034851016902));
#96922=CARTESIAN_POINT('Ctrl Pts',(0.282261170678959,10.0039434919652,1.6562059829034));
#96923=CARTESIAN_POINT('Ctrl Pts',(0.373376072507811,9.24109505723063,4.75816615273069));
#96924=CARTESIAN_POINT('Ctrl Pts',(0.510813799656914,6.01005809224591,8.51828336844459));
#96925=CARTESIAN_POINT('Ctrl Pts',(0.648055013464543,1.44123444891801,10.3120076322213));
#96926=CARTESIAN_POINT('Ctrl Pts',(0.785560276845269,-3.46060058477824,
9.84063572967199));
#96927=CARTESIAN_POINT('Ctrl Pts',(0.923051233060837,-7.5948417795504,7.15384051951451));
#96928=CARTESIAN_POINT('Ctrl Pts',(1.06080804358272,-10.0399709608217,2.87369562638161));
#96929=CARTESIAN_POINT('Ctrl Pts',(1.19834240096617,-10.2462067287989,-2.05861808649073));
#96930=CARTESIAN_POINT('Ctrl Pts',(1.33672216659611,-8.16439259011698,-6.53720175974399));
#96931=CARTESIAN_POINT('Ctrl Pts',(1.47356002226354,-4.25581898226483,-9.56340404211238));
#96932=CARTESIAN_POINT('Ctrl Pts',(1.61411187128628,0.609851298358065,-10.4585827142956));
#96933=CARTESIAN_POINT('Ctrl Pts',(1.74721742089645,5.34703287910853,-9.01859753161106));
#96934=CARTESIAN_POINT('Ctrl Pts',(1.8958818256709,8.89834087463024,-5.56308141247177));
#96935=CARTESIAN_POINT('Ctrl Pts',(2.01273080137881,10.4673283008352,-0.858147598243681));
#96936=CARTESIAN_POINT('Ctrl Pts',(2.20264435693172,9.70177269289523,4.05643050727519));
#96937=CARTESIAN_POINT('Ctrl Pts',(2.3822686105234,6.76787291889619,8.05918655449917));
#96938=CARTESIAN_POINT('Ctrl Pts',(2.58473753279966,1.81936906742815,10.5345311540723));
#96939=CARTESIAN_POINT('Ctrl Pts',(2.80668585042627,-4.37490532884103,9.95478178818736));
#96940=CARTESIAN_POINT('Ctrl Pts',(3.04970976329908,-9.4520606964986,5.41839539962617));
#96941=CARTESIAN_POINT('Ctrl Pts',(3.29292182462279,-10.8347486360525,-1.25311526530803));
#96942=CARTESIAN_POINT('Ctrl Pts',(3.53664883451739,-7.9896728535523,-7.45590618383817));
#96943=CARTESIAN_POINT('Ctrl Pts',(3.78075336580612,-2.00123281219044,-10.7644231829639));
#96944=CARTESIAN_POINT('Ctrl Pts',(3.99813845688202,4.02995046692096,-9.96214692229989));
#96945=CARTESIAN_POINT('Ctrl Pts',(4.18862746148973,8.12371844357838,-6.77022205761317));
#96946=CARTESIAN_POINT('Ctrl Pts',(4.35210354637076,10.199344026804,-2.83597488023603));
#96947=CARTESIAN_POINT('Ctrl Pts',(4.54305768697987,10.5289705057324,2.35743250402144));
#96948=CARTESIAN_POINT('Ctrl Pts',(4.76162944769493,7.77638110638611,7.82086590797216));
#96949=CARTESIAN_POINT('Ctrl Pts',(5.00798370995861,1.61236315088105,10.9305672780317));
#96950=CARTESIAN_POINT('Ctrl Pts',(5.25480916755377,-5.20207512827217,9.7714803690324));
#96951=CARTESIAN_POINT('Ctrl Pts',(5.50210984394784,-10.0080544559059,4.78164235860356));
#96952=CARTESIAN_POINT('Ctrl Pts',(5.74989536055484,-10.9132436390617,-2.09865134769182));
#96953=CARTESIAN_POINT('Ctrl Pts',(5.99817059546363,-7.54875564608264,-8.18768977461551));
#96954=CARTESIAN_POINT('Ctrl Pts',(6.20547988627588,-2.27065875717826,-10.6033776168208));
#96955=CARTESIAN_POINT('Ctrl Pts',(6.37157872831103,2.2034281101606,-10.38310575704));
#96956=CARTESIAN_POINT('Ctrl Pts',(6.5378458851255,6.39609170629518,-8.79205815441647));
#96957=CARTESIAN_POINT('Ctrl Pts',(6.74599686093403,10.2823120730407,-4.45053869669907));
#96958=CARTESIAN_POINT('Ctrl Pts',(6.99629129235853,10.940060962212,2.53477782652384));
#96959=CARTESIAN_POINT('Ctrl Pts',(7.24710420019219,7.31061279457704,8.54766467124672));
#96960=CARTESIAN_POINT('Ctrl Pts',(7.49843906124326,0.807422651314364,11.2437313176264));
#96961=CARTESIAN_POINT('Ctrl Pts',(7.75030187340421,-6.03794504664792,9.54528916818388));
#96962=CARTESIAN_POINT('Ctrl Pts',(8.00269551261862,-10.5549932902737,4.10604724051843));
#96963=CARTESIAN_POINT('Ctrl Pts',(8.21346992637613,-10.8796133252787,-1.78960216096524));
#96964=CARTESIAN_POINT('Ctrl Pts',(8.38235875812152,-9.00997128676483,-5.94254396635746));
#96965=CARTESIAN_POINT('Ctrl Pts',(8.55142780992127,-5.94780734069486,-9.31990615096143));
#96966=CARTESIAN_POINT('Ctrl Pts',(8.76310273990339,-0.391070994991625,
-11.3900354500284));
#96967=CARTESIAN_POINT('Ctrl Pts',(8.98937409723999,5.69639989756584,-9.62925783989565));
#96968=CARTESIAN_POINT('Ctrl Pts',(9.18771619472723,9.41506511084373,-5.71114232305533));
#96969=CARTESIAN_POINT('Ctrl Pts',(9.35796785690745,10.9487245660541,-1.3352779507663));
#96970=CARTESIAN_POINT('Ctrl Pts',(9.50952001769988,10.5851488734647,2.77388645518095));
#96971=CARTESIAN_POINT('Ctrl Pts',(9.6802207005967,8.6323656393866,6.93167007488376));
#96972=CARTESIAN_POINT('Ctrl Pts',(9.8511669282714,5.03341926711359,10.005370594796));
#96973=CARTESIAN_POINT('Ctrl Pts',(10.0414263863103,-0.0370302011065132,
11.0900539763085));
#96974=CARTESIAN_POINT('Ctrl Pts',(10.2129064709966,-4.60117272512858,10.1123079833804));
#96975=CARTESIAN_POINT('Ctrl Pts',(10.3846334810773,-8.36249887462001,7.333757088142));
#96976=CARTESIAN_POINT('Ctrl Pts',(10.5852700849522,-11.0438636264105,2.5710018780358));
#96977=CARTESIAN_POINT('Ctrl Pts',(10.8149812572377,-10.9327543857081,-3.85881574900101));
#96978=CARTESIAN_POINT('Ctrl Pts',(11.0739634856436,-6.51596063212015,-9.61787231659027));
#96979=CARTESIAN_POINT('Ctrl Pts',(11.3335027624831,0.467553896182886,-11.6326133959484));
#96980=CARTESIAN_POINT('Ctrl Pts',(11.5935990303907,7.30006443089141,-9.10202411414065));
#96981=CARTESIAN_POINT('Ctrl Pts',(11.8542514832384,11.3018959077801,-2.99469731082429));
#96982=CARTESIAN_POINT('Ctrl Pts',(12.1154595427833,10.8959931621228,4.30909650104135));
#96983=CARTESIAN_POINT('Ctrl Pts',(12.3772218554197,6.21966653448416,9.9610404039248));
#96984=CARTESIAN_POINT('Ctrl Pts',(12.6103907594023,-0.116341202195039,
11.5293645744839));
#96985=CARTESIAN_POINT('Ctrl Pts',(12.8147708022338,-5.45592049951901,9.9487140666827));
#96986=CARTESIAN_POINT('Ctrl Pts',(12.9901979397853,-9.07795159496635,6.83698031594479));
#96987=CARTESIAN_POINT('Ctrl Pts',(13.1658687037173,-11.1011708103344,2.50074889324405));
#96988=CARTESIAN_POINT('Ctrl Pts',(13.3417822439288,-11.1644930733986,-2.28894820766289));
#96989=CARTESIAN_POINT('Ctrl Pts',(13.5179379354906,-9.24673925825825,-6.68611271245235));
#96990=CARTESIAN_POINT('Ctrl Pts',(13.6796349152431,-5.98273132472607,-9.64237799750398));
#96991=CARTESIAN_POINT('Ctrl Pts',(13.8268076250129,-2.27546195949532,-11.054929025411));
#96992=CARTESIAN_POINT('Ctrl Pts',(14.0035943286413,2.48773327673549,-11.2885440550832));
#96993=CARTESIAN_POINT('Ctrl Pts',(14.2249137140213,8.12400984323024,-8.72005906989793));
#96994=CARTESIAN_POINT('Ctrl Pts',(14.491030376488,11.7338624047256,-2.18962997847152));
#96995=CARTESIAN_POINT('Ctrl Pts',(14.7576764173397,10.7646370052319,5.21155646912779));
#96996=CARTESIAN_POINT('Ctrl Pts',(15.0248485147023,5.57521599023327,10.6101885382146));
#96997=CARTESIAN_POINT('Ctrl Pts',(15.2627969903976,-0.992496529899604,
11.7232808389446));
#96998=CARTESIAN_POINT('Ctrl Pts',(15.4713367560048,-6.30461690989114,9.70932698413165));
#96999=CARTESIAN_POINT('Ctrl Pts',(15.6503127453385,-9.75400287905629,6.26911361970484));
#97000=CARTESIAN_POINT('Ctrl Pts',(15.8295149691491,-11.4822959817887,1.70334083365234));
#97001=CARTESIAN_POINT('Ctrl Pts',(16.0089418448568,-11.181216258242,-3.17259926566968));
#97002=CARTESIAN_POINT('Ctrl Pts',(16.188591039425,-8.89748663297175,-7.50014918261716));
#97003=CARTESIAN_POINT('Ctrl Pts',(16.3684625089748,-5.03250485728561,-10.5077706500309));
#97004=CARTESIAN_POINT('Ctrl Pts',(16.5485511407028,-0.265185102376701,
-11.6644002694677));
#97005=CARTESIAN_POINT('Ctrl Pts',(16.7288620799578,4.55737364209454,-10.7511864391277));
#97006=CARTESIAN_POINT('Ctrl Pts',(16.9394631424965,9.2650231182667,-7.47067789966794));
#97007=CARTESIAN_POINT('Ctrl Pts',(17.1805382346314,12.0898447529122,-1.34171254597968));
#97008=CARTESIAN_POINT('Ctrl Pts',(17.4521367413488,10.5409864853984,6.10996614926754));
#97009=CARTESIAN_POINT('Ctrl Pts',(17.724365137213,4.86145703151405,11.1967036665295));
#97010=CARTESIAN_POINT('Ctrl Pts',(17.9739918587982,-2.10415293108078,11.8489255250914));
#97011=CARTESIAN_POINT('Ctrl Pts',(18.202015234118,-7.68156807420211,9.06610251823513));
#97012=CARTESIAN_POINT('Ctrl Pts',(18.4054199419476,-10.9997362923052,4.53187719411499));
#97013=CARTESIAN_POINT('Ctrl Pts',(18.6198245873421,-11.8684771618245,-1.01371487948541));
#97014=CARTESIAN_POINT('Ctrl Pts',(18.7524864795234,-10.0876335066935,-6.35323592041183));
#97015=CARTESIAN_POINT('Ctrl Pts',(18.9215214647306,-6.05127039623785,-10.2851587824557));
#97016=CARTESIAN_POINT('Ctrl Pts',(19.0731272889727,-0.65573725462633,-11.9250004543447));
#97017=CARTESIAN_POINT('Ctrl Pts',(19.2334715077428,4.89535067915303,-10.9054852425954));
#97018=CARTESIAN_POINT('Ctrl Pts',(19.3898602964296,9.36302270195755,-7.44777342140719));
#97019=CARTESIAN_POINT('Ctrl Pts',(19.5482566143342,11.746908296497,-2.3215667695402));
#97020=CARTESIAN_POINT('Ctrl Pts',(19.7059549578916,11.5117047090732,3.33316592178669));
#97021=CARTESIAN_POINT('Ctrl Pts',(19.8641448857339,8.70443639357988,8.25003611575385));
#97022=CARTESIAN_POINT('Ctrl Pts',(20.0223213623772,3.95007659628246,11.3388902742205));
#97023=CARTESIAN_POINT('Ctrl Pts',(20.1806504341427,-1.69684253053496,11.8871678578889));
#97024=CARTESIAN_POINT('Ctrl Pts',(20.3391911994786,-6.96836333841185,9.80977543797914));
#97025=CARTESIAN_POINT('Ctrl Pts',(20.4976257595637,-10.7023126456679,5.48047659314321));
#97026=CARTESIAN_POINT('Ctrl Pts',(20.6037145486049,-11.585908889594,1.86712555758727));
#97027=CARTESIAN_POINT('Ctrl Pts',(20.6563591733144,-11.5926712737699,-0.0152754849923013));
#97028=CARTESIAN_POINT('Ctrl Pts',(0.414857473372219,9.90423208112614,0.00552890457929189));
#97029=CARTESIAN_POINT('Ctrl Pts',(0.460418169951906,9.89837965208721,1.63463165667105));
#97030=CARTESIAN_POINT('Ctrl Pts',(0.550524238756086,9.14347953248729,4.70199787951103));
#97031=CARTESIAN_POINT('Ctrl Pts',(0.686487743555868,5.94756858734584,8.42194829459827));
#97032=CARTESIAN_POINT('Ctrl Pts',(0.822188845948616,1.4295973741879,10.1949329202965));
#97033=CARTESIAN_POINT('Ctrl Pts',(0.958137305849702,-3.41644857527999,
9.72909274177817));
#97034=CARTESIAN_POINT('Ctrl Pts',(1.09403361926965,-7.50266239378958,7.07318924692806));
#97035=CARTESIAN_POINT('Ctrl Pts',(1.23016410051787,-9.91874295184523,2.84369449537073));
#97036=CARTESIAN_POINT('Ctrl Pts',(1.36604419717911,-10.1223645889116,-2.02923787138832));
#97037=CARTESIAN_POINT('Ctrl Pts',(1.50272853890757,-8.06598625809779,-6.45277962201427));
#97038=CARTESIAN_POINT('Ctrl Pts',(1.63786199458176,-4.2061118422785,-9.44114405015345));
#97039=CARTESIAN_POINT('Ctrl Pts',(1.77663105190054,0.597760567220721,-10.3247533804463));
#97040=CARTESIAN_POINT('Ctrl Pts',(1.90802235015697,5.27380437963824,-8.90337943938992));
#97041=CARTESIAN_POINT('Ctrl Pts',(2.05474079138054,8.77838187416392,-5.49286562090779));
#97042=CARTESIAN_POINT('Ctrl Pts',(2.17004101494486,10.3264823775258,-0.850681306693522));
#97043=CARTESIAN_POINT('Ctrl Pts',(2.35731632897177,9.57112254251312,3.99528315347118));
#97044=CARTESIAN_POINT('Ctrl Pts',(2.53450866734066,6.67744212272248,7.94394089643617));
#97045=CARTESIAN_POINT('Ctrl Pts',(2.73411483620783,1.79849490485795,10.3837363556879));
#97046=CARTESIAN_POINT('Ctrl Pts',(2.95290126451474,-4.30712195173813,9.81235656214055));
#97047=CARTESIAN_POINT('Ctrl Pts',(3.19236937666179,-9.30963369487423,5.34191601965425));
#97048=CARTESIAN_POINT('Ctrl Pts',(3.43194408501429,-10.6713573734611,-1.22966566693323));
#97049=CARTESIAN_POINT('Ctrl Pts',(3.67195964496792,-7.86933007701237,-7.33773481169104));
#97050=CARTESIAN_POINT('Ctrl Pts',(3.91227453885146,-1.97387050712104,-10.5945289197493));
#97051=CARTESIAN_POINT('Ctrl Pts',(4.12623048182538,3.96194440519949,-9.80466577550004));
#97052=CARTESIAN_POINT('Ctrl Pts',(4.31366124218865,7.98986025797959,-6.66394873887548));
#97053=CARTESIAN_POINT('Ctrl Pts',(4.47448428722267,10.0317165049964,-2.79356697241387));
#97054=CARTESIAN_POINT('Ctrl Pts',(4.66230978502311,10.3558279725464,2.31468255910313));
#97055=CARTESIAN_POINT('Ctrl Pts',(4.87726295846424,7.64870922201446,7.68740832032523));
#97056=CARTESIAN_POINT('Ctrl Pts',(5.11947477571608,1.58835118409914,10.7445226945064));
#97057=CARTESIAN_POINT('Ctrl Pts',(5.36209607434172,-5.1097851329423,9.60498844990581));
#97058=CARTESIAN_POINT('Ctrl Pts',(5.60512955006172,-9.8325723537292,4.70119518673858));
#97059=CARTESIAN_POINT('Ctrl Pts',(5.84859118648436,-10.721707014825,-2.05887588402894));
#97060=CARTESIAN_POINT('Ctrl Pts',(6.09248402304501,-7.41650091760526,-8.04022127100391));
#97061=CARTESIAN_POINT('Ctrl Pts',(6.29610216773837,-2.23247694919502,-10.412668314822));
#97062=CARTESIAN_POINT('Ctrl Pts',(6.45921389034127,2.1610887235209,-10.1963335049597));
#97063=CARTESIAN_POINT('Ctrl Pts',(6.62247800296255,6.27795117697407,-8.63400813873752));
#97064=CARTESIAN_POINT('Ctrl Pts',(6.82685309104326,10.0935096431048,-4.37126941277162));
#97065=CARTESIAN_POINT('Ctrl Pts',(7.07257095820066,10.7389892523422,2.48613635755055));
#97066=CARTESIAN_POINT('Ctrl Pts',(7.31875400381713,7.17651830463057,8.38788425967839));
#97067=CARTESIAN_POINT('Ctrl Pts',(7.56542542195868,0.7940738232045,11.0337241535568));
#97068=CARTESIAN_POINT('Ctrl Pts',(7.81258883522782,-5.92334267223987,9.36691902027508));
#97069=CARTESIAN_POINT('Ctrl Pts',(8.06023568790507,-10.355305921526,4.02992322014796));
#97070=CARTESIAN_POINT('Ctrl Pts',(8.26704359020869,-10.6737649965103,-1.7545294942458));
#97071=CARTESIAN_POINT('Ctrl Pts',(8.43273095233146,-8.83955444072362,-5.82870686778807));
#97072=CARTESIAN_POINT('Ctrl Pts',(8.59859108870107,-5.83554619435488,-9.1418987825165));
#97073=CARTESIAN_POINT('Ctrl Pts',(8.80624576829024,-0.38447258030216,-11.1726177352634));
#97074=CARTESIAN_POINT('Ctrl Pts',(9.02820909153645,5.58689185174015,-9.44533260690079));
#97075=CARTESIAN_POINT('Ctrl Pts',(9.22275895514135,9.23437826127017,-5.60217944378132));
#97076=CARTESIAN_POINT('Ctrl Pts',(9.38974987490141,10.738646239023,-1.31016596208437));
#97077=CARTESIAN_POINT('Ctrl Pts',(9.53840307001713,10.382012686018,2.72029969805813));
#97078=CARTESIAN_POINT('Ctrl Pts',(9.70583136768617,8.46668714972023,6.79831087477145));
#97079=CARTESIAN_POINT('Ctrl Pts',(9.87349729187605,4.93684808690671,9.81299815163281));
#97080=CARTESIAN_POINT('Ctrl Pts',(10.0601111882738,-0.0363289028640763,
10.8768934600605));
#97081=CARTESIAN_POINT('Ctrl Pts',(10.2282978646472,-4.51277420606732,9.91792503778587));
#97082=CARTESIAN_POINT('Ctrl Pts',(10.3967352451322,-8.20197618078149,7.19270305477791));
#97083=CARTESIAN_POINT('Ctrl Pts',(10.5935240094408,-10.831887292633,2.52135107060561));
#97084=CARTESIAN_POINT('Ctrl Pts',(10.8188415967134,-10.722977073751,-3.78530740392195));
#97085=CARTESIAN_POINT('Ctrl Pts',(11.072873928545,-6.39071183862135,-9.43422014294441));
#97086=CARTESIAN_POINT('Ctrl Pts',(11.3274651584233,0.459488233287932,-11.4105773080049));
#97087=CARTESIAN_POINT('Ctrl Pts',(11.5826156827513,7.16198049444802,-8.92822222363093));
#97088=CARTESIAN_POINT('Ctrl Pts',(11.8383292692865,11.0879837567681,-2.93677974621958));
#97089=CARTESIAN_POINT('Ctrl Pts',(12.0946076320618,10.6898359444383,4.22903042659061));
#97090=CARTESIAN_POINT('Ctrl Pts',(12.3514514772082,6.10154484510121,9.77475286626462));
#97091=CARTESIAN_POINT('Ctrl Pts',(12.5802650565851,-0.115947755772311,
11.3138309860641));
#97092=CARTESIAN_POINT('Ctrl Pts',(12.7808402128593,-5.35607564736957,9.76266262815981));
#97093=CARTESIAN_POINT('Ctrl Pts',(12.9530170339153,-8.91094778509916,6.7086566819509));
#97094=CARTESIAN_POINT('Ctrl Pts',(13.12544599583,-10.8968596648658,2.45251970711059));
#97095=CARTESIAN_POINT('Ctrl Pts',(13.2981269698541,-10.9590328324087,-2.24910381637141));
#97096=CARTESIAN_POINT('Ctrl Pts',(13.4710607907509,-9.07644430667711,-6.56582822441653));
#97097=CARTESIAN_POINT('Ctrl Pts',(13.629817907228,-5.8718461928328,-9.46833191108338));
#97098=CARTESIAN_POINT('Ctrl Pts',(13.7743254679023,-2.23176961892461,-10.8553170599986));
#97099=CARTESIAN_POINT('Ctrl Pts',(13.947922654666,2.44544351510108,-11.0847627749313));
#97100=CARTESIAN_POINT('Ctrl Pts',(14.1652771291645,7.9807212902622,-8.56247132454596));
#97101=CARTESIAN_POINT('Ctrl Pts',(14.426673351802,11.5266952104283,-2.14812344542611));
#97102=CARTESIAN_POINT('Ctrl Pts',(14.6886334109526,10.5747101394929,5.12290089122906));
#97103=CARTESIAN_POINT('Ctrl Pts',(14.9511576251903,5.47582248770765,10.4277192621086));
#97104=CARTESIAN_POINT('Ctrl Pts',(15.1850168097518,-0.978866148033905,
11.5218445338106));
#97105=CARTESIAN_POINT('Ctrl Pts',(15.3899998038495,-6.20039383677261,9.54233873489365));
#97106=CARTESIAN_POINT('Ctrl Pts',(15.5659485697773,-9.5914515069554,6.16037833139429));
#97107=CARTESIAN_POINT('Ctrl Pts',(15.7421485688689,-11.290841170853,1.67118798331995));
#97108=CARTESIAN_POINT('Ctrl Pts',(15.91859349859,-10.9948392663885,-3.12368117664651));
#97109=CARTESIAN_POINT('Ctrl Pts',(16.0952847407158,-8.7488133900966,-7.37996072217231));
#97110=CARTESIAN_POINT('Ctrl Pts',(16.2722211526758,-4.94699126663771,-10.3385555770745));
#97111=CARTESIAN_POINT('Ctrl Pts',(16.4493977178716,-0.256815859048274,
-11.4765472264812));
#97112=CARTESIAN_POINT('Ctrl Pts',(16.6268217932286,4.48852118140762,-10.5780577674155));
#97113=CARTESIAN_POINT('Ctrl Pts',(16.8340855571211,9.12157653404527,-7.34965948087608));
#97114=CARTESIAN_POINT('Ctrl Pts',(17.0713925325136,11.9024947483016,-1.31664378789847));
#97115=CARTESIAN_POINT('Ctrl Pts',(17.3388171639219,10.3777655633468,6.02036145965717));
#97116=CARTESIAN_POINT('Ctrl Pts',(17.6069246364637,4.78440903108591,11.0305903935865));
#97117=CARTESIAN_POINT('Ctrl Pts',(17.8528590762609,-2.07781594109665,11.6730984248505));
#97118=CARTESIAN_POINT('Ctrl Pts',(18.0775302086984,-7.57370613884857,8.9316707861517));
#97119=CARTESIAN_POINT('Ctrl Pts',(18.2780483340467,-10.8443366541153,4.46167669141483));
#97120=CARTESIAN_POINT('Ctrl Pts',(18.4893454671788,-11.7009227432788,-1.00327493205492));
#97121=CARTESIAN_POINT('Ctrl Pts',(18.620155096919,-9.94500696839018,-6.26795196146921));
#97122=CARTESIAN_POINT('Ctrl Pts',(18.7868531643319,-5.96462321927576,-10.1457961598287));
#97123=CARTESIAN_POINT('Ctrl Pts',(18.9363899977649,-0.642776950505896,
-11.7632196848552));
#97124=CARTESIAN_POINT('Ctrl Pts',(19.0945718779567,4.83344916781054,-10.7576469690656));
#97125=CARTESIAN_POINT('Ctrl Pts',(19.2488814384357,9.24176762102788,-7.34599960699894));
#97126=CARTESIAN_POINT('Ctrl Pts',(19.4051985522719,11.5944628332931,-2.28718014002714));
#97127=CARTESIAN_POINT('Ctrl Pts',(19.560856029607,11.3624302638596,3.29440256703827));
#97128=CARTESIAN_POINT('Ctrl Pts',(19.7170279013492,8.59111746859576,8.14848688572577));
#97129=CARTESIAN_POINT('Ctrl Pts',(19.8732130134576,3.8966145319634,11.1987915952599));
#97130=CARTESIAN_POINT('Ctrl Pts',(20.0295862073395,-1.68030661482981,11.7400692616394));
#97131=CARTESIAN_POINT('Ctrl Pts',(20.1861778729395,-6.8875480967494,9.68884223286411));
#97132=CARTESIAN_POINT('Ctrl Pts',(20.3427366995498,-10.5767665435211,5.41053330586961));
#97133=CARTESIAN_POINT('Ctrl Pts',(20.447527115044,-11.450015111617,1.84158505298324));
#97134=CARTESIAN_POINT('Ctrl Pts',(20.4995937278547,-11.4567032481648,-0.0201481587004812));
#97135=CARTESIAN_POINT('Ctrl Pts',(0.840394518298377,9.8112024191675,-0.00670618228483209));
#97136=CARTESIAN_POINT('Ctrl Pts',(0.885552519579505,9.80540171773232,1.60799749190895));
#97137=CARTESIAN_POINT('Ctrl Pts',(0.974750578127202,9.0576922562742,4.64438287980197));
#97138=CARTESIAN_POINT('Ctrl Pts',(1.10934238128961,5.89424784709291,8.3269760036482));
#97139=CARTESIAN_POINT('Ctrl Pts',(1.24355928276938,1.42507842855297,10.0798499360501));
#97140=CARTESIAN_POINT('Ctrl Pts',(1.37796108194799,-3.36571918358726,9.61929687754925));
#97141=CARTESIAN_POINT('Ctrl Pts',(1.51222657698763,-7.40286551116007,6.99470771718013));
#97142=CARTESIAN_POINT('Ctrl Pts',(1.64664791909928,-9.78837229914064,2.81815601860371));
#97143=CARTESIAN_POINT('Ctrl Pts',(1.78074561536888,-9.98898798636914,-1.99102191145044));
#97144=CARTESIAN_POINT('Ctrl Pts',(1.91555781226548,-7.96044407001117,-6.35391906224498));
#97145=CARTESIAN_POINT('Ctrl Pts',(2.04876863167595,-4.15521006841318,-9.29963433652184));
#97146=CARTESIAN_POINT('Ctrl Pts',(2.18548090920051,0.577631937284577,-10.169672800332));
#97147=CARTESIAN_POINT('Ctrl Pts',(2.31485557822428,5.18201744899307,-8.77015906126499));
#97148=CARTESIAN_POINT('Ctrl Pts',(2.45924280692048,8.63054056692016,-5.41297393495632));
#97149=CARTESIAN_POINT('Ctrl Pts',(2.57265305016202,10.15324509706,-0.847239260661916));
#97150=CARTESIAN_POINT('Ctrl Pts',(2.75655298519099,9.4102732574346,3.91072658414708));
#97151=CARTESIAN_POINT('Ctrl Pts',(2.93071565980367,6.56718797325696,7.7923694311073));
#97152=CARTESIAN_POINT('Ctrl Pts',(3.12658638027203,1.77805349278155,10.1852620677513));
#97153=CARTESIAN_POINT('Ctrl Pts',(3.34119969408586,-4.21044791581097,9.62486450025235));
#97154=CARTESIAN_POINT('Ctrl Pts',(3.5758276553806,-9.11166252069733,5.24318208444361));
#97155=CARTESIAN_POINT('Ctrl Pts',(3.81038380928619,-10.4439097069757,-1.19065991693002));
#97156=CARTESIAN_POINT('Ctrl Pts',(4.0451423272918,-7.70232284178181,-7.16496362076518));
#97157=CARTESIAN_POINT('Ctrl Pts',(4.27999813823747,-1.94023943533083,-10.3469623541626));
#97158=CARTESIAN_POINT('Ctrl Pts',(4.48890492429656,3.8556110503865,-9.57499253837833));
#97159=CARTESIAN_POINT('Ctrl Pts',(4.67179748834899,7.78584865357542,-6.51004394062785));
#97160=CARTESIAN_POINT('Ctrl Pts',(4.82863972732285,9.77698041904427,-2.73530434634081));
#97161=CARTESIAN_POINT('Ctrl Pts',(5.0117133577872,10.09260835835,2.24386005062187));
#97162=CARTESIAN_POINT('Ctrl Pts',(5.22107968543367,7.45508083801071,7.4768077396953));
#97163=CARTESIAN_POINT('Ctrl Pts',(5.45681647748818,1.55619885325388,10.4515425114258));
#97164=CARTESIAN_POINT('Ctrl Pts',(5.69276964571786,-4.95793332420886,9.34248767908207));
#97165=CARTESIAN_POINT('Ctrl Pts',(5.92894764174431,-9.54706610725953,4.57634563628634));
#97166=CARTESIAN_POINT('Ctrl Pts',(6.16536813622835,-10.4097935511739,-1.98854928432125));
#97167=CARTESIAN_POINT('Ctrl Pts',(6.4020422586417,-7.20166324917165,-7.79263732418621));
#97168=CARTESIAN_POINT('Ctrl Pts',(6.59949026276999,-2.17429698465326,-10.092758157656));
#97169=CARTESIAN_POINT('Ctrl Pts',(6.75759161856712,2.08433598343559,-9.88295467395817));
#97170=CARTESIAN_POINT('Ctrl Pts',(6.9157878368503,6.07347841979099,-8.36898824279205));
#97171=CARTESIAN_POINT('Ctrl Pts',(7.1137119010795,9.76828400366959,-4.24027621390453));
#97172=CARTESIAN_POINT('Ctrl Pts',(7.35152456967961,10.3924428604999,2.39684477307773));
#97173=CARTESIAN_POINT('Ctrl Pts',(7.58965789216565,6.94580978226224,8.10535272771152));
#97174=CARTESIAN_POINT('Ctrl Pts',(7.82811381443578,0.775522719167843,10.662626855712));
#97175=CARTESIAN_POINT('Ctrl Pts',(8.06691045556968,-5.71462403419679,9.05160752136358));
#97176=CARTESIAN_POINT('Ctrl Pts',(8.30606116330518,-9.99419182866903,3.89729828508907));
#97177=CARTESIAN_POINT('Ctrl Pts',(8.50564975817593,-10.301053359501,-1.68557337935384));
#97178=CARTESIAN_POINT('Ctrl Pts',(8.66551277345512,-8.53125361604988,-5.6165326975031));
#97179=CARTESIAN_POINT('Ctrl Pts',(8.82550163905307,-5.63343798709349,-8.81248942392093));
#97180=CARTESIAN_POINT('Ctrl Pts',(9.02572387901138,-0.377112405932923,
-10.7702099814649));
#97181=CARTESIAN_POINT('Ctrl Pts',(9.23964628508325,5.37806574910098,-9.10510040701057));
#97182=CARTESIAN_POINT('Ctrl Pts',(9.42709466339725,8.89239633905225,-5.40205281095219));
#97183=CARTESIAN_POINT('Ctrl Pts',(9.58794944648292,10.3412852051172,-1.26764760710221));
#97184=CARTESIAN_POINT('Ctrl Pts',(9.73109312372931,9.99778113623362,2.61357300057332));
#97185=CARTESIAN_POINT('Ctrl Pts',(9.89229087385157,8.15364281688216,6.53990392141035));
#97186=CARTESIAN_POINT('Ctrl Pts',(10.0536805462786,4.75573838903045,9.44164371222992));
#97187=CARTESIAN_POINT('Ctrl Pts',(10.2332520784286,-0.0299529409807728,
10.4652778834182));
#97188=CARTESIAN_POINT('Ctrl Pts',(10.3950687359733,-4.33689811382311,9.54254148160714));
#97189=CARTESIAN_POINT('Ctrl Pts',(10.5570818172104,-7.88545311500811,6.92103924802403));
#97190=CARTESIAN_POINT('Ctrl Pts',(10.7463390558374,-10.414668932124,2.42833144703078));
#97191=CARTESIAN_POINT('Ctrl Pts',(10.9629699253934,-10.3096478902391,-3.63548669311155));
#97192=CARTESIAN_POINT('Ctrl Pts',(11.207157532618,-6.14495684043231,-9.06547916791598));
#97193=CARTESIAN_POINT('Ctrl Pts',(11.4518252038093,0.438548929035689,-10.9646249539477));
#97194=CARTESIAN_POINT('Ctrl Pts',(11.6969823136692,6.87865568211547,-8.57922988332477));
#97195=CARTESIAN_POINT('Ctrl Pts',(11.9426382962662,10.6502059987716,-2.82316358352909));
#97196=CARTESIAN_POINT('Ctrl Pts',(12.1887977605246,10.2676274637117,4.05994586492189));
#97197=CARTESIAN_POINT('Ctrl Pts',(12.4354709555491,5.86080066266984,9.38613385806551));
#97198=CARTESIAN_POINT('Ctrl Pts',(12.6551953046859,-0.109975039867466,
10.8640910801617));
#97199=CARTESIAN_POINT('Ctrl Pts',(12.8477989586744,-5.14194189665667,9.37452435506929));
#97200=CARTESIAN_POINT('Ctrl Pts',(13.0131218263297,-8.55543065539852,6.44200174199404));
#97201=CARTESIAN_POINT('Ctrl Pts',(13.1786832680645,-10.4622549707042,2.35527172510316));
#97202=CARTESIAN_POINT('Ctrl Pts',(13.3444852793881,-10.5220007104345,-2.15915681205131));
#97203=CARTESIAN_POINT('Ctrl Pts',(13.5105288776343,-8.71433212967542,-6.30395785253688));
#97204=CARTESIAN_POINT('Ctrl Pts',(13.662956387324,-5.63744684102453,-9.09082112151706));
#97205=CARTESIAN_POINT('Ctrl Pts',(13.8017063001416,-2.14229738687632,-10.4225698278804));
#97206=CARTESIAN_POINT('Ctrl Pts',(13.9683923393898,2.34877791247678,-10.6428567220425));
#97207=CARTESIAN_POINT('Ctrl Pts',(14.1770945402735,7.66388977684096,-8.22094702734011));
#97208=CARTESIAN_POINT('Ctrl Pts',(14.4280953126858,11.068982097841,-2.06146913677415));
#97209=CARTESIAN_POINT('Ctrl Pts',(14.679663690643,10.1548744665846,4.92137235826369));
#97210=CARTESIAN_POINT('Ctrl Pts',(14.9318023145324,5.25763196840611,10.0165288092755));
#97211=CARTESIAN_POINT('Ctrl Pts',(15.1564310783341,-0.942520850929141,
11.0677083375238));
#97212=CARTESIAN_POINT('Ctrl Pts',(15.3533633298778,-5.95905978015328,9.16595882332264));
#97213=CARTESIAN_POINT('Ctrl Pts',(15.5224192741083,-9.21737896803036,5.91650325731429));
#97214=CARTESIAN_POINT('Ctrl Pts',(15.6917292680821,-10.850427368977,1.6027367108997));
#97215=CARTESIAN_POINT('Ctrl Pts',(15.8613012109163,-10.5660287731456,-3.00545159510626));
#97216=CARTESIAN_POINT('Ctrl Pts',(16.0311313871158,-8.40721701333872,-7.09661446390494));
#97217=CARTESIAN_POINT('Ctrl Pts',(16.2012245630604,-4.75238379045116,-9.94086992193184));
#97218=CARTESIAN_POINT('Ctrl Pts',(16.3715791736397,-0.242748863921299,
-11.0351697210793));
#97219=CARTESIAN_POINT('Ctrl Pts',(16.5421999866943,4.32073643703397,-10.1711459420049));
#97220=CARTESIAN_POINT('Ctrl Pts',(16.7415533331513,8.77708241140647,-7.06604653174035));
#97221=CARTESIAN_POINT('Ctrl Pts',(16.9698445054398,11.4526883383421,-1.2620410011127));
#97222=CARTESIAN_POINT('Ctrl Pts',(17.2272005571437,9.98569686135026,5.79875321887713));
#97223=CARTESIAN_POINT('Ctrl Pts',(17.4852834652622,4.60144346399131,10.6224289494326));
#97224=CARTESIAN_POINT('Ctrl Pts',(17.7221264018559,-2.00689161588762,11.2411048053495));
#97225=CARTESIAN_POINT('Ctrl Pts',(17.9385221855771,-7.30110778520626,8.60120368104034));
#97226=CARTESIAN_POINT('Ctrl Pts',(18.1317864645908,-10.4529103768998,4.29265039185786));
#97227=CARTESIAN_POINT('Ctrl Pts',(18.3353557032759,-11.2787530887185,-0.972196076855361));
#97228=CARTESIAN_POINT('Ctrl Pts',(18.461467953364,-9.58587761179443,-6.04767973256785));
#97229=CARTESIAN_POINT('Ctrl Pts',(18.6222145537073,-5.74771983808596,-9.7875564324453));
#97230=CARTESIAN_POINT('Ctrl Pts',(18.7664485808866,-0.614496977722204,
-11.3476121811775));
#97231=CARTESIAN_POINT('Ctrl Pts',(18.919057129735,4.6689269100397,-10.37770030444));
#97232=CARTESIAN_POINT('Ctrl Pts',(19.0679708368727,8.92327404926781,-7.0853647814176));
#97233=CARTESIAN_POINT('Ctrl Pts',(19.2188596216407,11.1944683039804,-2.20224801907994));
#97234=CARTESIAN_POINT('Ctrl Pts',(19.3691524522802,10.9705879762662,3.18723371060556));
#97235=CARTESIAN_POINT('Ctrl Pts',(19.5199850143116,8.29418732152164,7.87525299435256));
#97236=CARTESIAN_POINT('Ctrl Pts',(19.6708643849559,3.75892317031939,10.8228124930193));
#97237=CARTESIAN_POINT('Ctrl Pts',(19.8219912701959,-1.63037658945895,11.3451400693921));
#97238=CARTESIAN_POINT('Ctrl Pts',(19.9733148456315,-6.66397468925673,9.36442000366302));
#97239=CARTESIAN_POINT('Ctrl Pts',(20.1247714457631,-10.2313788447333,5.22459154891526));
#97240=CARTESIAN_POINT('Ctrl Pts',(20.2259938430529,-11.0759875132312,1.77747672674462));
#97241=CARTESIAN_POINT('Ctrl Pts',(20.2764796593326,-11.0824725909955,-0.0277323278312897));
#97242=CARTESIAN_POINT('Ctrl Pts',(1.5069621239122,10.1062642497049,-0.0242879192054315));
#97243=CARTESIAN_POINT('Ctrl Pts',(1.55334346900726,10.1003064055261,1.63415856235628));
#97244=CARTESIAN_POINT('Ctrl Pts',(1.64530857322812,9.3301337990831,4.76502605162024));
#97245=CARTESIAN_POINT('Ctrl Pts',(1.78368715348376,6.07563011846298,8.5500818783867));
#97246=CARTESIAN_POINT('Ctrl Pts',(1.92166086015211,1.48240340871853,10.3526479088268));
#97247=CARTESIAN_POINT('Ctrl Pts',(2.05964680268286,-3.43668383608774,9.87845827712341));
#97248=CARTESIAN_POINT('Ctrl Pts',(2.19738578920598,-7.57775083240144,7.18602209416567));
#97249=CARTESIAN_POINT('Ctrl Pts',(2.33514751881056,-10.0221669614262,2.90512444626086));
#97250=CARTESIAN_POINT('Ctrl Pts',(2.47245339717927,-10.2269687721166,-2.01903352888235));
#97251=CARTESIAN_POINT('Ctrl Pts',(2.61035542825578,-8.15142492455985,-6.48177840056761));
#97252=CARTESIAN_POINT('Ctrl Pts',(2.74649771620373,-4.26209165119445,-9.49194667508545));
#97253=CARTESIAN_POINT('Ctrl Pts',(2.8860755063246,0.570107557856309,-10.379365507633));
#97254=CARTESIAN_POINT('Ctrl Pts',(3.01804263479664,5.26675673347687,-8.95193129729442));
#97255=CARTESIAN_POINT('Ctrl Pts',(3.16518084822296,8.78023376225081,-5.52933408693512));
#97256=CARTESIAN_POINT('Ctrl Pts',(3.28065563177323,10.3304739499724,-0.8814684930199));
#97257=CARTESIAN_POINT('Ctrl Pts',(3.46733327630008,9.57406157984235,3.94707456960536));
#97258=CARTESIAN_POINT('Ctrl Pts',(3.64442432694637,6.68527681753859,7.89475514720481));
#97259=CARTESIAN_POINT('Ctrl Pts',(3.84299745953732,1.8275257206148,10.318269563343));
#97260=CARTESIAN_POINT('Ctrl Pts',(4.06042336981818,-4.23805330991327,9.75068525772592));
#97261=CARTESIAN_POINT('Ctrl Pts',(4.29761943218592,-9.19209258466678,5.31824870856728));
#97262=CARTESIAN_POINT('Ctrl Pts',(4.53437161274713,-10.5350051791128,-1.17556335380542));
#97263=CARTESIAN_POINT('Ctrl Pts',(4.7708980371129,-7.77097759235335,-7.19441649509308));
#97264=CARTESIAN_POINT('Ctrl Pts',(5.00711660622112,-1.97462556771702,-10.3930919627927));
#97265=CARTESIAN_POINT('Ctrl Pts',(5.21686324657125,3.84430502097436,-9.61644715696625));
#97266=CARTESIAN_POINT('Ctrl Pts',(5.40022325876364,7.78412965343201,-6.54316740517288));
#97267=CARTESIAN_POINT('Ctrl Pts',(5.55728136173065,9.77755506434019,-2.7630113948148));
#97268=CARTESIAN_POINT('Ctrl Pts',(5.74039202752718,10.0925810161338,2.21725805512244));
#97269=CARTESIAN_POINT('Ctrl Pts',(5.94949375129097,7.45693493819098,7.44288523114148));
#97270=CARTESIAN_POINT('Ctrl Pts',(6.18451777235544,1.57504642791826,10.4069276145566));
#97271=CARTESIAN_POINT('Ctrl Pts',(6.41934409059153,-4.9076259651148,9.30134643286956));
#97272=CARTESIAN_POINT('Ctrl Pts',(6.65398123255926,-9.46546493887723,4.56502892019478));
#97273=CARTESIAN_POINT('Ctrl Pts',(6.88844862201365,-10.3192263205529,-1.94583617559358));
#97274=CARTESIAN_POINT('Ctrl Pts',(7.12275735358216,-7.14154658054596,-7.69098867775806));
#97275=CARTESIAN_POINT('Ctrl Pts',(7.31789383154067,-2.17248871763666,-9.96277635107079));
#97276=CARTESIAN_POINT('Ctrl Pts',(7.47393908444266,2.03065753434173,-9.75540780747296));
#97277=CARTESIAN_POINT('Ctrl Pts',(7.6299434805996,5.9644634282179,-8.26211446422332));
#97278=CARTESIAN_POINT('Ctrl Pts',(7.82487598081776,9.60233065552826,-4.1948354558297));
#97279=CARTESIAN_POINT('Ctrl Pts',(8.05869462024724,10.2141341233479,2.33092319144744));
#97280=CARTESIAN_POINT('Ctrl Pts',(8.29242713293129,6.82975323685128,7.93295582313208));
#97281=CARTESIAN_POINT('Ctrl Pts',(8.52608518374186,0.782992881230091,10.4371166486048));
#97282=CARTESIAN_POINT('Ctrl Pts',(8.75968779881235,-5.56546712895628,8.85948026402679));
#97283=CARTESIAN_POINT('Ctrl Pts',(8.99324390420264,-9.74358840205274,3.82461799473537));
#97284=CARTESIAN_POINT('Ctrl Pts',(9.18785311736504,-10.0413667217101,-1.61886906842269));
#97285=CARTESIAN_POINT('Ctrl Pts',(9.34353133992201,-8.31767691397426,-5.4467288803861));
#97286=CARTESIAN_POINT('Ctrl Pts',(9.49920792635024,-5.49774110980979,-8.55637463672939));
#97287=CARTESIAN_POINT('Ctrl Pts',(9.69380443073233,-0.388675826148052,
-10.4577620504452));
#97288=CARTESIAN_POINT('Ctrl Pts',(9.90138990968947,5.19543696900351,-8.84060317707353));
#97289=CARTESIAN_POINT('Ctrl Pts',(10.0830435383244,8.60064437435068,-5.25171837777729));
#97290=CARTESIAN_POINT('Ctrl Pts',(10.2387643960254,10.0028444638209,-1.24914248103297));
#97291=CARTESIAN_POINT('Ctrl Pts',(10.37720298638,9.67023254520016,2.50437837408168));
#97292=CARTESIAN_POINT('Ctrl Pts',(10.5329676769268,7.88804604937092,6.29825863224296));
#97293=CARTESIAN_POINT('Ctrl Pts',(10.6887607398496,4.60750562412172,9.0987655073134));
#97294=CARTESIAN_POINT('Ctrl Pts',(10.8619109109484,-0.00703355469036902,
10.0852618131503));
#97295=CARTESIAN_POINT('Ctrl Pts',(11.0177828805925,-4.15564321735493,9.19600425219595));
#97296=CARTESIAN_POINT('Ctrl Pts',(11.1737001608909,-7.57035238191842,6.67287428521118));
#97297=CARTESIAN_POINT('Ctrl Pts',(11.3556582804353,-10.0015525960454,2.35319965804952));
#97298=CARTESIAN_POINT('Ctrl Pts',(11.5636962223343,-9.89945473807122,-3.46995082097515));
#97299=CARTESIAN_POINT('Ctrl Pts',(11.7978709095172,-5.90444684023231,-8.6762915307363));
#97300=CARTESIAN_POINT('Ctrl Pts',(12.0321903548044,0.400833060828008,-10.4937295217811));
#97301=CARTESIAN_POINT('Ctrl Pts',(12.2666675462662,6.55977924120225,-8.21100202194529));
#97302=CARTESIAN_POINT('Ctrl Pts',(12.5013204486353,10.1611836230131,-2.71214958148474));
#97303=CARTESIAN_POINT('Ctrl Pts',(12.7361586173256,9.79488883170482,3.85415353952862));
#97304=CARTESIAN_POINT('Ctrl Pts',(12.9711981732529,5.59499649365486,8.92819941309873));
#97305=CARTESIAN_POINT('Ctrl Pts',(13.1803153631814,-0.0875873623257469,
10.3336777025827));
#97306=CARTESIAN_POINT('Ctrl Pts',(13.3634371883564,-4.8715902948797,8.91705557662938));
#97307=CARTESIAN_POINT('Ctrl Pts',(13.520505724078,-8.11433355257515,6.13074937900602));
#97308=CARTESIAN_POINT('Ctrl Pts',(13.677682974814,-9.92426658237873,2.2509045507049));
#97309=CARTESIAN_POINT('Ctrl Pts',(13.8349734047848,-9.98057122548719,-2.0316952253054));
#97310=CARTESIAN_POINT('Ctrl Pts',(13.9923803080536,-8.2666973670815,-5.96072336484286));
#97311=CARTESIAN_POINT('Ctrl Pts',(14.1367835222368,-5.35165095933992,-8.6005816687047));
#97312=CARTESIAN_POINT('Ctrl Pts',(14.2681481522955,-2.04257932770994,-9.86129725114235));
#97313=CARTESIAN_POINT('Ctrl Pts',(14.4258813335358,2.20726207074819,-10.0695922061582));
#97314=CARTESIAN_POINT('Ctrl Pts',(14.6232328885067,7.23285997487796,-7.77868641881626));
#97315=CARTESIAN_POINT('Ctrl Pts',(14.8603648356027,10.4488462542502,-1.9592940246166));
#97316=CARTESIAN_POINT('Ctrl Pts',(15.0978152410641,9.58510242747451,4.63131300952894));
#97317=CARTESIAN_POINT('Ctrl Pts',(15.3355945418123,4.96624008693659,9.43556607275977));
#97318=CARTESIAN_POINT('Ctrl Pts',(15.5472659450391,-0.876115585652837,
10.4252628531268));
#97319=CARTESIAN_POINT('Ctrl Pts',(15.7327007535624,-5.59959226313437,8.63432403909379));
#97320=CARTESIAN_POINT('Ctrl Pts',(15.8918077602256,-8.6659356307169,5.57596084701422));
#97321=CARTESIAN_POINT('Ctrl Pts',(16.0510831684788,-10.2019230830579,1.51791718343275));
#97322=CARTESIAN_POINT('Ctrl Pts',(16.2105256124773,-9.9342900388101,-2.81488948283342));
#97323=CARTESIAN_POINT('Ctrl Pts',(16.3701404794229,-7.90520615830692,-6.65973809987124));
#97324=CARTESIAN_POINT('Ctrl Pts',(16.5299308091608,-4.47173190491229,-9.3315218483862));
#97325=CARTESIAN_POINT('Ctrl Pts',(16.689895927779,-0.237156293344815,-10.3588395266908));
#97326=CARTESIAN_POINT('Ctrl Pts',(16.8500471787606,4.04617623445192,-9.547731017281));
#97327=CARTESIAN_POINT('Ctrl Pts',(17.0370951498213,8.22725055971312,-6.63413010802371));
#97328=CARTESIAN_POINT('Ctrl Pts',(17.2512080029201,10.7361609685627,-1.19069424451522));
#97329=CARTESIAN_POINT('Ctrl Pts',(17.4924479420939,9.36052958618687,5.42776286527152));
#97330=CARTESIAN_POINT('Ctrl Pts',(17.7342626534981,4.31561709585493,9.94660037034397));
#97331=CARTESIAN_POINT('Ctrl Pts',(17.9560677398241,-1.87318360886642,10.5258988523837));
#97332=CARTESIAN_POINT('Ctrl Pts',(18.1586777030311,-6.82953792919343,8.0537380447665));
#97333=CARTESIAN_POINT('Ctrl Pts',(18.3395298833531,-9.77919804704876,4.02216254357936));
#97334=CARTESIAN_POINT('Ctrl Pts',(18.5300740388948,-10.5517653438536,-0.90606004736438));
#97335=CARTESIAN_POINT('Ctrl Pts',(18.64805587877,-8.96809223471218,-5.6541368174137));
#97336=CARTESIAN_POINT('Ctrl Pts',(18.7984112754343,-5.37797595348926,-9.15197600853212));
#97337=CARTESIAN_POINT('Ctrl Pts',(18.9333053939666,-0.577353141871393,
-10.6109679620998));
#97338=CARTESIAN_POINT('Ctrl Pts',(19.0760117727805,4.36310404586792,-9.7039080890023));
#97339=CARTESIAN_POINT('Ctrl Pts',(19.2152458180293,8.34073515999311,-6.62558477275444));
#97340=CARTESIAN_POINT('Ctrl Pts',(19.3563124474702,10.4639838983962,-2.06055455074961));
#97341=CARTESIAN_POINT('Ctrl Pts',(19.4968066664293,10.2545994787298,2.97769872115227));
#97342=CARTESIAN_POINT('Ctrl Pts',(19.6377988698527,7.75298183285304,7.35915813897839));
#97343=CARTESIAN_POINT('Ctrl Pts',(19.7788087536973,3.51396003949119,10.1150854546748));
#97344=CARTESIAN_POINT('Ctrl Pts',(19.9200865166857,-1.5228146944367,10.6014255500044));
#97345=CARTESIAN_POINT('Ctrl Pts',(20.0614293133846,-6.22707474371873,8.75402786138048));
#97346=CARTESIAN_POINT('Ctrl Pts',(20.2031253543693,-9.56103685363943,4.87911794644152));
#97347=CARTESIAN_POINT('Ctrl Pts',(20.2974622713297,-10.3504309907549,1.6673870870399));
#97348=CARTESIAN_POINT('Ctrl Pts',(20.3448886687027,-10.3565230755762,-0.028427069738528));
#97349=CARTESIAN_POINT('Ctrl Pts',(1.83818426640986,10.8689493708656,-0.0308112345521901));
#97350=CARTESIAN_POINT('Ctrl Pts',(1.88776189648677,10.8625809528271,1.74192403210919));
#97351=CARTESIAN_POINT('Ctrl Pts',(1.98696005135264,10.0340075995239,5.11962447490025));
#97352=CARTESIAN_POINT('Ctrl Pts',(2.13551416471739,6.53596609625885,9.18048144916341));
#97353=CARTESIAN_POINT('Ctrl Pts',(2.28385549019855,1.60092055185801,11.1212281400739));
#97354=CARTESIAN_POINT('Ctrl Pts',(2.43201757162897,-3.6820951696278,10.6096556943922));
#97355=CARTESIAN_POINT('Ctrl Pts',(2.57990783088367,-8.12742516058339,7.72019468550292));
#97356=CARTESIAN_POINT('Ctrl Pts',(2.72773989858082,-10.7503724424901,3.12577566618505));
#97357=CARTESIAN_POINT('Ctrl Pts',(2.87502614211072,-10.969712571133,-2.15572865673128));
#97358=CARTESIAN_POINT('Ctrl Pts',(3.02288074463859,-8.74423490665549,-6.94037080074683));
#97359=CARTESIAN_POINT('Ctrl Pts',(3.16878612908498,-4.57600120570609,-10.1660120144097));
#97360=CARTESIAN_POINT('Ctrl Pts',(3.31829567125103,0.599901256008977,-11.11609137723));
#97361=CARTESIAN_POINT('Ctrl Pts',(3.45958938695334,5.62820968933488,-9.58793407736161));
#97362=CARTESIAN_POINT('Ctrl Pts',(3.61704293708648,9.38747189660534,-5.92469929399861));
#97363=CARTESIAN_POINT('Ctrl Pts',(3.74056654439857,11.0455000317742,-0.9538859493391));
#97364=CARTESIAN_POINT('Ctrl Pts',(3.9398976454627,10.2365319010948,4.20107343062296));
#97365=CARTESIAN_POINT('Ctrl Pts',(4.12916837477669,7.15042126932385,8.42057304437813));
#97366=CARTESIAN_POINT('Ctrl Pts',(4.34103991393533,1.96602379561902,11.0048501470889));
#97367=CARTESIAN_POINT('Ctrl Pts',(4.5729306213578,-4.50201320676947,10.3996247365394));
#97368=CARTESIAN_POINT('Ctrl Pts',(4.8255857070546,-9.77799551649871,5.67675453717147));
#97369=CARTESIAN_POINT('Ctrl Pts',(5.07749033585182,-11.2056768141972,-1.23238566466435));
#97370=CARTESIAN_POINT('Ctrl Pts',(5.32887240299551,-8.26686359636807,-7.6286025326305));
#97371=CARTESIAN_POINT('Ctrl Pts',(5.57962526190281,-2.11347710892471,-11.0227160727275));
#97372=CARTESIAN_POINT('Ctrl Pts',(5.80201065073146,4.05562182529484,-10.1981135862017));
#97373=CARTESIAN_POINT('Ctrl Pts',(5.99619748242115,8.22765205976638,-6.94304765662431));
#97374=CARTESIAN_POINT('Ctrl Pts',(6.16238502036293,10.3365757371908,-2.94306233307449));
#97375=CARTESIAN_POINT('Ctrl Pts',(6.35597213040649,10.6690844793293,2.32209917177999));
#97376=CARTESIAN_POINT('Ctrl Pts',(6.57679779675907,7.88462429552231,7.8399572546674));
#97377=CARTESIAN_POINT('Ctrl Pts',(6.82464760372649,1.68122123786173,10.9642470927747));
#97378=CARTESIAN_POINT('Ctrl Pts',(7.0719359806289,-5.1449584383304,9.79849951504099));
#97379=CARTESIAN_POINT('Ctrl Pts',(7.31866327856874,-9.93634104403059,4.81715538296204));
#97380=CARTESIAN_POINT('Ctrl Pts',(7.56484307141959,-10.8310545876768,-2.01893420180603));
#97381=CARTESIAN_POINT('Ctrl Pts',(7.81047672182262,-7.49838634017914,-8.04079854736679));
#97382=CARTESIAN_POINT('Ctrl Pts',(8.0147315059415,-2.29677092419376,-10.4173489247643));
#97383=CARTESIAN_POINT('Ctrl Pts',(8.17786172927881,2.0970715104821,-10.2002860770181));
#97384=CARTESIAN_POINT('Ctrl Pts',(8.34081833458581,6.20607454866971,-8.64017166703644));
#97385=CARTESIAN_POINT('Ctrl Pts',(8.54419898417021,10.000471803415,-4.39575725264335));
#97386=CARTESIAN_POINT('Ctrl Pts',(8.78774561141104,10.6357859285607,2.40148995762388));
#97387=CARTESIAN_POINT('Ctrl Pts',(9.03078021376301,7.11527379626338,8.22542500490687));
#97388=CARTESIAN_POINT('Ctrl Pts',(9.27332878581485,0.837846907564282,10.8230720357878));
#97389=CARTESIAN_POINT('Ctrl Pts',(9.51539756520767,-5.74004007217375,9.18649736408127));
#97390=CARTESIAN_POINT('Ctrl Pts',(9.75697918017891,-10.0602275893844,3.97738562041968));
#97391=CARTESIAN_POINT('Ctrl Pts',(9.95792867482619,-10.3661161112419,-1.64326633591469));
#97392=CARTESIAN_POINT('Ctrl Pts',(10.1184478344858,-8.58857431044701,-5.58991834917576));
#97393=CARTESIAN_POINT('Ctrl Pts',(10.2788200862377,-5.683335003516,-8.79316631224028));
#97394=CARTESIAN_POINT('Ctrl Pts',(10.4790161508981,-0.426755680715147,
-10.7476973019787));
#97395=CARTESIAN_POINT('Ctrl Pts',(10.6921776353054,5.30667425331728,-9.08543831520305));
#97396=CARTESIAN_POINT('Ctrl Pts',(10.8784122755464,8.79717325481755,-5.40566075731209));
#97397=CARTESIAN_POINT('Ctrl Pts',(11.0378573747148,10.2323564000071,-1.30718768757403));
#97398=CARTESIAN_POINT('Ctrl Pts',(11.1794315307463,9.89171945814866,2.53120787155922));
#97399=CARTESIAN_POINT('Ctrl Pts',(11.3385508759767,8.07088824484368,6.40668023386538));
#97400=CARTESIAN_POINT('Ctrl Pts',(11.4974943772879,4.72338085120294,9.26303381412744));
#97401=CARTESIAN_POINT('Ctrl Pts',(11.6738835255329,0.0224914630507778,
10.2672914814035));
#97402=CARTESIAN_POINT('Ctrl Pts',(11.8324606855234,-4.19799457821475,9.36203711938622));
#97403=CARTESIAN_POINT('Ctrl Pts',(11.9908814020297,-7.6671319801918,6.797988448667));
#97404=CARTESIAN_POINT('Ctrl Pts',(12.1755152746382,-10.1334735184091,2.41440828085528));
#97405=CARTESIAN_POINT('Ctrl Pts',(12.3862701364914,-10.0282559850612,-3.48472158440349));
#97406=CARTESIAN_POINT('Ctrl Pts',(12.6230299247251,-5.98748195420321,-8.7472018168645));
#97407=CARTESIAN_POINT('Ctrl Pts',(12.859465524537,0.37524583457908,-10.579038475418));
#97408=CARTESIAN_POINT('Ctrl Pts',(13.0955874024424,6.57663912099642,-8.2783325277854));
#97409=CARTESIAN_POINT('Ctrl Pts',(13.3314131098248,10.1942562826981,-2.75087923652243));
#97410=CARTESIAN_POINT('Ctrl Pts',(13.5669515207943,9.82478241877411,3.83487919978063));
#97411=CARTESIAN_POINT('Ctrl Pts',(13.8022183194738,5.61919167439339,8.91245356687083));
#97412=CARTESIAN_POINT('Ctrl Pts',(14.0111170136416,-0.0578387583680794,
10.3146871657184));
#97413=CARTESIAN_POINT('Ctrl Pts',(14.1937410470241,-4.82856420086894,8.9012331076977));
#97414=CARTESIAN_POINT('Ctrl Pts',(14.350172686012,-8.05780235173047,6.12577966918914));
#97415=CARTESIAN_POINT('Ctrl Pts',(14.506503362215,-9.85743405856432,2.26657374520578));
#97416=CARTESIAN_POINT('Ctrl Pts',(14.662737409681,-9.91277321911816,-1.98729168662078));
#97417=CARTESIAN_POINT('Ctrl Pts',(14.8188789169398,-8.21212706834228,-5.88449319471934));
#97418=CARTESIAN_POINT('Ctrl Pts',(14.9619297947965,-5.32400842064335,-8.49923201713043));
#97419=CARTESIAN_POINT('Ctrl Pts',(15.0919132392097,-2.04965056788055,-9.74644660641511));
#97420=CARTESIAN_POINT('Ctrl Pts',(15.2478333215524,2.15143905872322,-9.95199811185607));
#97421=CARTESIAN_POINT('Ctrl Pts',(15.4426246944657,7.11126846897201,-7.68925041226127));
#97422=CARTESIAN_POINT('Ctrl Pts',(15.6762169225839,10.2774005373863,-1.95566702569206));
#97423=CARTESIAN_POINT('Ctrl Pts',(15.909663704702,9.42624261870193,4.52362470256974));
#97424=CARTESIAN_POINT('Ctrl Pts',(16.1429778981499,4.89257476540304,9.23627484965717));
#97425=CARTESIAN_POINT('Ctrl Pts',(16.3502681848699,-0.829186051812911,
10.2038045922452));
#97426=CARTESIAN_POINT('Ctrl Pts',(16.5315794164556,-5.44734383968922,8.45205581404979));
#97427=CARTESIAN_POINT('Ctrl Pts',(16.6869491325359,-8.44132728453901,5.46511601110685));
#97428=CARTESIAN_POINT('Ctrl Pts',(16.8422824860369,-9.93878585482269,1.50724672168229));
#97429=CARTESIAN_POINT('Ctrl Pts',(16.9975846873159,-9.67755952490929,-2.71305977140622));
#97430=CARTESIAN_POINT('Ctrl Pts',(17.1528587616045,-7.70313312175431,-6.45315215757489));
#97431=CARTESIAN_POINT('Ctrl Pts',(17.3081114703888,-4.36678293396964,-9.04865359635369));
#97432=CARTESIAN_POINT('Ctrl Pts',(17.4633433266442,-0.257307507931174,
-10.0450555316724));
#97433=CARTESIAN_POINT('Ctrl Pts',(17.6185664673369,3.89412154725938,-9.25838762996026));
#97434=CARTESIAN_POINT('Ctrl Pts',(17.7996358527774,7.94134476011658,-6.43722851335476));
#97435=CARTESIAN_POINT('Ctrl Pts',(18.006594507299,10.364912084505,-1.17513016360907));
#97436=CARTESIAN_POINT('Ctrl Pts',(18.2393437052062,9.03587592715122,5.21087315758684));
#97437=CARTESIAN_POINT('Ctrl Pts',(18.4722791560659,4.17530017099195,9.56114196894378));
#97438=CARTESIAN_POINT('Ctrl Pts',(18.685483449533,-1.77503968503135,10.1181556762285));
#97439=CARTESIAN_POINT('Ctrl Pts',(18.880106854292,-6.53372445406436,7.74112266949097));
#97440=CARTESIAN_POINT('Ctrl Pts',(19.0533284606598,-9.36098152271742,3.88031745665509));
#97441=CARTESIAN_POINT('Ctrl Pts',(19.2361266589478,-10.1000769718,-0.848911211642665));
#97442=CARTESIAN_POINT('Ctrl Pts',(19.3489763573003,-8.58507867110896,-5.39153275737696));
#97443=CARTESIAN_POINT('Ctrl Pts',(19.4926766226755,-5.15305056101582,-8.73333966878052));
#97444=CARTESIAN_POINT('Ctrl Pts',(19.6214820850813,-0.568968113951337,
-10.1266503521605));
#97445=CARTESIAN_POINT('Ctrl Pts',(19.7576303738871,4.144475299569,-9.26047530960638));
#97446=CARTESIAN_POINT('Ctrl Pts',(19.8903381036552,7.93547183918914,-6.32599142257229));
#97447=CARTESIAN_POINT('Ctrl Pts',(20.024680461408,9.95714380136737,-1.97832471792147));
#97448=CARTESIAN_POINT('Ctrl Pts',(20.1583550467776,9.75736223240569,2.81574382815119));
#97449=CARTESIAN_POINT('Ctrl Pts',(20.2923937974737,7.37877459907573,6.98054580469578));
#97450=CARTESIAN_POINT('Ctrl Pts',(20.4263199844727,3.35188564930949,9.59874115052656));
#97451=CARTESIAN_POINT('Ctrl Pts',(20.560425364838,-1.42837773210827,10.0584164488272));
#97452=CARTESIAN_POINT('Ctrl Pts',(20.6943868066463,-5.88919751845155,8.30912295420081));
#97453=CARTESIAN_POINT('Ctrl Pts',(20.8287698213737,-9.04785423569596,4.63223803957308));
#97454=CARTESIAN_POINT('Ctrl Pts',(20.9178530496044,-9.79467800620001,1.59976306232615));
#97455=CARTESIAN_POINT('Ctrl Pts',(20.9629606708448,-9.80047223620488,-0.0131391802037495));
#97456=CARTESIAN_POINT('Ctrl Pts',(1.5809870441838,11.4169386758616,-0.0216496558209534));
#97457=CARTESIAN_POINT('Ctrl Pts',(1.63289675206296,11.4102706943643,1.83447314990275));
#97458=CARTESIAN_POINT('Ctrl Pts',(1.73729284798262,10.5405348425062,5.39040289704493));
#97459=CARTESIAN_POINT('Ctrl Pts',(1.8933082281801,6.86421115644908,9.65429347040028));
#97460=CARTESIAN_POINT('Ctrl Pts',(2.04932475230953,1.67555195478847,11.6979359622337));
#97461=CARTESIAN_POINT('Ctrl Pts',(2.20512511369068,-3.8812787875302,11.1586878225894));
#97462=CARTESIAN_POINT('Ctrl Pts',(2.36072469806447,-8.55856555251663,8.11941596439485));
#97463=CARTESIAN_POINT('Ctrl Pts',(2.51630371286344,-11.3195400105841,3.28336209072214));
#97464=CARTESIAN_POINT('Ctrl Pts',(2.67136081404846,-11.5506449296019,-2.27719803269604));
#97465=CARTESIAN_POINT('Ctrl Pts',(2.82706597810207,-9.20692048539113,-7.31662279645037));
#97466=CARTESIAN_POINT('Ctrl Pts',(2.98076287682068,-4.81569331332354,-10.7149974591792));
#97467=CARTESIAN_POINT('Ctrl Pts',(3.13830732477856,0.638935692629033,-11.7165434272761));
#97468=CARTESIAN_POINT('Ctrl Pts',(3.28723251892036,5.93951699244716,-10.1055865581304));
#97469=CARTESIAN_POINT('Ctrl Pts',(3.45324044352558,9.90367736049909,-6.2433617525658));
#97470=CARTESIAN_POINT('Ctrl Pts',(3.58349680980263,11.6524189813092,-1.00031976365907));
#97471=CARTESIAN_POINT('Ctrl Pts',(3.79388045160135,10.7991398987405,4.44122959128948));
#97472=CARTESIAN_POINT('Ctrl Pts',(3.99355019295073,7.54252592952349,8.89267332393697));
#97473=CARTESIAN_POINT('Ctrl Pts',(4.21723559604996,2.06922068053357,11.6220329583823));
#97474=CARTESIAN_POINT('Ctrl Pts',(4.46207111387019,-4.76093494914438,10.9825998628467));
#97475=CARTESIAN_POINT('Ctrl Pts',(4.72893719312375,-10.334874453495,5.99419965381685));
#97476=CARTESIAN_POINT('Ctrl Pts',(4.99514679887966,-11.8437987505411,-1.30785848843795));
#97477=CARTESIAN_POINT('Ctrl Pts',(5.26084090744296,-8.73780244151131,-8.06924018541072));
#97478=CARTESIAN_POINT('Ctrl Pts',(5.52595750953483,-2.23133107764473,-11.6583422596195));
#97479=CARTESIAN_POINT('Ctrl Pts',(5.7611068176764,4.29279932288354,-10.7865607271241));
#97480=CARTESIAN_POINT('Ctrl Pts',(5.96652714516798,8.7064943800609,-7.34305887020326));
#97481=CARTESIAN_POINT('Ctrl Pts',(6.14235049354763,10.9378177637936,-3.11093327658175));
#97482=CARTESIAN_POINT('Ctrl Pts',(6.34717311281565,11.2897503542811,2.46018182270645));
#97483=CARTESIAN_POINT('Ctrl Pts',(6.58081017622451,8.34335570885647,8.29891791849555));
#97484=CARTESIAN_POINT('Ctrl Pts',(6.84309571117951,1.77811161543802,11.6055559975002));
#97485=CARTESIAN_POINT('Ctrl Pts',(7.10480193995066,-5.44689514012842,10.3716741505217));
#97486=CARTESIAN_POINT('Ctrl Pts',(7.3659363394261,-10.5184885864916,5.09901317667749));
#97487=CARTESIAN_POINT('Ctrl Pts',(7.62648869550098,-11.4655827108715,-2.13697521097448));
#97488=CARTESIAN_POINT('Ctrl Pts',(7.88646893283754,-7.93788982756581,-8.51098443842803));
#97489=CARTESIAN_POINT('Ctrl Pts',(8.1026212089916,-2.4326177345364,-11.0262083103435));
#97490=CARTESIAN_POINT('Ctrl Pts',(8.27527724919823,2.21799111278608,-10.7964225498402));
#97491=CARTESIAN_POINT('Ctrl Pts',(8.44773846159635,6.56691865522038,-9.14522106162279));
#97492=CARTESIAN_POINT('Ctrl Pts',(8.6629306742405,10.5818216065013,-4.65374125637833));
#97493=CARTESIAN_POINT('Ctrl Pts',(8.92058295804147,11.2539961301362,2.53794920615522));
#97494=CARTESIAN_POINT('Ctrl Pts',(9.17768234425578,7.52916588638302,8.69903847266077));
#97495=CARTESIAN_POINT('Ctrl Pts',(9.43418691040704,0.889964532955913,11.4461559338261));
#97496=CARTESIAN_POINT('Ctrl Pts',(9.69011268842353,-6.06506695109494,9.71534908612722));
#97497=CARTESIAN_POINT('Ctrl Pts',(9.94549168521195,-10.6318873005423,4.20842658922282));
#97498=CARTESIAN_POINT('Ctrl Pts',(10.1577958510016,-10.9546044353997,-1.73065225296835));
#97499=CARTESIAN_POINT('Ctrl Pts',(10.327383585701,-9.0765773666272,-5.90032179774202));
#97500=CARTESIAN_POINT('Ctrl Pts',(10.49677789506,-6.00767290500012,-9.28392549693938));
#97501=CARTESIAN_POINT('Ctrl Pts',(10.7081504461604,-0.457028090683516,
-11.3473051979206));
#97502=CARTESIAN_POINT('Ctrl Pts',(10.9331123366397,5.59420942624187,-9.59252532148522));
#97503=CARTESIAN_POINT('Ctrl Pts',(11.1296073081414,9.27704839612523,-5.70971854781571));
#97504=CARTESIAN_POINT('Ctrl Pts',(11.297786940236,10.7907142084956,-1.38653999583745));
#97505=CARTESIAN_POINT('Ctrl Pts',(11.4470487914226,10.4314326507295,2.66052368848947));
#97506=CARTESIAN_POINT('Ctrl Pts',(11.6147735026284,8.5119640671563,6.74573039814433));
#97507=CARTESIAN_POINT('Ctrl Pts',(11.7822558891056,4.98427451759871,9.75536146854628));
#97508=CARTESIAN_POINT('Ctrl Pts',(11.9680227641689,0.0331256487114618,
10.8127717293753));
#97509=CARTESIAN_POINT('Ctrl Pts',(12.1349843154738,-4.41056739519488,9.85946584683898));
#97510=CARTESIAN_POINT('Ctrl Pts',(12.3016942670706,-8.06126526847656,7.16083504228128));
#97511=CARTESIAN_POINT('Ctrl Pts',(12.4959220969932,-10.655623004286,2.54919301777192));
#97512=CARTESIAN_POINT('Ctrl Pts',(12.717489767947,-10.5442072791782,-3.65300085548494));
#97513=CARTESIAN_POINT('Ctrl Pts',(12.9662363807326,-6.29803981578373,-9.18160665973904));
#97514=CARTESIAN_POINT('Ctrl Pts',(13.214460617168,0.382489528166651,-11.1040129548448));
#97515=CARTESIAN_POINT('Ctrl Pts',(13.4621717586644,6.88816657569474,-8.68945672393844));
#97516=CARTESIAN_POINT('Ctrl Pts',(13.7093763702802,10.6796831715465,-2.89458716516783));
#97517=CARTESIAN_POINT('Ctrl Pts',(13.9560791595477,10.291740536784,4.00350012428347));
#97518=CARTESIAN_POINT('Ctrl Pts',(14.2022892176303,5.88962980452267,9.31674394387247));
#97519=CARTESIAN_POINT('Ctrl Pts',(14.4207087523392,-0.0465033974837142,
10.7820677674357));
#97520=CARTESIAN_POINT('Ctrl Pts',(14.6115180151071,-5.03098776215844,9.30489515804488));
#97521=CARTESIAN_POINT('Ctrl Pts',(14.7748574763112,-8.40269313292153,6.40659876167101));
#97522=CARTESIAN_POINT('Ctrl Pts',(14.9379888665339,-10.2803266780696,2.37931588593463));
#97523=CARTESIAN_POINT('Ctrl Pts',(15.1009157458048,-10.3377315800466,-2.05682724723024));
#97524=CARTESIAN_POINT('Ctrl Pts',(15.263638577978,-8.56506525302953,-6.11818660926039));
#97525=CARTESIAN_POINT('Ctrl Pts',(15.4126178905096,-5.55702315674806,-8.84107798464344));
#97526=CARTESIAN_POINT('Ctrl Pts',(15.5479084789727,-2.14891101096889,-10.1390596050238));
#97527=CARTESIAN_POINT('Ctrl Pts',(15.7101105471896,2.2215090845951,-10.3526814778452));
#97528=CARTESIAN_POINT('Ctrl Pts',(15.9125903919246,7.37675549081694,-7.99971492454468));
#97529=CARTESIAN_POINT('Ctrl Pts',(16.1551398067183,10.66316984791,-2.04563823051419));
#97530=CARTESIAN_POINT('Ctrl Pts',(16.3972724776516,9.77911126777587,4.67451911452633));
#97531=CARTESIAN_POINT('Ctrl Pts',(16.6389940080972,5.08114453646148,9.55608842508968));
#97532=CARTESIAN_POINT('Ctrl Pts',(16.8535101459097,-0.840131908612288,
10.5561550864893));
#97533=CARTESIAN_POINT('Ctrl Pts',(17.0409517630139,-5.61421615837297,8.7447801338398));
#97534=CARTESIAN_POINT('Ctrl Pts',(17.2014479827319,-8.70669146981356,5.65902412117622));
#97535=CARTESIAN_POINT('Ctrl Pts',(17.3617817749257,-10.2519259768557,1.57368476722833));
#97536=CARTESIAN_POINT('Ctrl Pts',(17.5219505321004,-9.98210887180923,-2.77878183638506));
#97537=CARTESIAN_POINT('Ctrl Pts',(17.6819601751567,-7.9471388192863,-6.63264401487525));
#97538=CARTESIAN_POINT('Ctrl Pts',(17.841813076855,-4.51175814935185,-9.30470904997924));
#97539=CARTESIAN_POINT('Ctrl Pts',(18.0015074983284,-0.284100670960046,
-10.3292985319853));
#97540=CARTESIAN_POINT('Ctrl Pts',(18.1610574640256,3.98286343161655,-9.5203859703373));
#97541=CARTESIAN_POINT('Ctrl Pts',(18.3470121213786,8.13897972179755,-6.62263664608639));
#97542=CARTESIAN_POINT('Ctrl Pts',(18.5593421327914,10.6241500885949,-1.22395338402533));
#97543=CARTESIAN_POINT('Ctrl Pts',(18.797792357215,9.26114234990766,5.31857227275897));
#97544=CARTESIAN_POINT('Ctrl Pts',(19.0361531638009,4.28697136791716,9.76769129949924));
#97545=CARTESIAN_POINT('Ctrl Pts',(19.253957480802,-1.7926669194774,10.3368279771911));
#97546=CARTESIAN_POINT('Ctrl Pts',(19.4526697367228,-6.64906312358094,7.90795031395204));
#97547=CARTESIAN_POINT('Ctrl Pts',(19.6291042447626,-9.53038483805921,3.97628906838568));
#97548=CARTESIAN_POINT('Ctrl Pts',(19.8155522410141,-10.2823637494848,-0.848298560168487));
#97549=CARTESIAN_POINT('Ctrl Pts',(19.9303748982537,-8.74083838503278,-5.4707959614783));
#97550=CARTESIAN_POINT('Ctrl Pts',(20.0764801747596,-5.25087077138079,-8.86716469444201));
#97551=CARTESIAN_POINT('Ctrl Pts',(20.207336615988,-0.594041765760311,-10.2826716766978));
#97552=CARTESIAN_POINT('Ctrl Pts',(20.3455459356972,4.19039095150704,-9.40267864491185));
#97553=CARTESIAN_POINT('Ctrl Pts',(20.4801452049017,8.03490413176417,-6.42622072618347));
#97554=CARTESIAN_POINT('Ctrl Pts',(20.6162967802764,10.0832377386608,-2.02003780110226));
#97555=CARTESIAN_POINT('Ctrl Pts',(20.7516569644152,9.88041700244468,2.83412583686586));
#97556=CARTESIAN_POINT('Ctrl Pts',(20.8872752484866,7.47350957465415,7.04757904292594));
#97557=CARTESIAN_POINT('Ctrl Pts',(21.0226693111701,3.40249785529857,9.69366523532026));
#97558=CARTESIAN_POINT('Ctrl Pts',(21.1581257461099,-1.42584389188091,10.1577350821885));
#97559=CARTESIAN_POINT('Ctrl Pts',(21.2933416880766,-5.92768137593638,8.3913040602114));
#97560=CARTESIAN_POINT('Ctrl Pts',(21.4288360559202,-9.11241563482646,4.6841853921408));
#97561=CARTESIAN_POINT('Ctrl Pts',(21.5186264843219,-9.86491503987726,1.6277742877437));
#97562=CARTESIAN_POINT('Ctrl Pts',(21.5640403001055,-9.87074860163053,0.0039235213980661));
#97563=CARTESIAN_POINT('Ctrl Pts',(1.37078399030106,11.5968559808931,-0.0151246218382906));
#97564=CARTESIAN_POINT('Ctrl Pts',(1.42344639163322,11.5900913133187,1.86791206070984));
#97565=CARTESIAN_POINT('Ctrl Pts',(1.52957558472544,10.7061758009457,5.48262935286527));
#97566=CARTESIAN_POINT('Ctrl Pts',(1.68806725517556,6.97084997875402,9.81349774501377));
#97567=CARTESIAN_POINT('Ctrl Pts',(1.8466683983699,1.6973507383663,11.8916950100086));
#97568=CARTESIAN_POINT('Ctrl Pts',(2.0050573808635,-3.9517229938656,11.3432022055592));
#97569=CARTESIAN_POINT('Ctrl Pts',(2.16329525988592,-8.70792520129272,8.25316135195273));
#97570=CARTESIAN_POINT('Ctrl Pts',(2.32154720540008,-11.5163007375259,3.33435837475925));
#97571=CARTESIAN_POINT('Ctrl Pts',(2.47930854099689,-11.7516016019017,-2.32262613844776));
#97572=CARTESIAN_POINT('Ctrl Pts',(2.63776873621243,-9.36675741608683,-7.45090770551429));
#97573=CARTESIAN_POINT('Ctrl Pts',(2.794221957083,-4.89725641148081,-10.9100368889974));
#97574=CARTESIAN_POINT('Ctrl Pts',(2.95463219424662,0.65612867535488,-11.9299825759692));
#97575=CARTESIAN_POINT('Ctrl Pts',(3.10630295800782,6.05393905269005,-10.2894470217606));
#97576=CARTESIAN_POINT('Ctrl Pts',(3.27540722237603,10.0919898594489,-6.355864787022));
#97577=CARTESIAN_POINT('Ctrl Pts',(3.40813022326932,11.8736472086377,-1.01402480604459));
#97578=CARTESIAN_POINT('Ctrl Pts',(3.62262736521885,11.0043548607243,4.5340281022513));
#97579=CARTESIAN_POINT('Ctrl Pts',(3.82612278073918,7.68498823728818,9.0702913426232));
#97580=CARTESIAN_POINT('Ctrl Pts',(4.05424821818397,2.10412498813912,11.8542631681714));
#97581=CARTESIAN_POINT('Ctrl Pts',(4.303989670121,-4.8628204540389,11.2021430709084));
#97582=CARTESIAN_POINT('Ctrl Pts',(4.57634402750476,-10.5508382917611,6.11230439642354));
#97583=CARTESIAN_POINT('Ctrl Pts',(4.84807252719374,-12.0916100956696,-1.34090444160256));
#97584=CARTESIAN_POINT('Ctrl Pts',(5.11941097117775,-8.92019588881371,-8.24532599345198));
#97585=CARTESIAN_POINT('Ctrl Pts',(5.39023633845774,-2.27430390790531,-11.9119316600466));
#97586=CARTESIAN_POINT('Ctrl Pts',(5.63055313505298,4.39258743413944,-11.0213734801145));
#97587=CARTESIAN_POINT('Ctrl Pts',(5.84050673057507,8.90360029523043,-7.50212221815739));
#97588=CARTESIAN_POINT('Ctrl Pts',(6.02024823233398,11.1846843243296,-3.17590078333041));
#97589=CARTESIAN_POINT('Ctrl Pts',(6.22968662701296,11.544641290149,2.52046272257992));
#97590=CARTESIAN_POINT('Ctrl Pts',(6.46867162670811,8.53143552522916,8.49250563983966));
#97591=CARTESIAN_POINT('Ctrl Pts',(6.73702105051741,1.81498495087946,11.8757023821266));
#97592=CARTESIAN_POINT('Ctrl Pts',(7.00485521835245,-5.57868259143474,10.6134222524762));
#97593=CARTESIAN_POINT('Ctrl Pts',(7.2721709266545,-10.7702618995273,5.21651065947963));
#97594=CARTESIAN_POINT('Ctrl Pts',(7.53896165766792,-11.7402232781411,-2.19213779211188));
#97595=CARTESIAN_POINT('Ctrl Pts',(7.80522410360587,-8.12778048205399,-8.71999414935387));
#97596=CARTESIAN_POINT('Ctrl Pts',(8.02666584019603,-2.4883280973737,-11.2967625293358));
#97597=CARTESIAN_POINT('Ctrl Pts',(8.20355086005244,2.27606964817821,-11.0614057110565));
#97598=CARTESIAN_POINT('Ctrl Pts',(8.38025653867744,6.73185738052523,-9.36966081926595));
#97599=CARTESIAN_POINT('Ctrl Pts',(8.60080147814508,10.8466067486195,-4.76692154743445));
#97600=CARTESIAN_POINT('Ctrl Pts',(8.8649123953267,11.53567362654,2.60451498005851));
#97601=CARTESIAN_POINT('Ctrl Pts',(9.12847741076998,7.71759982857128,8.92050555669179));
#97602=CARTESIAN_POINT('Ctrl Pts',(9.39149464051184,0.910228632703197,11.7373707917927));
#97603=CARTESIAN_POINT('Ctrl Pts',(9.65396108917076,-6.22213213447626,9.96266504826013));
#97604=CARTESIAN_POINT('Ctrl Pts',(9.91587545576831,-10.9058248797927,4.31498350177216));
#97605=CARTESIAN_POINT('Ctrl Pts',(10.1336756686123,-11.2371057762643,-1.77728859852975));
#97606=CARTESIAN_POINT('Ctrl Pts',(10.3076382792719,-9.31065173826634,-6.05446460465524));
#97607=CARTESIAN_POINT('Ctrl Pts',(10.4814156460693,-6.16247232954605,-9.52550747694019));
#97608=CARTESIAN_POINT('Ctrl Pts',(10.6982897832722,-0.46769691448907,-11.6426103959247));
#97609=CARTESIAN_POINT('Ctrl Pts',(10.9291272306577,5.74125850040209,-9.84212207388334));
#97610=CARTESIAN_POINT('Ctrl Pts',(11.1307489689019,9.52008597182504,-5.85814707876185));
#97611=CARTESIAN_POINT('Ctrl Pts',(11.3033199977502,11.0732864155087,-1.42217404507495));
#97612=CARTESIAN_POINT('Ctrl Pts',(11.4564964171182,10.7046015292691,2.73085096518305));
#97613=CARTESIAN_POINT('Ctrl Pts',(11.6286136828385,8.73492349297909,6.92294423096825));
#97614=CARTESIAN_POINT('Ctrl Pts',(11.8004836313932,5.11492430571815,10.0113894279398));
#97615=CARTESIAN_POINT('Ctrl Pts',(11.9911299728693,0.0339235184241942,
11.0965941162476));
#97616=CARTESIAN_POINT('Ctrl Pts',(12.162464967972,-4.52610964494761,10.1183218009339));
#97617=CARTESIAN_POINT('Ctrl Pts',(12.3335535502395,-8.27258546931572,7.34898304513248));
#97618=CARTESIAN_POINT('Ctrl Pts',(12.532870094617,-10.9348781729764,2.61659421510092));
#97619=CARTESIAN_POINT('Ctrl Pts',(12.760250907581,-10.8206047745579,-3.74804922686595));
#97620=CARTESIAN_POINT('Ctrl Pts',(13.0155042484857,-6.46343218839986,-9.42113306769874));
#97621=CARTESIAN_POINT('Ctrl Pts',(13.2702093387032,0.391327358387318,-11.3936597114125));
#97622=CARTESIAN_POINT('Ctrl Pts',(13.524368452853,7.06620025081125,-8.9162445302784));
#97623=CARTESIAN_POINT('Ctrl Pts',(13.777985289017,10.9559308253974,-2.97113304537923));
#97624=CARTESIAN_POINT('Ctrl Pts',(14.031061929482,10.5578777907155,4.10505318065189));
#97625=CARTESIAN_POINT('Ctrl Pts',(14.2836025108293,6.04255217281376,9.55477027287382));
#97626=CARTESIAN_POINT('Ctrl Pts',(14.5076098421657,-0.0453816316895607,
11.0574491674935));
#97627=CARTESIAN_POINT('Ctrl Pts',(14.7032734937542,-5.15662434425682,9.54266445836023));
#97628=CARTESIAN_POINT('Ctrl Pts',(14.8707516580605,-8.61371327624903,6.57092670033119));
#97629=CARTESIAN_POINT('Ctrl Pts',(15.0379975327689,-10.5386613119923,2.44207817038835));
#97630=CARTESIAN_POINT('Ctrl Pts',(15.2050127003932,-10.5974563283306,-2.1053734957677));
#97631=CARTESIAN_POINT('Ctrl Pts',(15.3717983084661,-8.7805015035724,-6.26810077555588));
#97632=CARTESIAN_POINT('Ctrl Pts',(15.524476514162,-5.69774406154741,-9.05856483432574));
#97633=CARTESIAN_POINT('Ctrl Pts',(15.6631094354508,-2.20543986778316,-10.388596236232));
#97634=CARTESIAN_POINT('Ctrl Pts',(15.8293004622731,2.27246813187408,-10.6074440625974));
#97635=CARTESIAN_POINT('Ctrl Pts',(16.0367241073791,7.55354012610783,-8.1968485777852));
#97636=CARTESIAN_POINT('Ctrl Pts',(16.2851349651193,10.9191675552082,-2.09873860741072));
#97637=CARTESIAN_POINT('Ctrl Pts',(16.5330544248483,10.0137352869958,4.7820760466034));
#97638=CARTESIAN_POINT('Ctrl Pts',(16.7804874957598,5.20451469300203,9.77881847117864));
#97639=CARTESIAN_POINT('Ctrl Pts',(17.0000035731033,-0.854928450922944,
10.8020033214215));
#97640=CARTESIAN_POINT('Ctrl Pts',(17.191773677799,-5.73923533968931,8.94868572317326));
#97641=CARTESIAN_POINT('Ctrl Pts',(17.3559407800684,-8.90243151287278,5.79227145828906));
#97642=CARTESIAN_POINT('Ctrl Pts',(17.5199021456526,-10.4825864347342,1.61438667171539));
#97643=CARTESIAN_POINT('Ctrl Pts',(17.6836608334526,-10.2066412558964,-2.83569312779677));
#97644=CARTESIAN_POINT('Ctrl Pts',(17.8472177794713,-8.12643600848449,-6.77504806505468));
#97645=CARTESIAN_POINT('Ctrl Pts',(18.010577720969,-4.61555788199374,-9.50568575518433));
#97646=CARTESIAN_POINT('Ctrl Pts',(18.1737385767459,-0.296033859425129,
-10.5524578266823));
#97647=CARTESIAN_POINT('Ctrl Pts',(18.3367119961153,4.06252364851462,-9.72604612296011));
#97648=CARTESIAN_POINT('Ctrl Pts',(18.5266075658491,8.30676695663606,-6.7667072174541));
#97649=CARTESIAN_POINT('Ctrl Pts',(18.7433599818689,10.8434180575509,-1.2552796992343));
#97650=CARTESIAN_POINT('Ctrl Pts',(18.9866784786254,9.45215064511234,5.42117041791776));
#97651=CARTESIAN_POINT('Ctrl Pts',(19.2298169638985,4.37791280923335,9.9588947253312));
#97652=CARTESIAN_POINT('Ctrl Pts',(19.451862738617,-1.82076892763169,10.5392741564668));
#97653=CARTESIAN_POINT('Ctrl Pts',(19.6544197627791,-6.77058311285345,8.06270985402027));
#97654=CARTESIAN_POINT('Ctrl Pts',(19.8341212662609,-9.7059697419469,4.05833494626081));
#97655=CARTESIAN_POINT('Ctrl Pts',(20.0241128660578,-10.4716758765513,-0.858388280088311));
#97656=CARTESIAN_POINT('Ctrl Pts',(20.1410146593591,-8.90209080241453,-5.56525451310402));
#97657=CARTESIAN_POINT('Ctrl Pts',(20.2897362311998,-5.3492990423135,-9.02216707869922));
#97658=CARTESIAN_POINT('Ctrl Pts',(20.4228963780776,-0.610233353923302,
-10.4627269070358));
#97659=CARTESIAN_POINT('Ctrl Pts',(20.5635028431947,4.2573586450909,-9.56719051602513));
#97660=CARTESIAN_POINT('Ctrl Pts',(20.7003940395719,8.16743907076133,-6.53981610359476));
#97661=CARTESIAN_POINT('Ctrl Pts',(20.8388262275972,10.2500428497637,-2.05952756842641));
#97662=CARTESIAN_POINT('Ctrl Pts',(20.9764120894268,10.043725870545,2.87462578415665));
#97663=CARTESIAN_POINT('Ctrl Pts',(21.1142192325514,7.59769699822165,7.15633992564172));
#97664=CARTESIAN_POINT('Ctrl Pts',(21.2517597955772,3.46196734104235,9.84409234348526));
#97665=CARTESIAN_POINT('Ctrl Pts',(21.3893130359357,-1.44159676850522,10.3156356270535));
#97666=CARTESIAN_POINT('Ctrl Pts',(21.5266025241148,-6.01199771485613,8.52126837621254));
#97667=CARTESIAN_POINT('Ctrl Pts',(21.6640852851583,-9.24412410769275,4.75990666379241));
#97668=CARTESIAN_POINT('Ctrl Pts',(21.7552321039728,-10.0072228406033,1.65687208126127));
#97669=CARTESIAN_POINT('Ctrl Pts',(21.8012598463038,-10.0131352633455,0.0110692926695165));
#100000=UNCERTAINTY_MEASURE_WITH_UNIT(LENGTH_MEASURE(0.01),#100032,
'DISTANCE_ACCURACY_VALUE',
'Maximum model space distance between geometric entities at asserted c
onnectivities');
#100011=UNCERTAINTY_MEASURE_WITH_UNIT(LENGTH_MEASURE(0.01),#100032,
'DISTANCE_ACCURACY_VALUE',
'Maximum model space distance between geometric entities at asserted c
onnectivities');
#100020=(
GEOMETRIC_REPRESENTATION_CONTEXT(3)
GLOBAL_UNCERTAINTY_ASSIGNED_CONTEXT((#100000))
GLOBAL_UNIT_ASSIGNED_CONTEXT((#100032,#100034,#100035))
REPRESENTATION_CONTEXT('','3D')
);
#100031=(
GEOMETRIC_REPRESENTATION_CONTEXT(3)
GLOBAL_UNCERTAINTY_ASSIGNED_CONTEXT((#100011))
GLOBAL_UNIT_ASSIGNED_CONTEXT((#100032,#100034,#100035))
REPRESENTATION_CONTEXT('','3D')
);
#100032=(
LENGTH_UNIT()
NAMED_UNIT(*)
SI_UNIT(.MILLI.,.METRE.)
);
#100034=(
NAMED_UNIT(*)
PLANE_ANGLE_UNIT()
SI_UNIT($,.RADIAN.)
);
#100035=(
NAMED_UNIT(*)
SI_UNIT($,.STERADIAN.)
SOLID_ANGLE_UNIT()
);
#100044=SHAPE_DEFINITION_REPRESENTATION(#100063,#100108);
#100063=PRODUCT_DEFINITION_SHAPE('',$,#100128);
#100108=SHAPE_REPRESENTATION('',(#22152),#100020);
#100119=PRODUCT_DEFINITION_CONTEXT('part definition',#100178,'design');
#100128=PRODUCT_DEFINITION('2026-10-12-11-55-10-897',
'08_Compression_Spring_OD24',#100147,#100119);
#100147=PRODUCT_DEFINITION_FORMATION('',$,#100188);
#100178=APPLICATION_CONTEXT(
'Core Data for Automotive Mechanical Design Process');
#100179=PRODUCT_CONTEXT('part definition',#100178,'mechanical');
#100188=PRODUCT('2026-10-12-11-55-10-897','08_Compression_Spring_OD24',
$,(#100179));
#100203=PRESENTATION_STYLE_ASSIGNMENT((#100209));
#100209=SURFACE_STYLE_USAGE(.BOTH.,#100215);
#100215=SURFACE_SIDE_STYLE('',(#100221));
#100221=SURFACE_STYLE_FILL_AREA(#100227);
#100227=FILL_AREA_STYLE('Opaque(122,133,145)',(#100233));
#100233=FILL_AREA_STYLE_COLOUR('Opaque(122,133,145)',#100239);
#100239=COLOUR_RGB('Opaque(122,133,145)',0.47843137254902,0.52156862745098,
0.568627450980392);
ENDSEC;
END-ISO-10303-21;
